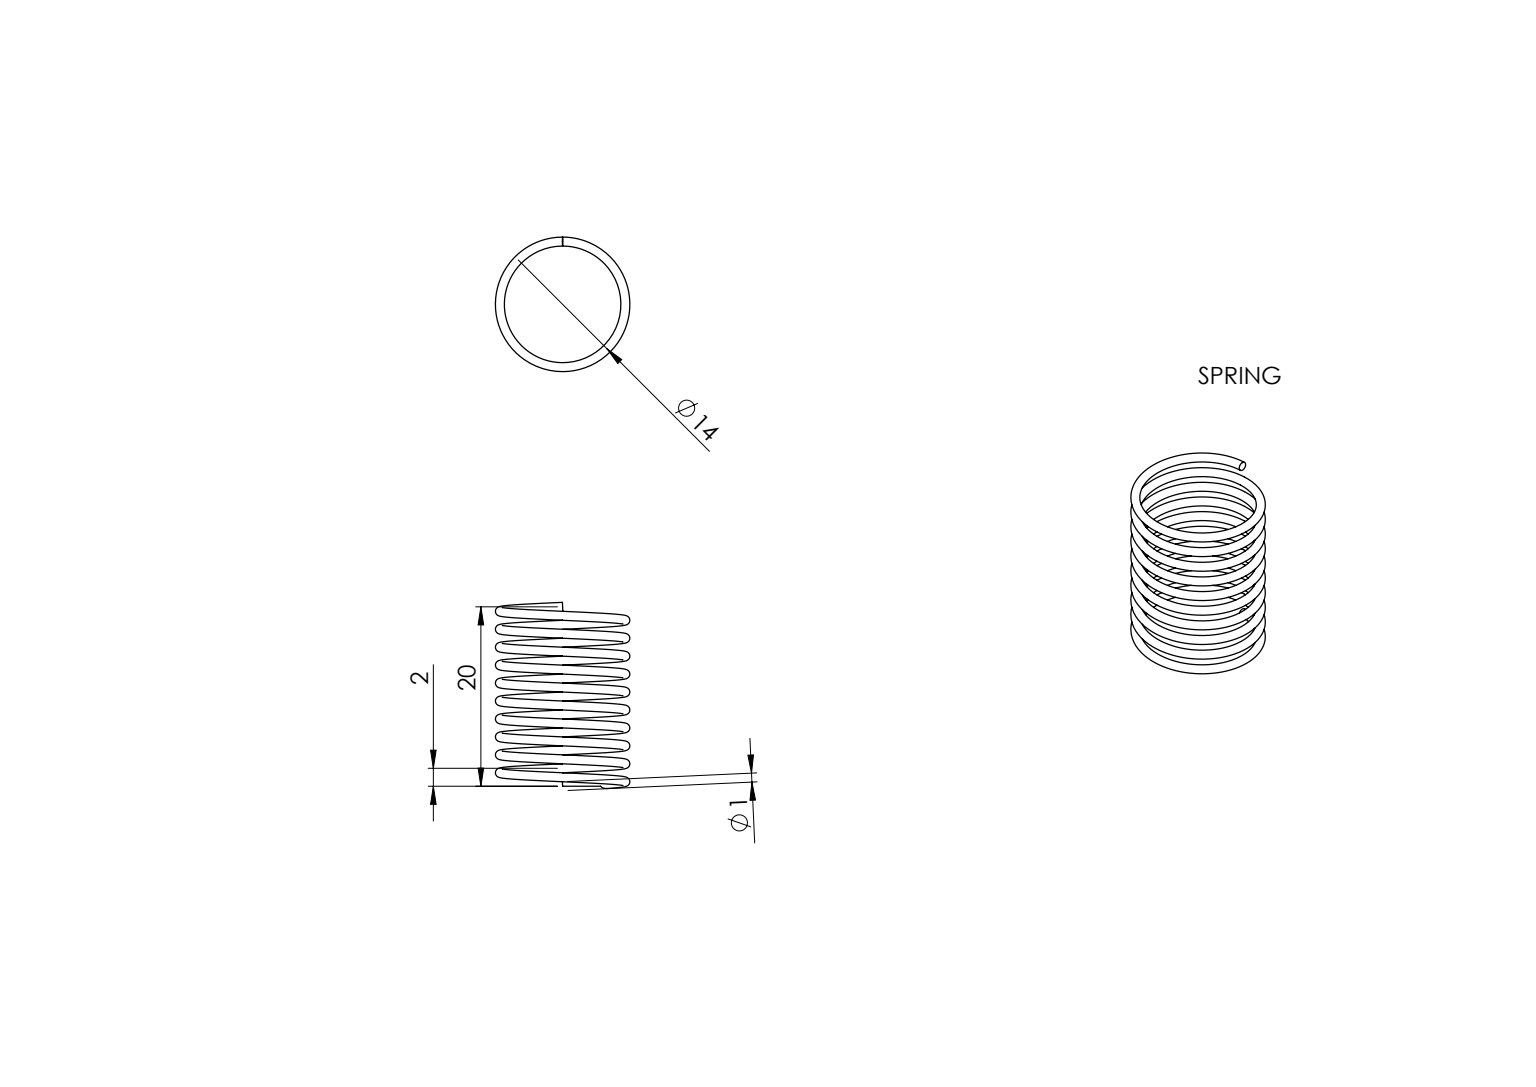
ISO-10303-21;
HEADER;
FILE_DESCRIPTION (('STEP AP214'),
    '1' );
FILE_NAME ('spring.step',
    '2026-10-31T03:44:21',
    ( '' ),
    ( '' ),
    'SwSTEP 2.0',
    'SolidWorks 2026',
    '' );
FILE_SCHEMA (( 'AUTOMOTIVE_DESIGN' ));
ENDSEC;

DATA;
#1=CARTESIAN_POINT ( 'NONE',  ( 55.94051828345054389, 59.20051614449765509, 4.345558710429044957 ) ) ;
#5=CARTESIAN_POINT ( 'NONE',  ( 55.08986747509849380, 53.20051614449766220, 3.727524721679155384 ) ) ;
#7=CARTESIAN_POINT ( 'NONE',  ( 55.11794222512601493, 60.19948385550240744, 3.688883143319541702 ) ) ;
#9=CARTESIAN_POINT ( 'NONE',  ( 44.05948171654949874, 50.79948385550238754, 4.345558710429105354 ) ) ;
#11=CARTESIAN_POINT ( 'NONE',  ( 43.18075615816994173, 53.80051614449766362, 4.924951120819380357 ) ) ;
#23=CARTESIAN_POINT ( 'NONE',  ( 50.02271294988512551, 62.49948385550240459, 7.000000000000000888 ) ) ;
#29=CARTESIAN_POINT ( 'NONE',  ( 47.74827507625478518, 56.59948385550238470, 7.007379884777227730 ) ) ;
#32=CARTESIAN_POINT ( 'NONE',  ( 54.68390685589033495, 51.69948385550241454, -6.485486291978119766 ) ) ;
#34=CARTESIAN_POINT ( 'NONE',  ( 56.65037692655921120, 57.10051614449766078, 2.184720259617097593 ) ) ;
#39=AXIS2_PLACEMENT_3D ( 'NONE', #18626, #14180, #9573 ) ;
#51=CARTESIAN_POINT ( 'NONE',  ( 44.28664221472220675, 59.09948385550240602, -1.832500667257165317 ) ) ;
#56=CARTESIAN_POINT ( 'NONE',  ( 49.97728705011495265, 51.50051614449765935, 8.000000000000001776 ) ) ;
#57=CARTESIAN_POINT ( 'NONE',  ( 53.54508667620424234, 58.70051614449765509, -4.840751629271188961 ) ) ;
#69=CARTESIAN_POINT ( 'NONE',  ( 44.05948171654949874, 62.79948385550241596, 4.345558710429105354 ) ) ;
#70=DIRECTION ( 'NONE',  ( -0.9989677110047504582, -0.04542589977017007230, 1.386346192018204258E-14 ) ) ;
#77=CARTESIAN_POINT ( 'NONE',  ( 58.41169779390614281, 45.99948385550240459, -0.02388180880523160798 ) ) ;
#80=CARTESIAN_POINT ( 'NONE',  ( 50.02271294988512551, 56.49948385550240459, 7.000000000000000888 ) ) ;
#84=CARTESIAN_POINT ( 'NONE',  ( 43.34962307344078880, 54.10051614449766788, -2.184720259617096705 ) ) ;
#92=CARTESIAN_POINT ( 'NONE',  ( 43.20883090819745576, 64.79948385550240175, 4.963592699179006473 ) ) ;
#97=CARTESIAN_POINT ( 'NONE',  ( 42.63976443033212149, 62.00051614449765225, -0.02388180880514948964 ) ) ;
#103=CARTESIAN_POINT ( 'NONE',  ( 55.11794222512599362, 56.80051614449764941, -3.688883143319583446 ) ) ;
#106=CARTESIAN_POINT ( 'NONE',  ( 49.97728705011488870, 55.49948385550241170, -6.000000000000000888 ) ) ;
#108=CARTESIAN_POINT ( 'NONE',  ( 43.20883090819742023, 54.20051614449766220, -4.963592699178938972 ) ) ;
#119=CARTESIAN_POINT ( 'NONE',  ( 43.33558569842703179, 65.09948385550239891, -2.141517661632099223 ) ) ;
#123=CARTESIAN_POINT ( 'NONE',  ( 44.03140696652192787, 61.19948385550239323, -4.306917132069425058 ) ) ;
#125=CARTESIAN_POINT ( 'NONE',  ( 43.18075615816989199, 53.19948385550240744, -4.924951120819313743 ) ) ;
#127=CARTESIAN_POINT ( 'NONE',  ( 45.90387839640208512, 54.30051614449765651, -5.676469297603124353 ) ) ;
#136=CARTESIAN_POINT ( 'NONE',  ( 55.96859303347804371, 62.19948385550240744, 4.306917132069425946 ) ) ;
#137=PLANE ( 'NONE',  #4619 ) ;
#141=CARTESIAN_POINT ( 'NONE',  ( 51.97223112728254790, 58.39948385550241028, 5.992620115222778487 ) ) ;
#144=CARTESIAN_POINT ( 'NONE',  ( 45.31609314410960820, 54.30051614449765651, -6.485486291978072693 ) ) ;
#146=CARTESIAN_POINT ( 'NONE',  ( 48.07319477248762496, 54.40051614449765793, -6.007379884777208190 ) ) ;
#155=CARTESIAN_POINT ( 'NONE',  ( 54.09612160359786515, 63.69948385550240744, -5.676469297603166098 ) ) ;
#165=CARTESIAN_POINT ( 'NONE',  ( 47.37792948025162332, 47.39948385550241028, -7.992620115222770494 ) ) ;
#169=CARTESIAN_POINT ( 'NONE',  ( 55.94051828345050836, 55.79948385550238044, -4.345558710429104465 ) ) ;
#172=CARTESIAN_POINT ( 'NONE',  ( 56.66441430157294690, 56.90051614449766504, -2.141517661632166281 ) ) ;
#185=CARTESIAN_POINT ( 'NONE',  ( 57.61547081786812896, 64.09948385550239891, 2.450534656007040901 ) ) ;
#190=CARTESIAN_POINT ( 'NONE',  ( 44.05948171654945611, 58.20051614449764799, -4.345558710429044069 ) ) ;
#196=CARTESIAN_POINT ( 'NONE',  ( 50.02271294988506156, 56.50051614449767357, -6.000000000000000888 ) ) ;
#200=CARTESIAN_POINT ( 'NONE',  ( 46.49166364869460466, 56.69948385550240744, 4.867452303228209765 ) ) ;
#202=CARTESIAN_POINT ( 'NONE',  ( 47.37792948025170858, 53.60051614449765367, 7.992620115222797139 ) ) ;
#212=CARTESIAN_POINT ( 'NONE',  ( 55.96859303347805081, 62.19948385550241454, 4.306917132069425058 ) ) ;
#216=CARTESIAN_POINT ( 'NONE',  ( 56.65037692655918988, 57.89948385550240317, -2.184720259617163762 ) ) ;
#219=CARTESIAN_POINT ( 'NONE',  ( 52.57664461997811856, 55.59948385550240602, -8.007379884777229506 ) ) ;
#221=CARTESIAN_POINT ( 'NONE',  ( 47.74827507625469281, 54.40051614449766504, -7.007379884777203749 ) ) ;
#229=CARTESIAN_POINT ( 'NONE',  ( 57.36023556966787851, 49.00051614449764514, 0.02388180880515038476 ) ) ;
#230=CARTESIAN_POINT ( 'NONE',  ( 50.02271294988512551, 62.49948385550240459, 7.000000000000000888 ) ) ;
#235=CARTESIAN_POINT ( 'NONE',  ( 44.91013252490152752, 56.79948385550240175, 3.727524721679198461 ) ) ;
#239=CARTESIAN_POINT ( 'NONE',  ( 49.97728705011495265, 55.50051614449766646, 8.000000000000001776 ) ) ;
#240=CARTESIAN_POINT ( 'NONE',  ( 53.50833635130544508, 57.30051614449767072, 4.867452303228181343 ) ) ;
#254=CARTESIAN_POINT ( 'NONE',  ( 55.94051828345050836, 51.79948385550240175, -4.345558710429103577 ) ) ;
#259=CARTESIAN_POINT ( 'NONE',  ( 56.81924384183011512, 48.19948385550240744, 4.924951120819313743 ) ) ;
#261=CARTESIAN_POINT ( 'NONE',  ( 52.25172492374522903, 57.59948385550241312, -7.007379884777225953 ) ) ;
#263=( GEOMETRIC_REPRESENTATION_CONTEXT ( 3 ) GLOBAL_UNCERTAINTY_ASSIGNED_CONTEXT ( ( #6357 ) ) GLOBAL_UNIT_ASSIGNED_CONTEXT ( ( #5384, #15479, #3919 ) ) REPRESENTATION_CONTEXT ( 'NONE', 'WORKASPACE' ) );
#264=CARTESIAN_POINT ( 'NONE',  ( 54.09612160359792199, 57.30051614449765651, 5.676469297603124353 ) ) ;
#276=CARTESIAN_POINT ( 'NONE',  ( 55.94051828345050836, 45.79948385550240886, -4.345558710429104465 ) ) ;
#283=CARTESIAN_POINT ( 'NONE',  ( 43.33558569842706021, 59.90051614449766504, 2.141517661632167169 ) ) ;
#290=CARTESIAN_POINT ( 'NONE',  ( 44.30067958973594955, 54.10051614449766078, -1.875703265242155693 ) ) ;
#296=CARTESIAN_POINT ( 'NONE',  ( 48.02776887271745210, 61.39948385550240317, -5.992620115222778487 ) ) ;
#299=CARTESIAN_POINT ( 'NONE',  ( 47.37792948025170858, 55.60051614449765367, 7.992620115222797139 ) ) ;
#321=CARTESIAN_POINT ( 'NONE',  ( 49.97728705011488159, 55.49948385550240459, -7.000000000000000888 ) ) ;
#323=CARTESIAN_POINT ( 'NONE',  ( 47.37792948025162332, 57.39948385550241028, -7.992620115222770494 ) ) ;
#324=CARTESIAN_POINT ( 'NONE',  ( 47.74827507625469281, 52.40051614449763662, -7.007379884777203749 ) ) ;
#334=CARTESIAN_POINT ( 'NONE',  ( 54.13287192849676188, 64.29948385550241596, 5.649768623646098220 ) ) ;
#341=CARTESIAN_POINT ( 'NONE',  ( 46.49166364869460466, 60.69948385550240033, 4.867452303228209765 ) ) ;
#345=CARTESIAN_POINT ( 'NONE',  ( 43.18075615816994173, 57.80051614449766362, 4.924951120819380357 ) ) ;
#346=CARTESIAN_POINT ( 'NONE',  ( 49.97728705011494554, 57.50051614449766646, 6.000000000000000888 ) ) ;
#360=CARTESIAN_POINT ( 'NONE',  ( 52.25172492374522903, 49.59948385550240602, -7.007379884777227730 ) ) ;
#366=CARTESIAN_POINT ( 'NONE',  ( 54.72065718078924590, 46.29948385550240886, 6.458785618021043895 ) ) ;
#370=CARTESIAN_POINT ( 'NONE',  ( 56.66441430157296821, 64.09948385550239891, 2.141517661632100111 ) ) ;
#373=CARTESIAN_POINT ( 'NONE',  ( 47.74827507625469281, 56.40051614449766504, -7.007379884777203749 ) ) ;
#375=CARTESIAN_POINT ( 'NONE',  ( 52.25172492374522903, 53.59948385550241312, -7.007379884777225953 ) ) ;
#381=CARTESIAN_POINT ( 'NONE',  ( 56.66441430157296821, 54.09948385550240602, 2.141517661632100111 ) ) ;
#387=CARTESIAN_POINT ( 'NONE',  ( 47.70284917648459810, 59.60051614449765367, 6.992620115222797139 ) ) ;
#391=CARTESIAN_POINT ( 'NONE',  ( 46.45491332379576477, 55.70051614449766220, 4.840751629271188961 ) ) ;
#394=CARTESIAN_POINT ( 'NONE',  ( 53.50833635130540955, 61.69948385550240744, -4.867452303228209765 ) ) ;
#396=CARTESIAN_POINT ( 'NONE',  ( 47.37792948025170858, 57.60051614449765367, 7.992620115222797139 ) ) ;
#407=CARTESIAN_POINT ( 'NONE',  ( 47.70284917648453415, 65.39948385550239607, -6.992620115222774047 ) ) ;
#413=CARTESIAN_POINT ( 'NONE',  ( 56.66441430157296821, 62.09948385550239891, 2.141517661632100111 ) ) ;
#415=CARTESIAN_POINT ( 'NONE',  ( 54.72065718078924590, 62.29948385550241596, 6.458785618021043895 ) ) ;
#416=CARTESIAN_POINT ( 'NONE',  ( 57.36023556966787851, 63.00051614449767357, 0.02388180880515038476 ) ) ;
#425=CARTESIAN_POINT ( 'NONE',  ( 44.03140696652198471, 45.80051614449766362, 4.306917132069485454 ) ) ;
#426=CARTESIAN_POINT ( 'NONE',  ( 55.96859303347804371, 64.19948385550239323, 4.306917132069425946 ) ) ;
#431=CARTESIAN_POINT ( 'NONE',  ( 43.69122665457040000, 64.99948385550240459, 0.02388180880521036456 ) ) ;
#433=CARTESIAN_POINT ( 'NONE',  ( 42.38452918213190657, 61.90051614449766504, 2.450534656007115508 ) ) ;
#434=CARTESIAN_POINT ( 'NONE',  ( 44.88205777487401349, 57.80051614449766362, 3.688883143319584779 ) ) ;
#446=CARTESIAN_POINT ( 'NONE',  ( 43.34962307344081012, 54.89948385550240317, 2.184720259617164650 ) ) ;
#451=CARTESIAN_POINT ( 'NONE',  ( 47.42335538002188144, 52.59948385550240602, 8.007379884777233059 ) ) ;
#454=CARTESIAN_POINT ( 'NONE',  ( 56.66441430157296821, 62.09948385550239891, 2.141517661632100111 ) ) ;
#456=CARTESIAN_POINT ( 'NONE',  ( 47.70284917648459100, 63.60051614449766078, 6.992620115222796251 ) ) ;
#458=CARTESIAN_POINT ( 'NONE',  ( 49.97728705011488159, 57.49948385550241170, -7.000000000000000888 ) ) ;
#466=CARTESIAN_POINT ( 'NONE',  ( 54.13287192849676188, 52.29948385550240886, 5.649768623646098220 ) ) ;
#472=CARTESIAN_POINT ( 'NONE',  ( 42.63976443033212149, 64.00051614449765225, -0.02388180880514948964 ) ) ;
#478=CARTESIAN_POINT ( 'NONE',  ( 55.71335778527780036, 58.90051614449766504, -1.832500667257213056 ) ) ;
#483=CARTESIAN_POINT ( 'NONE',  ( 52.57664461997821093, 57.40051614449767214, 8.007379884777206414 ) ) ;
#493=LINE ( 'NONE', #12738, #1897 ) ;
#496=UNCERTAINTY_MEASURE_WITH_UNIT (LENGTH_MEASURE( 1.000000000000000082E-05 ), #5087, 'distance_accuracy_value', 'NONE');
#501=CARTESIAN_POINT ( 'NONE',  ( 55.94051828345050836, 63.79948385550240886, -4.345558710429104465 ) ) ;
#503=CARTESIAN_POINT ( 'NONE',  ( 42.38452918213188525, 63.09948385550240602, -2.450534656007040013 ) ) ;
#505=CARTESIAN_POINT ( 'NONE',  ( 42.63976443033212860, 58.00051614449765225, -0.02388180880514948964 ) ) ;
#511=CARTESIAN_POINT ( 'NONE',  ( 45.86712807150323812, 63.29948385550240886, -5.649768623646098220 ) ) ;
#518=CARTESIAN_POINT ( 'NONE',  ( 51.97223112728254790, 62.39948385550240317, 5.992620115222778487 ) ) ;
#521=CARTESIAN_POINT ( 'NONE',  ( 41.58830220609386430, 62.00051614449766646, -0.02388180880514929535 ) ) ;
#523=CARTESIAN_POINT ( 'NONE',  ( 44.88205777487401349, 61.80051614449766362, 3.688883143319584779 ) ) ;
#539=CARTESIAN_POINT ( 'NONE',  ( 54.13287192849676188, 52.29948385550240886, 5.649768623646098220 ) ) ;
#544=AXIS2_PLACEMENT_3D ( 'NONE', #1693, #7660, #14721 ) ;
#545=CARTESIAN_POINT ( 'NONE',  ( 58.41169779390614281, 49.99948385550240459, -0.02388180880523160798 ) ) ;
#548=CARTESIAN_POINT ( 'NONE',  ( 52.29715082351547295, 64.39948385550239607, 6.992620115222774047 ) ) ;
#552=CARTESIAN_POINT ( 'NONE',  ( 44.05948171654945611, 60.20051614449764799, -4.345558710429044069 ) ) ;
#554=CARTESIAN_POINT ( 'NONE',  ( 50.02271294988512551, 60.49948385550240459, 7.000000000000000888 ) ) ;
#561=CARTESIAN_POINT ( 'NONE',  ( 56.65037692655918988, 51.89948385550241028, -2.184720259617163762 ) ) ;
#570=CARTESIAN_POINT ( 'NONE',  ( 45.86712807150323812, 47.29948385550240886, -5.649768623646098220 ) ) ;
#572=CARTESIAN_POINT ( 'NONE',  ( 46.49166364869456913, 62.30051614449766362, -4.867452303228181343 ) ) ;
#578=CARTESIAN_POINT ( 'NONE',  ( 52.57664461997821093, 61.40051614449765793, 8.007379884777206414 ) ) ;
#596=CARTESIAN_POINT ( 'NONE',  ( 55.08986747509847248, 45.79948385550240886, -3.727524721679197572 ) ) ;
#598=CARTESIAN_POINT ( 'NONE',  ( 41.58830220609386430, 58.99948385550239749, 0.02388180880523263147 ) ) ;
#600=CARTESIAN_POINT ( 'NONE',  ( 47.74827507625469281, 62.40051614449766504, -7.007379884777203749 ) ) ;
#609=CARTESIAN_POINT ( 'NONE',  ( 42.63976443033212149, 48.00051614449766646, -0.02388180880514948964 ) ) ;
#616=CARTESIAN_POINT ( 'NONE',  ( 43.69122665457040000, 60.99948385550241170, 0.02388180880521036456 ) ) ;
#618=CARTESIAN_POINT ( 'NONE',  ( 54.09612160359786515, 47.69948385550240744, -5.676469297603166098 ) ) ;
#621=CARTESIAN_POINT ( 'NONE',  ( 56.81924384183006538, 56.80051614449764941, -4.924951120819380357 ) ) ;
#622=CARTESIAN_POINT ( 'NONE',  ( 44.88205777487401349, 59.80051614449766362, 3.688883143319584779 ) ) ;
#626=ORIENTED_EDGE ( 'NONE', *, *, #1141, .T. ) ;
#636=CARTESIAN_POINT ( 'NONE',  ( 57.36023556966787851, 53.99948385550239749, -0.02388180880522424582 ) ) ;
#641=CARTESIAN_POINT ( 'NONE',  ( 56.79116909180255135, 49.79948385550240175, -4.963592699179005585 ) ) ;
#645=CARTESIAN_POINT ( 'NONE',  ( 44.88205777487398507, 47.19948385550240744, -3.688883143319540814 ) ) ;
#650=CARTESIAN_POINT ( 'NONE',  ( 43.33558569842706021, 57.90051614449766504, 2.141517661632167169 ) ) ;
#654=CARTESIAN_POINT ( 'NONE',  ( 57.36023556966787851, 55.99948385550239038, -0.02388180880522424582 ) ) ;
#663=CARTESIAN_POINT ( 'NONE',  ( 56.65037692655918988, 53.89948385550240317, -2.184720259617163762 ) ) ;
#672=CARTESIAN_POINT ( 'NONE',  ( 43.34962307344078880, 64.10051614449766078, -2.184720259617096705 ) ) ;
#676=CARTESIAN_POINT ( 'NONE',  ( 46.45491332379576477, 61.70051614449766220, 4.840751629271188961 ) ) ;
#682=CARTESIAN_POINT ( 'NONE',  ( 49.97728705011495265, 59.50051614449765935, 8.000000000000001776 ) ) ;
#700=CARTESIAN_POINT ( 'NONE',  ( 46.49166364869460466, 46.69948385550240744, 4.867452303228209765 ) ) ;
#702=CARTESIAN_POINT ( 'NONE',  ( 42.39856655714566358, 60.89948385550241028, 2.493737253992119207 ) ) ;
#703=CARTESIAN_POINT ( 'NONE',  ( 45.86712807150329496, 63.70051614449766220, 5.649768623646139964 ) ) ;
#712=CARTESIAN_POINT ( 'NONE',  ( 44.03140696652198471, 53.80051614449766362, 4.306917132069485454 ) ) ;
#722=CARTESIAN_POINT ( 'NONE',  ( 47.42335538002180328, 58.40051614449765793, -8.007379884777206414 ) ) ;
#723=CARTESIAN_POINT ( 'NONE',  ( 44.30067958973594955, 62.10051614449765367, -1.875703265242155693 ) ) ;
#734=CARTESIAN_POINT ( 'NONE',  ( 43.34962307344081012, 60.89948385550241028, 2.184720259617164650 ) ) ;
#738=CARTESIAN_POINT ( 'NONE',  ( 47.42335538002188144, 54.59948385550240602, 8.007379884777233059 ) ) ;
#740=CARTESIAN_POINT ( 'NONE',  ( 44.03140696652192787, 65.19948385550240744, -4.306917132069425058 ) ) ;
#743=CARTESIAN_POINT ( 'NONE',  ( 56.65037692655921120, 61.10051614449766078, 2.184720259617097593 ) ) ;
#744=CARTESIAN_POINT ( 'NONE',  ( 44.28664221472220675, 65.09948385550239891, -1.832500667257165317 ) ) ;
#745=CARTESIAN_POINT ( 'NONE',  ( 43.34962307344081012, 58.89948385550241028, 2.184720259617164650 ) ) ;
#754=CARTESIAN_POINT ( 'NONE',  ( 45.90387839640214196, 58.69948385550240033, 5.676469297603166098 ) ) ;
#764=CARTESIAN_POINT ( 'NONE',  ( 55.96859303347804371, 46.19948385550238612, 4.306917132069425946 ) ) ;
#767=CARTESIAN_POINT ( 'NONE',  ( 53.54508667620424234, 58.70051614449765509, -4.840751629271188961 ) ) ;
#780=ADVANCED_BREP_SHAPE_REPRESENTATION ( '', ( #2030, #10359 ), #6832 ) ;
#796=CARTESIAN_POINT ( 'NONE',  ( 54.13287192849676188, 64.29948385550241596, 5.649768623646098220 ) ) ;
#798=CARTESIAN_POINT ( 'NONE',  ( 57.60143344285433642, 63.89948385550240317, -2.493737253992118319 ) ) ;
#799=CARTESIAN_POINT ( 'NONE',  ( 52.29715082351538769, 62.60051614449766078, -6.992620115222796251 ) ) ;
#806=CARTESIAN_POINT ( 'NONE',  ( 55.94051828345054389, 55.20051614449766220, 4.345558710429044957 ) ) ;
#815=CARTESIAN_POINT ( 'NONE',  ( 47.74827507625478518, 48.59948385550239180, 7.007379884777227730 ) ) ;
#817=CARTESIAN_POINT ( 'NONE',  ( 49.97728705011486738, 47.49948385550240459, -8.000000000000001776 ) ) ;
#820=CARTESIAN_POINT ( 'NONE',  ( 55.69932041026405045, 61.10051614449766788, 1.875703265242156359 ) ) ;
#830=EDGE_LOOP ( 'NONE', ( #4840, #13776, #3319, #7867, #626, #1665 ) ) ;
#832=CARTESIAN_POINT ( 'NONE',  ( 56.65037692655918988, 57.89948385550240317, -2.184720259617163762 ) ) ;
#836=CARTESIAN_POINT ( 'NONE',  ( 45.27934281921075410, 55.29948385550240175, -6.458785618021043895 ) ) ;
#838=CARTESIAN_POINT ( 'NONE',  ( 51.92680522751233951, 51.59948385550240602, -6.007379884777223289 ) ) ;
#841=CARTESIAN_POINT ( 'NONE',  ( 44.03140696652198471, 61.80051614449767072, 4.306917132069485454 ) ) ;
#842=CARTESIAN_POINT ( 'NONE',  ( 49.97728705011488870, 65.49948385550240459, -6.000000000000000888 ) ) ;
#844=CARTESIAN_POINT ( 'NONE',  ( 56.66441430157296821, 60.09948385550240602, 2.141517661632100111 ) ) ;
#852=CARTESIAN_POINT ( 'NONE',  ( 43.33558569842703179, 61.09948385550240602, -2.141517661632099223 ) ) ;
#863=CARTESIAN_POINT ( 'NONE',  ( 46.45491332379576477, 59.70051614449766220, 4.840751629271188961 ) ) ;
#888=CARTESIAN_POINT ( 'NONE',  ( 44.88205777487398507, 51.19948385550240744, -3.688883143319540814 ) ) ;
#890=CARTESIAN_POINT ( 'NONE',  ( 44.03140696652192787, 47.19948385550240744, -4.306917132069425058 ) ) ;
#891=CARTESIAN_POINT ( 'NONE',  ( 41.58830220609386430, 46.00051614449764514, -0.02388180880514929535 ) ) ;
#902=CARTESIAN_POINT ( 'NONE',  ( 43.34962307344078880, 52.10051614449766078, -2.184720259617096705 ) ) ;
#913=CARTESIAN_POINT ( 'NONE',  ( 44.03140696652192787, 49.19948385550240033, -4.306917132069425058 ) ) ;
#915=CARTESIAN_POINT ( 'NONE',  ( 56.81924384183011512, 50.19948385550241454, 4.924951120819313743 ) ) ;
#917=CARTESIAN_POINT ( 'NONE',  ( 49.97728705011494554, 59.50051614449765935, 6.000000000000000888 ) ) ;
#919=PLANE ( 'NONE',  #15371 ) ;
#931=CARTESIAN_POINT ( 'NONE',  ( 55.94051828345050836, 55.79948385550239465, -4.345558710429103577 ) ) ;
#937=CARTESIAN_POINT ( 'NONE',  ( 54.72065718078924590, 60.29948385550240175, 6.458785618021043895 ) ) ;
#939=CARTESIAN_POINT ( 'NONE',  ( 55.08986747509847248, 49.79948385550240175, -3.727524721679197572 ) ) ;
#943=CARTESIAN_POINT ( 'NONE',  ( 57.61547081786810764, 46.90051614449766504, -2.450534656007114176 ) ) ;
#945=CARTESIAN_POINT ( 'NONE',  ( 55.71335778527780036, 44.90051614449765793, -1.832500667257213056 ) ) ;
#954=CARTESIAN_POINT ( 'NONE',  ( 54.13287192849676188, 60.29948385550240886, 5.649768623646098220 ) ) ;
#966=CARTESIAN_POINT ( 'NONE',  ( 56.66441430157296821, 54.09948385550240602, 2.141517661632100111 ) ) ;
#968=CARTESIAN_POINT ( 'NONE',  ( 44.05948171654945611, 46.20051614449766930, -4.345558710429044069 ) ) ;
#991=CARTESIAN_POINT ( 'NONE',  ( 50.02271294988506156, 44.50051614449765935, -6.000000000000000888 ) ) ;
#995=CARTESIAN_POINT ( 'NONE',  ( 44.91013252490152752, 52.79948385550240175, 3.727524721679198461 ) ) ;
#997=CARTESIAN_POINT ( 'NONE',  ( 43.18075615816989199, 63.19948385550240744, -4.924951120819313743 ) ) ;
#998=CARTESIAN_POINT ( 'NONE',  ( 56.81924384183006538, 48.80051614449767072, -4.924951120819380357 ) ) ;
#1009=CARTESIAN_POINT ( 'NONE',  ( 50.02271294988505446, 54.50051614449765935, -7.000000000000000888 ) ) ;
#1018=CARTESIAN_POINT ( 'NONE',  ( 57.36023556966787851, 49.99948385550238328, -0.02388180880522424582 ) ) ;
#1020=CARTESIAN_POINT ( 'NONE',  ( 49.97728705011495265, 63.50051614449765935, 8.000000000000001776 ) ) ;
#1022=CARTESIAN_POINT ( 'NONE',  ( 47.74827507625469281, 48.40051614449764372, -7.007379884777203749 ) ) ;
#1035=CARTESIAN_POINT ( 'NONE',  ( 44.03140696652193498, 57.19948385550239323, -4.306917132069424170 ) ) ;
#1040=CARTESIAN_POINT ( 'NONE',  ( 47.37792948025162332, 59.39948385550240317, -7.992620115222770494 ) ) ;
#1042=CARTESIAN_POINT ( 'NONE',  ( 49.97728705011488870, 51.49948385550240459, -6.000000000000000888 ) ) ;
#1045=CARTESIAN_POINT ( 'NONE',  ( 56.81924384183006538, 44.80051614449766362, -4.924951120819380357 ) ) ;
#1046=CARTESIAN_POINT ( 'NONE',  ( 43.69122665457040000, 48.00051614449766646, -0.02388180880515696977 ) ) ;
#1053=CARTESIAN_POINT ( 'NONE',  ( 42.63976443033212860, 56.99948385550241170, 0.02388180880522514787 ) ) ;
#1061=CARTESIAN_POINT ( 'NONE',  ( 56.65037692655918988, 49.89948385550240317, -2.184720259617163762 ) ) ;
#1063=CARTESIAN_POINT ( 'NONE',  ( 57.36023556966787851, 47.00051614449764514, 0.02388180880515038476 ) ) ;
#1085=CARTESIAN_POINT ( 'NONE',  ( 44.91013252490150620, 48.20051614449766930, -3.727524721679154940 ) ) ;
#1089=CARTESIAN_POINT ( 'NONE',  ( 43.69122665457040000, 52.99948385550241170, 0.02388180880521036456 ) ) ;
#1091=CARTESIAN_POINT ( 'NONE',  ( 56.66441430157296821, 46.09948385550240602, 2.141517661632100111 ) ) ;
#1092=CARTESIAN_POINT ( 'NONE',  ( 41.58830220609386430, 48.00051614449766646, -0.02388180880514929535 ) ) ;
#1100=CARTESIAN_POINT ( 'NONE',  ( 49.97728705011495265, 51.50051614449765935, 7.000000000000000888 ) ) ;
#1108=CARTESIAN_POINT ( 'NONE',  ( 55.94051828345050836, 51.79948385550240175, -4.345558710429104465 ) ) ;
#1110=CARTESIAN_POINT ( 'NONE',  ( 45.31609314410967926, 46.69948385550240744, 6.485486291978119766 ) ) ;
#1112=CARTESIAN_POINT ( 'NONE',  ( 45.90387839640208512, 46.30051614449766362, -5.676469297603124353 ) ) ;
#1127=CARTESIAN_POINT ( 'NONE',  ( 57.61547081786812896, 58.09948385550241312, 2.450534656007040901 ) ) ;
#1131=CARTESIAN_POINT ( 'NONE',  ( 55.71335778527780747, 48.09948385550240602, 1.832500667257165983 ) ) ;
#1135=CARTESIAN_POINT ( 'NONE',  ( 43.20883090819742023, 50.20051614449766220, -4.963592699178938972 ) ) ;
#1136=CARTESIAN_POINT ( 'NONE',  ( 48.07319477248762496, 50.40051614449766504, -6.007379884777208190 ) ) ;
#1141=EDGE_CURVE ( 'NONE', #2212, #18471, #2132, .T. ) ;
#1146=CARTESIAN_POINT ( 'NONE',  ( 43.34962307344081012, 60.89948385550241028, 2.184720259617164650 ) ) ;
#1156=CARTESIAN_POINT ( 'NONE',  ( 57.36023556966787851, 51.99948385550238328, -0.02388180880522424582 ) ) ;
#1160=CARTESIAN_POINT ( 'NONE',  ( 54.13287192849671214, 50.70051614449766220, -5.649768623646139964 ) ) ;
#1183=CARTESIAN_POINT ( 'NONE',  ( 44.88205777487401349, 49.80051614449765651, 3.688883143319584779 ) ) ;
#1187=CARTESIAN_POINT ( 'NONE',  ( 53.54508667620428497, 48.29948385550240175, 4.840751629271157874 ) ) ;
#1190=CARTESIAN_POINT ( 'NONE',  ( 52.62207051974839089, 64.39948385550239607, 7.992620115222770494 ) ) ;
#1191=CARTESIAN_POINT ( 'NONE',  ( 47.74827507625469281, 64.40051614449765793, -7.007379884777203749 ) ) ;
#1205=CARTESIAN_POINT ( 'NONE',  ( 43.34962307344081012, 50.89948385550241028, 2.184720259617164650 ) ) ;
#1207=CARTESIAN_POINT ( 'NONE',  ( 54.72065718078924590, 46.29948385550240886, 6.458785618021043895 ) ) ;
#1209=CARTESIAN_POINT ( 'NONE',  ( 55.96859303347802239, 46.80051614449767072, -4.306917132069484566 ) ) ;
#1225=CARTESIAN_POINT ( 'NONE',  ( 56.79116909180255135, 61.79948385550240175, -4.963592699179005585 ) ) ;
#1228=CARTESIAN_POINT ( 'NONE',  ( 48.02776887271745210, 51.39948385550241028, -5.992620115222778487 ) ) ;
#1232=CARTESIAN_POINT ( 'NONE',  ( 54.72065718078918906, 48.70051614449766930, -6.458785618021089192 ) ) ;
#1233=CARTESIAN_POINT ( 'NONE',  ( 50.02271294988506156, 50.50051614449765935, -6.000000000000000888 ) ) ;
#1243=CARTESIAN_POINT ( 'NONE',  ( 50.02271294988512551, 62.49948385550240459, 7.000000000000000888 ) ) ;
#1258=CARTESIAN_POINT ( 'NONE',  ( 49.97728705011488159, 53.49948385550240459, -7.000000000000000888 ) ) ;
#1260=CARTESIAN_POINT ( 'NONE',  ( 49.97728705011495265, 45.50051614449765935, 7.000000000000000888 ) ) ;
#1283=CARTESIAN_POINT ( 'NONE',  ( 44.30067958973594955, 50.10051614449766078, -1.875703265242155693 ) ) ;
#1287=CARTESIAN_POINT ( 'NONE',  ( 49.97728705011488870, 51.49948385550240459, -6.000000000000000888 ) ) ;
#1291=CARTESIAN_POINT ( 'NONE',  ( 57.36023556966787851, 51.99948385550238328, -0.02388180880522424582 ) ) ;
#1292=CARTESIAN_POINT ( 'NONE',  ( 47.42335538002180328, 46.40051614449765793, -8.007379884777206414 ) ) ;
#1309=CARTESIAN_POINT ( 'NONE',  ( 47.70284917648453415, 49.39948385550238896, -6.992620115222774047 ) ) ;
#1311=CARTESIAN_POINT ( 'NONE',  ( 54.68390685589033495, 53.69948385550240744, -6.485486291978119766 ) ) ;
#1312=CARTESIAN_POINT ( 'NONE',  ( 56.65037692655921120, 49.10051614449766078, 2.184720259617097593 ) ) ;
#1328=CARTESIAN_POINT ( 'NONE',  ( 50.02271294988513972, 58.49948385550241170, 8.000000000000001776 ) ) ;
#1330=CARTESIAN_POINT ( 'NONE',  ( 44.91013252490152752, 58.79948385550240175, 3.727524721679198461 ) ) ;
#1333=CARTESIAN_POINT ( 'NONE',  ( 43.20883090819742023, 46.20051614449766220, -4.963592699178938972 ) ) ;
#1334=CARTESIAN_POINT ( 'NONE',  ( 44.30067958973594955, 52.10051614449766788, -1.875703265242155693 ) ) ;
#1345=CARTESIAN_POINT ( 'NONE',  ( 56.65037692655918988, 47.89948385550240317, -2.184720259617163762 ) ) ;
#1350=CARTESIAN_POINT ( 'NONE',  ( 49.97728705011488159, 55.49948385550240459, -7.000000000000000888 ) ) ;
#1352=CARTESIAN_POINT ( 'NONE',  ( 44.03140696652198471, 49.80051614449766362, 4.306917132069485454 ) ) ;
#1364=CARTESIAN_POINT ( 'NONE',  ( 45.27934281921075410, 63.29948385550240175, -6.458785618021043895 ) ) ;
#1373=CARTESIAN_POINT ( 'NONE',  ( 51.92680522751238925, 49.40051614449766504, 6.007379884777208190 ) ) ;
#1378=CARTESIAN_POINT ( 'NONE',  ( 50.02271294988511841, 54.49948385550240459, 6.000000000000000888 ) ) ;
#1380=CARTESIAN_POINT ( 'NONE',  ( 54.13287192849676188, 50.29948385550240175, 5.649768623646098220 ) ) ;
#1382=CARTESIAN_POINT ( 'NONE',  ( 47.37792948025170858, 51.60051614449766788, 7.992620115222797139 ) ) ;
#1401=CARTESIAN_POINT ( 'NONE',  ( 52.25172492374522903, 57.59948385550241312, -7.007379884777225953 ) ) ;
#1403=CARTESIAN_POINT ( 'NONE',  ( 41.58830220609386430, 50.99948385550241170, 0.02388180880523263147 ) ) ;
#1405=CARTESIAN_POINT ( 'NONE',  ( 42.63976443033212860, 50.00051614449766646, -0.02388180880514948964 ) ) ;
#1414=ORIENTED_EDGE ( 'NONE', *, *, #12268, .T. ) ;
#1425=CARTESIAN_POINT ( 'NONE',  ( 55.11794222512601493, 58.19948385550240744, 3.688883143319541702 ) ) ;
#1428=CARTESIAN_POINT ( 'NONE',  ( 57.60143344285435774, 53.10051614449767499, 2.493737253992045044 ) ) ;
#1430=CARTESIAN_POINT ( 'NONE',  ( 51.97223112728249816, 48.60051614449766788, -5.992620115222793586 ) ) ;
#1442=CARTESIAN_POINT ( 'NONE',  ( 45.90387839640214196, 48.69948385550240744, 5.676469297603166098 ) ) ;
#1446=CARTESIAN_POINT ( 'NONE',  ( 49.97728705011486738, 49.49948385550241170, -8.000000000000001776 ) ) ;
#1448=CARTESIAN_POINT ( 'NONE',  ( 43.34962307344081012, 58.89948385550241028, 2.184720259617164650 ) ) ;
#1451=CARTESIAN_POINT ( 'NONE',  ( 47.74827507625469281, 54.40051614449766504, -7.007379884777203749 ) ) ;
#1458=CARTESIAN_POINT ( 'NONE',  ( 41.58830220609386430, 64.99948385550240459, 0.02388180880523263147 ) ) ;
#1463=CARTESIAN_POINT ( 'NONE',  ( 55.94051828345054389, 61.20051614449765509, 4.345558710429044957 ) ) ;
#1467=UNCERTAINTY_MEASURE_WITH_UNIT (LENGTH_MEASURE( 1.000000000000000082E-05 ), #8121, 'distance_accuracy_value', 'NONE');
#1469=CARTESIAN_POINT ( 'NONE',  ( 53.54508667620424234, 50.70051614449766220, -4.840751629271188961 ) ) ;
#1473=CARTESIAN_POINT ( 'NONE',  ( 44.88205777487398507, 55.19948385550240744, -3.688883143319540814 ) ) ;
#1475=CARTESIAN_POINT ( 'NONE',  ( 50.02271294988512551, 54.49948385550240459, 7.000000000000000888 ) ) ;
#1476=CARTESIAN_POINT ( 'NONE',  ( 52.57664461997821093, 51.40051614449767214, 8.007379884777206414 ) ) ;
#1497=CARTESIAN_POINT ( 'NONE',  ( 45.86712807150323812, 57.29948385550240175, -5.649768623646098220 ) ) ;
#1499=CARTESIAN_POINT ( 'NONE',  ( 47.37792948025162332, 53.39948385550241028, -7.992620115222770494 ) ) ;
#1501=CARTESIAN_POINT ( 'NONE',  ( 44.03140696652198471, 51.80051614449766362, 4.306917132069485454 ) ) ;
#1521=CARTESIAN_POINT ( 'NONE',  ( 55.69932041026404335, 59.89948385550240317, -1.875703265242203432 ) ) ;
#1524=CARTESIAN_POINT ( 'NONE',  ( 45.31609314410960820, 56.30051614449766362, -6.485486291978072693 ) ) ;
#1525=CARTESIAN_POINT ( 'NONE',  ( 48.07319477248762496, 58.40051614449765793, -6.007379884777208190 ) ) ;
#1535=EDGE_CURVE ( 'NONE', #11812, #12707, #10245, .T. ) ;
#1538=CARTESIAN_POINT ( 'NONE',  ( 43.34962307344081012, 48.89948385550240317, 2.184720259617164650 ) ) ;
#1544=CARTESIAN_POINT ( 'NONE',  ( 49.97728705011486738, 45.49948385550240459, -8.000000000000001776 ) ) ;
#1546=CARTESIAN_POINT ( 'NONE',  ( 43.34962307344081012, 60.89948385550241028, 2.184720259617164650 ) ) ;
#1549=CARTESIAN_POINT ( 'NONE',  ( 49.97728705011495265, 51.50051614449765935, 7.000000000000000888 ) ) ;
#1563=CARTESIAN_POINT ( 'NONE',  ( 52.29715082351547295, 46.39948385550240317, 6.992620115222774047 ) ) ;
#1570=CARTESIAN_POINT ( 'NONE',  ( 55.96859303347802239, 58.80051614449765651, -4.306917132069484566 ) ) ;
#1574=CARTESIAN_POINT ( 'NONE',  ( 53.50833635130544508, 55.30051614449765651, 4.867452303228181343 ) ) ;
#1577=CARTESIAN_POINT ( 'NONE',  ( 55.08986747509847248, 55.79948385550239465, -3.727524721679197572 ) ) ;
#1580=CARTESIAN_POINT ( 'NONE',  ( 56.81924384183006538, 50.80051614449766362, -4.924951120819380357 ) ) ;
#1593=CARTESIAN_POINT ( 'NONE',  ( 54.13287192849676188, 62.29948385550240886, 5.649768623646098220 ) ) ;
#1598=CARTESIAN_POINT ( 'NONE',  ( 55.96859303347804371, 60.19948385550240744, 4.306917132069425946 ) ) ;
#1601=CARTESIAN_POINT ( 'NONE',  ( 56.81924384183011512, 56.19948385550240744, 4.924951120819313743 ) ) ;
#1604=CARTESIAN_POINT ( 'NONE',  ( 56.66441430157294690, 52.90051614449765793, -2.141517661632166281 ) ) ;
#1619=CARTESIAN_POINT ( 'NONE',  ( 49.97728705011488159, 65.49948385550240459, -7.000000000000000888 ) ) ;
#1625=CARTESIAN_POINT ( 'NONE',  ( 49.97728705011488870, 57.49948385550241170, -6.000000000000000888 ) ) ;
#1629=CARTESIAN_POINT ( 'NONE',  ( 50.02271294988505446, 52.50051614449766646, -8.000000000000001776 ) ) ;
#1631=CARTESIAN_POINT ( 'NONE',  ( 46.45491332379576477, 53.70051614449766220, 4.840751629271188961 ) ) ;
#1638=CARTESIAN_POINT ( 'NONE',  ( 54.31203442848995877, 44.90264883920728778, -4.999999999999999112 ) ) ;
#1650=CARTESIAN_POINT ( 'NONE',  ( 43.20883090819745576, 48.79948385550240175, 4.963592699179006473 ) ) ;
#1652=CARTESIAN_POINT ( 'NONE',  ( 47.70284917648453415, 55.39948385550238896, -6.992620115222774047 ) ) ;
#1655=CARTESIAN_POINT ( 'NONE',  ( 52.25172492374527877, 55.40051614449764372, 7.007379884777203749 ) ) ;
#1664=CARTESIAN_POINT ( 'NONE',  ( 47.70284917648453415, 47.39948385550238896, -6.992620115222774047 ) ) ;
#1665=ORIENTED_EDGE ( 'NONE', *, *, #2942, .F. ) ;
#1668=CARTESIAN_POINT ( 'NONE',  ( 50.02271294988505446, 62.50051614449766646, -7.000000000000000888 ) ) ;
#1675=CARTESIAN_POINT ( 'NONE',  ( 48.07319477248762496, 52.40051614449767214, -6.007379884777208190 ) ) ;
#1679=CARTESIAN_POINT ( 'NONE',  ( 44.28664221472220675, 59.09948385550240602, -1.832500667257165317 ) ) ;
#1681=CARTESIAN_POINT ( 'NONE',  ( 49.97728705011495265, 51.50051614449765935, 8.000000000000001776 ) ) ;
#1690=CARTESIAN_POINT ( 'NONE',  ( 54.09612160359786515, 61.69948385550240744, -5.676469297603166098 ) ) ;
#1693=CARTESIAN_POINT ( 'NONE',  ( 49.99999999999997158, 65.00000000000002842, -7.000000000000000888 ) ) ;
#1694=CARTESIAN_POINT ( 'NONE',  ( 56.66441430157296821, 60.09948385550240602, 2.141517661632100111 ) ) ;
#1696=CARTESIAN_POINT ( 'NONE',  ( 45.31609314410967926, 52.69948385550240744, 6.485486291978119766 ) ) ;
#1698=CARTESIAN_POINT ( 'NONE',  ( 43.34962307344078880, 52.10051614449766078, -2.184720259617096705 ) ) ;
#1708=CARTESIAN_POINT ( 'NONE',  ( 49.97728705011488159, 63.49948385550241170, -7.000000000000000888 ) ) ;
#1713=CARTESIAN_POINT ( 'NONE',  ( 44.28664221472220675, 55.09948385550241312, -1.832500667257165317 ) ) ;
#1716=CARTESIAN_POINT ( 'NONE',  ( 58.41169779390614281, 55.00051614449766646, 0.02388180880515032231 ) ) ;
#1717=CARTESIAN_POINT ( 'NONE',  ( 53.50833635130544508, 53.30051614449767072, 4.867452303228181343 ) ) ;
#1732=CARTESIAN_POINT ( 'NONE',  ( 44.03140696652193498, 49.19948385550240744, -4.306917132069424170 ) ) ;
#1735=ORIENTED_EDGE ( 'NONE', *, *, #11053, .F. ) ;
#1738=CARTESIAN_POINT ( 'NONE',  ( 47.42335538002188144, 46.59948385550239891, 8.007379884777233059 ) ) ;
#1742=CARTESIAN_POINT ( 'NONE',  ( 52.29715082351547295, 58.39948385550238896, 6.992620115222774047 ) ) ;
#1745=CARTESIAN_POINT ( 'NONE',  ( 50.02271294988505446, 52.50051614449765935, -7.000000000000000888 ) ) ;
#1753=CARTESIAN_POINT ( 'NONE',  ( 49.97728705011486738, 65.49948385550240459, -8.000000000000001776 ) ) ;
#1760=CARTESIAN_POINT ( 'NONE',  ( 47.74827507625470702, 60.40051614449766504, -7.007379884777204637 ) ) ;
#1764=CARTESIAN_POINT ( 'NONE',  ( 51.92680522751238925, 57.40051614449767214, 6.007379884777208190 ) ) ;
#1768=CARTESIAN_POINT ( 'NONE',  ( 56.30877334542961421, 55.99948385550241170, -0.02388180880520959434 ) ) ;
#1770=CARTESIAN_POINT ( 'NONE',  ( 57.60143344285435774, 53.10051614449767499, 2.493737253992045044 ) ) ;
#1789=CARTESIAN_POINT ( 'NONE',  ( 54.13287192849676188, 60.29948385550240886, 5.649768623646098220 ) ) ;
#1792=CARTESIAN_POINT ( 'NONE',  ( 52.62207051974839089, 60.39948385550241028, 7.992620115222770494 ) ) ;
#1794=CARTESIAN_POINT ( 'NONE',  ( 54.13287192849671214, 56.70051614449766220, -5.649768623646139964 ) ) ;
#1803=CARTESIAN_POINT ( 'NONE',  ( 57.36023556966787851, 47.00051614449765935, 0.02388180880515038476 ) ) ;
#1809=CARTESIAN_POINT ( 'NONE',  ( 53.54508667620424234, 44.70051614449765509, -4.840751629271188961 ) ) ;
#1812=CARTESIAN_POINT ( 'NONE',  ( 45.31609314410960820, 50.30051614449766362, -6.485486291978072693 ) ) ;
#1813=CARTESIAN_POINT ( 'NONE',  ( 43.69122665457040000, 56.00051614449765935, -0.02388180880515696977 ) ) ;
#1826=CARTESIAN_POINT ( 'NONE',  ( 54.09612160359786515, 49.69948385550240744, -5.676469297603166098 ) ) ;
#1831=CARTESIAN_POINT ( 'NONE',  ( 43.18075615816994173, 63.80051614449766362, 4.924951120819380357 ) ) ;
#1833=CARTESIAN_POINT ( 'NONE',  ( 56.65037692655918988, 63.89948385550239607, -2.184720259617163762 ) ) ;
#1836=CARTESIAN_POINT ( 'NONE',  ( 44.05948171654945611, 52.20051614449764799, -4.345558710429044069 ) ) ;
#1838=CARTESIAN_POINT ( 'NONE',  ( 55.94051828345050836, 51.79948385550240175, -4.345558710429104465 ) ) ;
#1848=CARTESIAN_POINT ( 'NONE',  ( 55.94051828345050836, 49.79948385550240175, -4.345558710429104465 ) ) ;
#1856=CARTESIAN_POINT ( 'NONE',  ( 56.66441430157294690, 58.90051614449766504, -2.141517661632166281 ) ) ;
#1864=CARTESIAN_POINT ( 'NONE',  ( 44.28664221472221385, 55.90051614449766504, 1.832500667257213722 ) ) ;
#1867=CARTESIAN_POINT ( 'NONE',  ( 48.02776887271745210, 65.39948385550239607, -5.992620115222778487 ) ) ;
#1870=CARTESIAN_POINT ( 'NONE',  ( 41.58830220609386430, 62.00051614449766646, -0.02388180880514929535 ) ) ;
#1888=CARTESIAN_POINT ( 'NONE',  ( 53.50833635130540955, 47.69948385550240744, -4.867452303228209765 ) ) ;
#1890=CARTESIAN_POINT ( 'NONE',  ( 43.20883090819745576, 56.79948385550240175, 4.963592699179006473 ) ) ;
#1891=CARTESIAN_POINT ( 'NONE',  ( 49.97728705011495265, 57.50051614449766646, 7.000000000000000888 ) ) ;
#1894=DIRECTION ( 'NONE',  ( -1.387778780781445991E-14, 0.000000000000000000, -1.000000000000000000 ) ) ;
#1897=VECTOR ( 'NONE', #5185, 1000.000000000000000 ) ;
#1901=CARTESIAN_POINT ( 'NONE',  ( 47.74827507625470702, 46.40051614449765083, -7.007379884777204637 ) ) ;
#1909=CARTESIAN_POINT ( 'NONE',  ( 50.02271294988511841, 60.49948385550240459, 6.000000000000000888 ) ) ;
#1912=CARTESIAN_POINT ( 'NONE',  ( 41.58830220609386430, 58.00051614449765935, -0.02388180880514929535 ) ) ;
#1915=CARTESIAN_POINT ( 'NONE',  ( 55.11794222512599362, 54.80051614449764941, -3.688883143319583446 ) ) ;
#1926=SHAPE_REPRESENTATION ( 'spring', ( #10359 ), #6832 ) ;
#1929=CARTESIAN_POINT ( 'NONE',  ( 55.96859303347805081, 52.19948385550240033, 4.306917132069425058 ) ) ;
#1934=CARTESIAN_POINT ( 'NONE',  ( 41.58830220609386430, 52.99948385550241170, 0.02388180880523263147 ) ) ;
#1937=CARTESIAN_POINT ( 'NONE',  ( 46.45491332379572924, 47.29948385550241596, -4.840751629271157874 ) ) ;
#1942=CARTESIAN_POINT ( 'NONE',  ( 54.09612160359792199, 63.30051614449766362, 5.676469297603124353 ) ) ;
#1944=CARTESIAN_POINT ( 'NONE',  ( 49.97728705011488159, 53.49948385550240459, -7.000000000000000888 ) ) ;
#1948=CARTESIAN_POINT ( 'NONE',  ( 56.65037692655918988, 49.89948385550240317, -2.184720259617163762 ) ) ;
#1960=CARTESIAN_POINT ( 'NONE',  ( 46.45491332379576477, 63.70051614449766930, 4.840751629271188961 ) ) ;
#1964=CARTESIAN_POINT ( 'NONE',  ( 50.02271294988505446, 58.50051614449765225, -8.000000000000001776 ) ) ;
#1982=CARTESIAN_POINT ( 'NONE',  ( 55.96859303347804371, 62.19948385550240744, 4.306917132069425946 ) ) ;
#1984=CARTESIAN_POINT ( 'NONE',  ( 50.02271294988513972, 62.49948385550240459, 8.000000000000001776 ) ) ;
#1985=CARTESIAN_POINT ( 'NONE',  ( 54.13287192849671214, 60.70051614449766220, -5.649768623646139964 ) ) ;
#1995=CARTESIAN_POINT ( 'NONE',  ( 55.94051828345054389, 45.20051614449765509, 4.345558710429044957 ) ) ;
#2002=CARTESIAN_POINT ( 'NONE',  ( 55.08986747509847248, 61.79948385550240175, -3.727524721679197572 ) ) ;
#2004=CARTESIAN_POINT ( 'NONE',  ( 52.29715082351547295, 46.39948385550240317, 6.992620115222774047 ) ) ;
#2006=CARTESIAN_POINT ( 'NONE',  ( 47.42335538002180328, 60.40051614449765793, -8.007379884777206414 ) ) ;
#2007=CARTESIAN_POINT ( 'NONE',  ( 44.91013252490150620, 60.20051614449766220, -3.727524721679154940 ) ) ;
#2020=CARTESIAN_POINT ( 'NONE',  ( 56.65037692655918988, 53.89948385550240317, -2.184720259617163762 ) ) ;
#2026=CARTESIAN_POINT ( 'NONE',  ( 45.31609314410967926, 50.69948385550240744, 6.485486291978119766 ) ) ;
#2029=CARTESIAN_POINT ( 'NONE',  ( 54.13287192849676188, 64.29948385550241596, 5.649768623646098220 ) ) ;
#2030=MANIFOLD_SOLID_BREP ( 'Cavity1', #16195 ) ;
#2033=CARTESIAN_POINT ( 'NONE',  ( 43.34962307344078880, 58.10051614449766078, -2.184720259617096705 ) ) ;
#2035=CARTESIAN_POINT ( 'NONE',  ( 47.74827507625478518, 60.59948385550239891, 7.007379884777227730 ) ) ;
#2041=CARTESIAN_POINT ( 'NONE',  ( 57.36023556966787851, 49.99948385550238328, -0.02388180880522424582 ) ) ;
#2048=CARTESIAN_POINT ( 'NONE',  ( 55.94051828345054389, 63.20051614449764799, 4.345558710429044957 ) ) ;
#2052=CARTESIAN_POINT ( 'NONE',  ( 51.97223112728249816, 62.60051614449765367, -5.992620115222793586 ) ) ;
#2057=CARTESIAN_POINT ( 'NONE',  ( 52.62207051974829852, 58.60051614449766788, -7.992620115222797139 ) ) ;
#2074=CARTESIAN_POINT ( 'NONE',  ( 43.34962307344081012, 64.89948385550239607, 2.184720259617164650 ) ) ;
#2076=CARTESIAN_POINT ( 'NONE',  ( 47.42335538002188144, 58.59948385550239891, 8.007379884777233059 ) ) ;
#2077=CARTESIAN_POINT ( 'NONE',  ( 49.97728705011495265, 59.50051614449765935, 7.000000000000000888 ) ) ;
#2096=CARTESIAN_POINT ( 'NONE',  ( 55.11794222512601493, 64.19948385550240744, 3.688883143319541702 ) ) ;
#2098=CARTESIAN_POINT ( 'NONE',  ( 54.13287192849676188, 46.29948385550240886, 5.649768623646098220 ) ) ;
#2100=CARTESIAN_POINT ( 'NONE',  ( 42.39856655714564226, 60.10051614449766788, -2.493737253992044156 ) ) ;
#2101=CARTESIAN_POINT ( 'NONE',  ( 44.88205777487401349, 63.80051614449766362, 3.688883143319584779 ) ) ;
#2115=CARTESIAN_POINT ( 'NONE',  ( 43.33558569842703179, 51.09948385550240602, -2.141517661632099223 ) ) ;
#2119=CARTESIAN_POINT ( 'NONE',  ( 58.41169779390614281, 51.99948385550239749, -0.02388180880523160798 ) ) ;
#2122=CARTESIAN_POINT ( 'NONE',  ( 57.36023556966787851, 63.99948385550241881, -0.02388180880522424582 ) ) ;
#2126=CARTESIAN_POINT ( 'NONE',  ( 52.25172492374527877, 59.40051614449765083, 7.007379884777203749 ) ) ;
#2127=CARTESIAN_POINT ( 'NONE',  ( 56.66441430157296821, 58.09948385550240602, 2.141517661632100111 ) ) ;
#2132=CIRCLE ( 'NONE', #10569, 0.4999999999999972244 ) ;
#2138=CARTESIAN_POINT ( 'NONE',  ( 54.09612160359786515, 53.69948385550240744, -5.676469297603166098 ) ) ;
#2147=CARTESIAN_POINT ( 'NONE',  ( 49.97728705011488159, 47.49948385550240459, -7.000000000000000888 ) ) ;
#2149=CARTESIAN_POINT ( 'NONE',  ( 48.02776887271750184, 59.60051614449765367, 5.992620115222795363 ) ) ;
#2155=CARTESIAN_POINT ( 'NONE',  ( 42.38452918213190657, 59.90051614449767214, 2.450534656007115508 ) ) ;
#2168=B_SPLINE_CURVE_WITH_KNOTS ( 'NONE', 3,
 ( #13578, #1638, #16728, #7976, #6412, #16821 ),
 .UNSPECIFIED., .F., .F.,
 ( 4, 2, 4 ),
 ( 0.000000000000000000, 0.0003657767439067419277, 0.0007315534878134838555 ),
 .UNSPECIFIED. ) ;
#2175=CARTESIAN_POINT ( 'NONE',  ( 51.92680522751233951, 45.59948385550240602, -6.007379884777223289 ) ) ;
#2177=CARTESIAN_POINT ( 'NONE',  ( 54.68390685589033495, 57.69948385550241454, -6.485486291978119766 ) ) ;
#2179=CARTESIAN_POINT ( 'NONE',  ( 49.97728705011495265, 63.50051614449765935, 7.000000000000000888 ) ) ;
#2188=CARTESIAN_POINT ( 'NONE',  ( 56.65037692655921120, 53.10051614449766078, 2.184720259617097593 ) ) ;
#2197=CARTESIAN_POINT ( 'NONE',  ( 55.96859303347804371, 48.19948385550240033, 4.306917132069425946 ) ) ;
#2200=CARTESIAN_POINT ( 'NONE',  ( 52.62207051974829852, 58.60051614449766788, -7.992620115222797139 ) ) ;
#2202=CARTESIAN_POINT ( 'NONE',  ( 43.69122665457040000, 62.00051614449766646, -0.02388180880515696977 ) ) ;
#2212=VERTEX_POINT ( 'NONE', #8306 ) ;
#2220=CARTESIAN_POINT ( 'NONE',  ( 47.74827507625477807, 60.59948385550239891, 7.007379884777229506 ) ) ;
#2224=CARTESIAN_POINT ( 'NONE',  ( 57.61547081786812896, 54.09948385550241312, 2.450534656007040901 ) ) ;
#2228=CARTESIAN_POINT ( 'NONE',  ( 55.96859303347804371, 64.19948385550239323, 4.306917132069425946 ) ) ;
#2234=CARTESIAN_POINT ( 'NONE',  ( 47.70284917648459100, 59.60051614449765367, 6.992620115222796251 ) ) ;
#2235=CARTESIAN_POINT ( 'NONE',  ( 44.28664221472221385, 45.90051614449766504, 1.832500667257213722 ) ) ;
#2237=CARTESIAN_POINT ( 'NONE',  ( 47.74827507625478518, 58.59948385550238470, 7.007379884777227730 ) ) ;
#2248=CARTESIAN_POINT ( 'NONE',  ( 45.90387839640214196, 54.69948385550240744, 5.676469297603166098 ) ) ;
#2257=CARTESIAN_POINT ( 'NONE',  ( 54.09612160359786515, 47.69948385550240744, -5.676469297603166098 ) ) ;
#2259=CARTESIAN_POINT ( 'NONE',  ( 46.49166364869456913, 64.30051614449766362, -4.867452303228181343 ) ) ;
#2280=CARTESIAN_POINT ( 'NONE',  ( 47.74827507625478518, 62.59948385550240602, 7.007379884777227730 ) ) ;
#2282=CARTESIAN_POINT ( 'NONE',  ( 42.39856655714566358, 64.89948385550239607, 2.493737253992119207 ) ) ;
#2283=CARTESIAN_POINT ( 'NONE',  ( 44.05948171654945611, 64.20051614449765509, -4.345558710429044069 ) ) ;
#2293=CARTESIAN_POINT ( 'NONE',  ( 56.65037692655921120, 55.10051614449766078, 2.184720259617097593 ) ) ;
#2294=CARTESIAN_POINT ( 'NONE',  ( 55.48859070151218020, 45.00000000000002132, -4.999999999999993783 ) ) ;
#2300=CARTESIAN_POINT ( 'NONE',  ( 52.29715082351547295, 48.39948385550240317, 6.992620115222774047 ) ) ;
#2303=CARTESIAN_POINT ( 'NONE',  ( 54.68390685589033495, 47.69948385550240744, -6.485486291978119766 ) ) ;
#2304=CARTESIAN_POINT ( 'NONE',  ( 53.54508667620424234, 62.70051614449766220, -4.840751629271188961 ) ) ;
#2316=CARTESIAN_POINT ( 'NONE',  ( 56.65037692655918988, 59.89948385550241028, -2.184720259617163762 ) ) ;
#2320=CARTESIAN_POINT ( 'NONE',  ( 45.31609314410967926, 52.69948385550240744, 6.485486291978119766 ) ) ;
#2322=CARTESIAN_POINT ( 'NONE',  ( 56.30877334542961421, 51.99948385550239749, -0.02388180880520959434 ) ) ;
#2326=CARTESIAN_POINT ( 'NONE',  ( 54.09612160359792199, 61.30051614449766362, 5.676469297603124353 ) ) ;
#2328=CARTESIAN_POINT ( 'NONE',  ( 51.92680522751233951, 63.59948385550239891, -6.007379884777223289 ) ) ;
#2330=CARTESIAN_POINT ( 'NONE',  ( 44.05948171654949874, 58.79948385550240886, 4.345558710429105354 ) ) ;
#2340=CARTESIAN_POINT ( 'NONE',  ( 56.66441430157296821, 60.09948385550240602, 2.141517661632100111 ) ) ;
#2352=CARTESIAN_POINT ( 'NONE',  ( 52.29715082351547295, 48.39948385550240317, 6.992620115222774047 ) ) ;
#2354=CARTESIAN_POINT ( 'NONE',  ( 52.29715082351538769, 44.60051614449766788, -6.992620115222796251 ) ) ;
#2376=CARTESIAN_POINT ( 'NONE',  ( 44.88205777487398507, 53.19948385550240744, -3.688883143319540814 ) ) ;
#2378=CARTESIAN_POINT ( 'NONE',  ( 52.25172492374522903, 45.59948385550240602, -7.007379884777225953 ) ) ;
#2379=CARTESIAN_POINT ( 'NONE',  ( 44.05948171654945611, 62.20051614449764799, -4.345558710429044069 ) ) ;
#2390=CARTESIAN_POINT ( 'NONE',  ( 47.74827507625470702, 54.40051614449765793, -7.007379884777204637 ) ) ;
#2398=CARTESIAN_POINT ( 'NONE',  ( 54.09612160359786515, 49.69948385550240744, -5.676469297603166098 ) ) ;
#2400=CARTESIAN_POINT ( 'NONE',  ( 50.02271294988513972, 48.49948385550241170, 8.000000000000001776 ) ) ;
#2403=CARTESIAN_POINT ( 'NONE',  ( 46.45491332379576477, 63.70051614449766930, 4.840751629271188961 ) ) ;
#2406=APPLICATION_CONTEXT ( 'automotive_design' ) ;
#2417=CARTESIAN_POINT ( 'NONE',  ( 45.90387839640214196, 58.69948385550240033, 5.676469297603166098 ) ) ;
#2421=CARTESIAN_POINT ( 'NONE',  ( 56.81924384183011512, 58.19948385550240744, 4.924951120819313743 ) ) ;
#2424=CARTESIAN_POINT ( 'NONE',  ( 44.28664221472220675, 53.09948385550240602, -1.832500667257165317 ) ) ;
#2427=CARTESIAN_POINT ( 'NONE',  ( 50.02271294988505446, 44.50051614449765935, -8.000000000000001776 ) ) ;
#2428=CARTESIAN_POINT ( 'NONE',  ( 44.30067958973596376, 62.89948385550240317, 1.875703265242204099 ) ) ;
#2438=CARTESIAN_POINT ( 'NONE',  ( 50.02271294988512551, 56.49948385550240459, 7.000000000000000888 ) ) ;
#2446=CARTESIAN_POINT ( 'NONE',  ( 56.65037692655918988, 53.89948385550240317, -2.184720259617163762 ) ) ;
#2448=CARTESIAN_POINT ( 'NONE',  ( 43.33558569842706021, 49.90051614449766504, 2.141517661632167169 ) ) ;
#2473=CARTESIAN_POINT ( 'NONE',  ( 44.30067958973596376, 64.89948385550239607, 1.875703265242204099 ) ) ;
#2478=CARTESIAN_POINT ( 'NONE',  ( 55.69932041026404335, 51.89948385550241028, -1.875703265242203432 ) ) ;
#2480=CARTESIAN_POINT ( 'NONE',  ( 47.70284917648453415, 49.39948385550238896, -6.992620115222774047 ) ) ;
#2481=CARTESIAN_POINT ( 'NONE',  ( 57.61547081786810764, 46.90051614449766504, -2.450534656007114176 ) ) ;
#2491=CARTESIAN_POINT ( 'NONE',  ( 45.90387839640208512, 54.30051614449765651, -5.676469297603124353 ) ) ;
#2501=CARTESIAN_POINT ( 'NONE',  ( 43.33558569842703179, 53.09948385550240602, -2.141517661632099223 ) ) ;
#2503=CARTESIAN_POINT ( 'NONE',  ( 58.41169779390614281, 45.99948385550240459, -0.02388180880523160798 ) ) ;
#2505=CARTESIAN_POINT ( 'NONE',  ( 52.25172492374527877, 51.40051614449767214, 7.007379884777203749 ) ) ;
#2518=CARTESIAN_POINT ( 'NONE',  ( 54.09612160359786515, 57.69948385550240744, -5.676469297603166098 ) ) ;
#2524=CARTESIAN_POINT ( 'NONE',  ( 45.31609314410967926, 60.69948385550240033, 6.485486291978119766 ) ) ;
#2527=CARTESIAN_POINT ( 'NONE',  ( 53.50833635130540955, 47.69948385550240744, -4.867452303228209765 ) ) ;
#2531=CARTESIAN_POINT ( 'NONE',  ( 44.05948171654945611, 64.20051614449765509, -4.345558710429044069 ) ) ;
#2533=CARTESIAN_POINT ( 'NONE',  ( 44.28664221472220675, 61.09948385550241312, -1.832500667257165317 ) ) ;
#2541=CARTESIAN_POINT ( 'NONE',  ( 47.74827507625478518, 60.59948385550239891, 7.007379884777227730 ) ) ;
#2552=CARTESIAN_POINT ( 'NONE',  ( 55.96859303347804371, 54.19948385550240033, 4.306917132069425946 ) ) ;
#2555=CARTESIAN_POINT ( 'NONE',  ( 52.25172492374527877, 49.40051614449766504, 7.007379884777203749 ) ) ;
#2577=CARTESIAN_POINT ( 'NONE',  ( 51.92680522751238925, 51.40051614449767214, 6.007379884777208190 ) ) ;
#2581=CARTESIAN_POINT ( 'NONE',  ( 56.30877334542961421, 49.99948385550240459, -0.02388180880520959434 ) ) ;
#2583=CARTESIAN_POINT ( 'NONE',  ( 49.97728705011488159, 45.49948385550240459, -7.000000000000000888 ) ) ;
#2584=CARTESIAN_POINT ( 'NONE',  ( 58.41169779390614281, 45.00051614449765225, 0.02388180880515032231 ) ) ;
#2596=CARTESIAN_POINT ( 'NONE',  ( 57.36023556966787851, 55.00051614449765935, 0.02388180880515038476 ) ) ;
#2598=CARTESIAN_POINT ( 'NONE',  ( 55.48859070151218020, 45.00000000000002132, -4.999999999999993783 ) ) ;
#2603=CARTESIAN_POINT ( 'NONE',  ( 52.25172492374522903, 53.59948385550241312, -7.007379884777225953 ) ) ;
#2606=CARTESIAN_POINT ( 'NONE',  ( 45.31609314410960820, 64.30051614449766362, -6.485486291978072693 ) ) ;
#2608=CARTESIAN_POINT ( 'NONE',  ( 57.36023556966787851, 47.00051614449764514, 0.02388180880515038476 ) ) ;
#2622=CARTESIAN_POINT ( 'NONE',  ( 45.27934281921075410, 57.29948385550240175, -6.458785618021043895 ) ) ;
#2625=CARTESIAN_POINT ( 'NONE',  ( 44.88205777487398507, 51.19948385550240744, -3.688883143319540814 ) ) ;
#2628=CARTESIAN_POINT ( 'NONE',  ( 56.81924384183006538, 48.80051614449767072, -4.924951120819380357 ) ) ;
#2629=CARTESIAN_POINT ( 'NONE',  ( 44.30067958973594955, 48.10051614449766078, -1.875703265242155693 ) ) ;
#2639=CARTESIAN_POINT ( 'NONE',  ( 57.36023556966787851, 57.99948385550239038, -0.02388180880522424582 ) ) ;
#2649=CARTESIAN_POINT ( 'NONE',  ( 43.33558569842703179, 51.09948385550240602, -2.141517661632099223 ) ) ;
#2651=CARTESIAN_POINT ( 'NONE',  ( 57.36023556966787851, 45.00051614449763804, 0.02388180880515038476 ) ) ;
#2670=CARTESIAN_POINT ( 'NONE',  ( 53.54508667620424234, 46.70051614449766220, -4.840751629271188961 ) ) ;
#2673=CARTESIAN_POINT ( 'NONE',  ( 55.11794222512601493, 54.19948385550241454, 3.688883143319541702 ) ) ;
#2675=CARTESIAN_POINT ( 'NONE',  ( 44.05948171654949874, 48.79948385550238754, 4.345558710429105354 ) ) ;
#2676=CARTESIAN_POINT ( 'NONE',  ( 45.31609314410960820, 46.30051614449766362, -6.485486291978072693 ) ) ;
#2692=CARTESIAN_POINT ( 'NONE',  ( 56.65037692655918988, 49.89948385550240317, -2.184720259617163762 ) ) ;
#2694=CARTESIAN_POINT ( 'NONE',  ( 42.39856655714564226, 64.10051614449766078, -2.493737253992044156 ) ) ;
#2697=CARTESIAN_POINT ( 'NONE',  ( 49.97728705011495265, 49.50051614449765935, 7.000000000000000888 ) ) ;
#2714=CARTESIAN_POINT ( 'NONE',  ( 56.81924384183011512, 60.19948385550240744, 4.924951120819313743 ) ) ;
#2716=CARTESIAN_POINT ( 'NONE',  ( 55.08986747509847248, 53.79948385550241596, -3.727524721679197572 ) ) ;
#2719=CARTESIAN_POINT ( 'NONE',  ( 52.62207051974829852, 46.60051614449764656, -7.992620115222797139 ) ) ;
#2721=CARTESIAN_POINT ( 'NONE',  ( 49.97728705011494554, 49.50051614449766646, 6.000000000000000888 ) ) ;
#2730=CARTESIAN_POINT ( 'NONE',  ( 49.97728705011488159, 57.49948385550241170, -7.000000000000000888 ) ) ;
#2740=CARTESIAN_POINT ( 'NONE',  ( 45.90387839640214196, 50.69948385550240744, 5.676469297603166098 ) ) ;
#2743=CARTESIAN_POINT ( 'NONE',  ( 44.05948171654945611, 48.20051614449764799, -4.345558710429044069 ) ) ;
#2748=PRODUCT_DEFINITION_SHAPE ( 'NONE', 'NONE',  #3281 ) ;
#2761=CARTESIAN_POINT ( 'NONE',  ( 51.92680522751238925, 47.40051614449765793, 6.007379884777208190 ) ) ;
#2765=CARTESIAN_POINT ( 'NONE',  ( 46.45491332379572924, 53.29948385550240886, -4.840751629271157874 ) ) ;
#2768=CARTESIAN_POINT ( 'NONE',  ( 56.65037692655918988, 49.89948385550240317, -2.184720259617163762 ) ) ;
#2769=CARTESIAN_POINT ( 'NONE',  ( 54.72065718078918906, 44.70051614449765509, -6.458785618021089192 ) ) ;
#2783=CARTESIAN_POINT ( 'NONE',  ( 52.29715082351547295, 54.39948385550239607, 6.992620115222774047 ) ) ;
#2785=CARTESIAN_POINT ( 'NONE',  ( 56.81924384183011512, 52.19948385550240744, 4.924951120819313743 ) ) ;
#2788=CARTESIAN_POINT ( 'NONE',  ( 47.74827507625469281, 50.40051614449764372, -7.007379884777203749 ) ) ;
#2803=CARTESIAN_POINT ( 'NONE',  ( 52.62207051974839089, 58.39948385550241028, 7.992620115222770494 ) ) ;
#2805=CARTESIAN_POINT ( 'NONE',  ( 51.92680522751233951, 55.59948385550240602, -6.007379884777223289 ) ) ;
#2809=CARTESIAN_POINT ( 'NONE',  ( 56.79116909180259398, 49.20051614449766220, 4.963592699178938972 ) ) ;
#2810=CARTESIAN_POINT ( 'NONE',  ( 44.28664221472221385, 51.90051614449765793, 1.832500667257213722 ) ) ;
#2826=CARTESIAN_POINT ( 'NONE',  ( 55.96859303347805081, 46.19948385550240033, 4.306917132069425058 ) ) ;
#2833=CARTESIAN_POINT ( 'NONE',  ( 43.34962307344081012, 48.89948385550240317, 2.184720259617164650 ) ) ;
#2835=CARTESIAN_POINT ( 'NONE',  ( 47.70284917648459100, 49.60051614449763946, 6.992620115222796251 ) ) ;
#2846=CARTESIAN_POINT ( 'NONE',  ( 47.74827507625478518, 48.59948385550239180, 7.007379884777227730 ) ) ;
#2858=CARTESIAN_POINT ( 'NONE',  ( 56.30877334542961421, 47.00051614449766646, 0.02388180880515774693 ) ) ;
#2862=CARTESIAN_POINT ( 'NONE',  ( 44.91013252490152752, 54.79948385550240175, 3.727524721679198461 ) ) ;
#2865=CARTESIAN_POINT ( 'NONE',  ( 45.90387839640214196, 54.69948385550240744, 5.676469297603166098 ) ) ;
#2866=CARTESIAN_POINT ( 'NONE',  ( 54.68390685589039890, 47.30051614449766362, 6.485486291978072693 ) ) ;
#2871=CARTESIAN_POINT ( 'NONE',  ( 0.000000000000000000, 0.000000000000000000, 0.000000000000000000 ) ) ;
#2885=CARTESIAN_POINT ( 'NONE',  ( 56.66441430157296821, 56.09948385550240602, 2.141517661632100111 ) ) ;
#2887=CARTESIAN_POINT ( 'NONE',  ( 49.97728705011486738, 53.49948385550240459, -8.000000000000001776 ) ) ;
#2890=CARTESIAN_POINT ( 'NONE',  ( 47.74827507625469281, 46.40051614449764372, -7.007379884777203749 ) ) ;
#2905=CARTESIAN_POINT ( 'NONE',  ( 44.28664221472220675, 57.09948385550240602, -1.832500667257165317 ) ) ;
#2908=CARTESIAN_POINT ( 'NONE',  ( 54.68390685589039890, 51.30051614449765651, 6.485486291978072693 ) ) ;
#2909=CARTESIAN_POINT ( 'NONE',  ( 55.11794222512599362, 48.80051614449767072, -3.688883143319583446 ) ) ;
#2925=CARTESIAN_POINT ( 'NONE',  ( 51.51576781266200555, 45.00000000000000711, -6.337576802645323859 ) ) ;
#2926=CARTESIAN_POINT ( 'NONE',  ( 42.63976443033212860, 58.99948385550239038, 0.02388180880522514787 ) ) ;
#2929=CARTESIAN_POINT ( 'NONE',  ( 54.13287192849671214, 52.70051614449766220, -5.649768623646139964 ) ) ;
#2939=CARTESIAN_POINT ( 'NONE',  ( 47.37792948025162332, 63.39948385550238896, -7.992620115222770494 ) ) ;
#2942=EDGE_CURVE ( 'NONE', #17307, #18471, #10397, .T. ) ;
#2945=CARTESIAN_POINT ( 'NONE',  ( 43.33558569842706021, 57.90051614449766504, 2.141517661632167169 ) ) ;
#2949=CARTESIAN_POINT ( 'NONE',  ( 55.71335778527780036, 46.90051614449766504, -1.832500667257213056 ) ) ;
#2953=CARTESIAN_POINT ( 'NONE',  ( 46.49166364869460466, 54.69948385550240033, 4.867452303228209765 ) ) ;
#2955=CARTESIAN_POINT ( 'NONE',  ( 47.74827507625478518, 54.59948385550239180, 7.007379884777227730 ) ) ;
#2958=CARTESIAN_POINT ( 'NONE',  ( 58.41169779390614281, 55.00051614449766646, 0.02388180880515032231 ) ) ;
#2973=CARTESIAN_POINT ( 'NONE',  ( 45.90387839640214196, 60.69948385550240033, 5.676469297603166098 ) ) ;
#2975=CARTESIAN_POINT ( 'NONE',  ( 42.39856655714566358, 52.89948385550241028, 2.493737253992119207 ) ) ;
#2977=CARTESIAN_POINT ( 'NONE',  ( 44.03140696652198471, 57.80051614449766362, 4.306917132069485454 ) ) ;
#2997=CARTESIAN_POINT ( 'NONE',  ( 51.92680522751233951, 59.59948385550240602, -6.007379884777223289 ) ) ;
#3000=CARTESIAN_POINT ( 'NONE',  ( 47.37792948025170858, 53.60051614449765367, 7.992620115222797139 ) ) ;
#3003=CARTESIAN_POINT ( 'NONE',  ( 44.30067958973594955, 58.10051614449765367, -1.875703265242155693 ) ) ;
#3010=CARTESIAN_POINT ( 'NONE',  ( 45.90387839640214196, 62.69948385550240744, 5.676469297603166098 ) ) ;
#3015=CARTESIAN_POINT ( 'NONE',  ( 49.97728705011488159, 45.49948385550240459, -7.000000000000000888 ) ) ;
#3019=CARTESIAN_POINT ( 'NONE',  ( 49.97728705011495265, 63.50051614449765935, 8.000000000000001776 ) ) ;
#3020=CARTESIAN_POINT ( 'NONE',  ( 53.61415392313774220, 44.99999999999997868, -5.449226822604907206 ) ) ;
#3021=CARTESIAN_POINT ( 'NONE',  ( 43.34962307344081012, 54.89948385550240317, 2.184720259617164650 ) ) ;
#3025=CARTESIAN_POINT ( 'NONE',  ( 55.96859303347802239, 56.80051614449764230, -4.306917132069484566 ) ) ;
#3034=CARTESIAN_POINT ( 'NONE',  ( 52.25172492374522903, 47.59948385550239891, -7.007379884777225953 ) ) ;
#3039=CARTESIAN_POINT ( 'NONE',  ( 45.86712807150329496, 57.70051614449765509, 5.649768623646139964 ) ) ;
#3047=CARTESIAN_POINT ( 'NONE',  ( 49.97728705011494554, 53.50051614449767357, 6.000000000000000888 ) ) ;
#3052=CARTESIAN_POINT ( 'NONE',  ( 44.28664221472220675, 57.09948385550240602, -1.832500667257165317 ) ) ;
#3054=CARTESIAN_POINT ( 'NONE',  ( 43.18075615816994173, 55.80051614449766362, 4.924951120819380357 ) ) ;
#3070=CARTESIAN_POINT ( 'NONE',  ( 50.02271294988512551, 64.49948385550240459, 7.000000000000000888 ) ) ;
#3076=CARTESIAN_POINT ( 'NONE',  ( 52.25172492374522903, 59.59948385550240602, -7.007379884777225953 ) ) ;
#3078=CARTESIAN_POINT ( 'NONE',  ( 58.41169779390614281, 51.99948385550239749, -0.02388180880523160798 ) ) ;
#3080=CARTESIAN_POINT ( 'NONE',  ( 49.97728705011495265, 53.50051614449765935, 7.000000000000000888 ) ) ;
#3091=CARTESIAN_POINT ( 'NONE',  ( 55.94051828345050836, 63.79948385550240886, -4.345558710429104465 ) ) ;
#3092=CARTESIAN_POINT ( 'NONE',  ( 50.02271294988505446, 44.50051614449765935, -7.000000000000000888 ) ) ;
#3098=CARTESIAN_POINT ( 'NONE',  ( 44.88205777487398507, 55.19948385550240744, -3.688883143319540814 ) ) ;
#3101=CARTESIAN_POINT ( 'NONE',  ( 52.57664461997821093, 55.40051614449767214, 8.007379884777206414 ) ) ;
#3102=CARTESIAN_POINT ( 'NONE',  ( 44.30067958973594955, 54.10051614449766078, -1.875703265242155693 ) ) ;
#3112=CARTESIAN_POINT ( 'NONE',  ( 55.94051828345050836, 61.79948385550239465, -4.345558710429104465 ) ) ;
#3121=CARTESIAN_POINT ( 'NONE',  ( 50.02271294988505446, 64.50051614449766646, -8.000000000000001776 ) ) ;
#3123=CARTESIAN_POINT ( 'NONE',  ( 56.65037692655918988, 59.89948385550241028, -2.184720259617163762 ) ) ;
#3126=CARTESIAN_POINT ( 'NONE',  ( 52.29715082351538769, 54.60051614449766788, -6.992620115222796251 ) ) ;
#3137=CARTESIAN_POINT ( 'NONE',  ( 56.65037692655918988, 47.89948385550240317, -2.184720259617163762 ) ) ;
#3142=CARTESIAN_POINT ( 'NONE',  ( 56.65037692655921120, 57.10051614449766078, 2.184720259617097593 ) ) ;
#3147=CARTESIAN_POINT ( 'NONE',  ( 51.92680522751238925, 53.40051614449765793, 6.007379884777208190 ) ) ;
#3149=CARTESIAN_POINT ( 'NONE',  ( 50.02271294988511841, 58.49948385550241170, 6.000000000000000888 ) ) ;
#3152=CARTESIAN_POINT ( 'NONE',  ( 58.41169779390614281, 51.00051614449765935, 0.02388180880515032231 ) ) ;
#3173=CARTESIAN_POINT ( 'NONE',  ( 55.96859303347804371, 56.19948385550241454, 4.306917132069425946 ) ) ;
#3176=CARTESIAN_POINT ( 'NONE',  ( 50.02271294988513972, 56.49948385550240459, 8.000000000000001776 ) ) ;
#3178=CARTESIAN_POINT ( 'NONE',  ( 52.29715082351538769, 52.60051614449766788, -6.992620115222796251 ) ) ;
#3184=ORIENTED_EDGE ( 'NONE', *, *, #1535, .F. ) ;
#3194=CARTESIAN_POINT ( 'NONE',  ( 56.30877334542961421, 57.99948385550241170, -0.02388180880520959434 ) ) ;
#3198=CARTESIAN_POINT ( 'NONE',  ( 50.02271294988505446, 50.50051614449765935, -8.000000000000001776 ) ) ;
#3199=CARTESIAN_POINT ( 'NONE',  ( 50.02271294988506156, 56.50051614449767357, -6.000000000000000888 ) ) ;
#3209=CARTESIAN_POINT ( 'NONE',  ( 55.94051828345050836, 63.79948385550240886, -4.345558710429104465 ) ) ;
#3213=CARTESIAN_POINT ( 'NONE',  ( 49.97728705011488159, 49.49948385550240459, -7.000000000000000888 ) ) ;
#3217=CARTESIAN_POINT ( 'NONE',  ( 56.79116909180259398, 63.20051614449766220, 4.963592699178938972 ) ) ;
#3219=CARTESIAN_POINT ( 'NONE',  ( 52.29715082351547295, 56.39948385550238896, 6.992620115222774047 ) ) ;
#3221=CARTESIAN_POINT ( 'NONE',  ( 45.86712807150329496, 51.70051614449766220, 5.649768623646139964 ) ) ;
#3231=CARTESIAN_POINT ( 'NONE',  ( 56.79116909180255135, 63.79948385550241596, -4.963592699179005585 ) ) ;
#3236=CARTESIAN_POINT ( 'NONE',  ( 44.03140696652198471, 57.80051614449766362, 4.306917132069485454 ) ) ;
#3242=CARTESIAN_POINT ( 'NONE',  ( 44.88205777487401349, 57.80051614449766362, 3.688883143319584779 ) ) ;
#3246=CARTESIAN_POINT ( 'NONE',  ( 55.69932041026404335, 59.89948385550240317, -1.875703265242203432 ) ) ;
#3248=CARTESIAN_POINT ( 'NONE',  ( 49.97728705011495265, 55.50051614449766646, 8.000000000000001776 ) ) ;
#3253=PRODUCT_CONTEXT ( 'NONE', #2406, 'mechanical' ) ;
#3257=CARTESIAN_POINT ( 'NONE',  ( 47.70284917648453415, 61.39948385550241028, -6.992620115222774047 ) ) ;
#3261=CARTESIAN_POINT ( 'NONE',  ( 52.25172492374522903, 61.59948385550239891, -7.007379884777225953 ) ) ;
#3263=CARTESIAN_POINT ( 'NONE',  ( 43.20883090819745576, 58.79948385550240175, 4.963592699179006473 ) ) ;
#3264=CARTESIAN_POINT ( 'NONE',  ( 43.34962307344078880, 56.10051614449766078, -2.184720259617096705 ) ) ;
#3269=CARTESIAN_POINT ( 'NONE',  ( 45.86712807150329496, 45.70051614449766220, 5.649768623646139964 ) ) ;
#3270=CARTESIAN_POINT ( 'NONE',  ( 44.05948171654949874, 64.79948385550240175, 4.345558710429105354 ) ) ;
#3276=CARTESIAN_POINT ( 'NONE',  ( 56.30877334542961421, 45.00051614449765225, 0.02388180880515774693 ) ) ;
#3279=CARTESIAN_POINT ( 'NONE',  ( 47.42335538002180328, 52.40051614449767214, -8.007379884777206414 ) ) ;
#3281=PRODUCT_DEFINITION ( 'UNKNOWN', '', #14811, #18341 ) ;
#3282=CARTESIAN_POINT ( 'NONE',  ( 51.92680522751238925, 53.40051614449765793, 6.007379884777208190 ) ) ;
#3300=CARTESIAN_POINT ( 'NONE',  ( 57.36023556966787851, 49.99948385550239749, -0.02388180880522424582 ) ) ;
#3304=CARTESIAN_POINT ( 'NONE',  ( 50.02271294988513972, 48.49948385550241170, 8.000000000000001776 ) ) ;
#3308=CARTESIAN_POINT ( 'NONE',  ( 56.66441430157296821, 58.09948385550240602, 2.141517661632100111 ) ) ;
#3312=CARTESIAN_POINT ( 'NONE',  ( 54.09612160359792199, 53.30051614449766362, 5.676469297603124353 ) ) ;
#3314=CARTESIAN_POINT ( 'NONE',  ( 45.90387839640214196, 52.69948385550240033, 5.676469297603166098 ) ) ;
#3319=ORIENTED_EDGE ( 'NONE', *, *, #1535, .T. ) ;
#3321=CARTESIAN_POINT ( 'NONE',  ( 43.33558569842703179, 55.09948385550241312, -2.141517661632099223 ) ) ;
#3327=CARTESIAN_POINT ( 'NONE',  ( 50.02271294988505446, 58.50051614449765935, -7.000000000000000888 ) ) ;
#3331=CARTESIAN_POINT ( 'NONE',  ( 48.07319477248762496, 58.40051614449765793, -6.007379884777208190 ) ) ;
#3336=CARTESIAN_POINT ( 'NONE',  ( 55.71335778527780747, 62.09948385550240602, 1.832500667257165983 ) ) ;
#3338=CARTESIAN_POINT ( 'NONE',  ( 42.38452918213190657, 61.90051614449766504, 2.450534656007115508 ) ) ;
#3351=CARTESIAN_POINT ( 'NONE',  ( 52.25172492374522903, 63.59948385550239180, -7.007379884777227730 ) ) ;
#3356=CARTESIAN_POINT ( 'NONE',  ( 48.02776887271745210, 47.39948385550241028, -5.992620115222778487 ) ) ;
#3358=CARTESIAN_POINT ( 'NONE',  ( 56.79116909180255135, 61.79948385550240175, -4.963592699179005585 ) ) ;
#3359=CARTESIAN_POINT ( 'NONE',  ( 55.94051828345053679, 57.20051614449766930, 4.345558710429044069 ) ) ;
#3367=CARTESIAN_POINT ( 'NONE',  ( 56.65037692655918988, 61.89948385550241028, -2.184720259617163762 ) ) ;
#3372=CARTESIAN_POINT ( 'NONE',  ( 55.08986747509847248, 63.79948385550241596, -3.727524721679197572 ) ) ;
#3376=CARTESIAN_POINT ( 'NONE',  ( 57.61547081786810764, 58.90051614449766504, -2.450534656007114176 ) ) ;
#3377=CARTESIAN_POINT ( 'NONE',  ( 55.69932041026405045, 57.10051614449766788, 1.875703265242156359 ) ) ;
#3391=CARTESIAN_POINT ( 'NONE',  ( 50.02271294988512551, 52.49948385550240459, 7.000000000000000888 ) ) ;
#3396=CARTESIAN_POINT ( 'NONE',  ( 47.37792948025162332, 49.39948385550241028, -7.992620115222770494 ) ) ;
#3398=CARTESIAN_POINT ( 'NONE',  ( 56.30877334542961421, 45.99948385550240459, -0.02388180880520959434 ) ) ;
#3402=CARTESIAN_POINT ( 'NONE',  ( 57.36023556966787851, 63.00051614449767357, 0.02388180880515038476 ) ) ;
#3405=CARTESIAN_POINT ( 'NONE',  ( 54.13287192849676188, 52.29948385550240886, 5.649768623646098220 ) ) ;
#3414=CARTESIAN_POINT ( 'NONE',  ( 49.97728705011488159, 49.49948385550240459, -7.000000000000000888 ) ) ;
#3429=CARTESIAN_POINT ( 'NONE',  ( 44.30067958973594955, 56.10051614449766078, -1.875703265242155693 ) ) ;
#3435=CARTESIAN_POINT ( 'NONE',  ( 47.42335538002180328, 62.40051614449765793, -8.007379884777206414 ) ) ;
#3453=CARTESIAN_POINT ( 'NONE',  ( 56.66441430157296821, 64.09948385550239891, 2.141517661632100111 ) ) ;
#3455=CARTESIAN_POINT ( 'NONE',  ( 45.27934281921075410, 57.29948385550240175, -6.458785618021043895 ) ) ;
#3456=CARTESIAN_POINT ( 'NONE',  ( 49.97728705011495265, 61.50051614449765935, 7.000000000000000888 ) ) ;
#3462=EDGE_LOOP ( 'NONE', ( #1735, #1414, #15069, #8475, #5824, #17918 ) ) ;
#3467=CARTESIAN_POINT ( 'NONE',  ( 56.65037692655921120, 47.10051614449766078, 2.184720259617097593 ) ) ;
#3468=CARTESIAN_POINT ( 'NONE',  ( 52.25172492374522903, 61.59948385550239891, -7.007379884777225953 ) ) ;
#3474=CARTESIAN_POINT ( 'NONE',  ( 49.97728705011488870, 61.49948385550241170, -6.000000000000000888 ) ) ;
#3477=CARTESIAN_POINT ( 'NONE',  ( 57.61547081786810764, 60.90051614449766504, -2.450534656007114176 ) ) ;
#3479=CARTESIAN_POINT ( 'NONE',  ( 51.97223112728249816, 60.60051614449765367, -5.992620115222793586 ) ) ;
#3491=CARTESIAN_POINT ( 'NONE',  ( 47.70284917648453415, 49.39948385550239607, -6.992620115222774047 ) ) ;
#3496=CARTESIAN_POINT ( 'NONE',  ( 42.38452918213188525, 53.09948385550240602, -2.450534656007040013 ) ) ;
#3499=CARTESIAN_POINT ( 'NONE',  ( 42.63976443033212860, 64.99948385550240459, 0.02388180880522514787 ) ) ;
#3503=CARTESIAN_POINT ( 'NONE',  ( 43.33558569842706021, 63.90051614449765793, 2.141517661632167169 ) ) ;
#3505=CARTESIAN_POINT ( 'NONE',  ( 43.34962307344081012, 60.89948385550241028, 2.184720259617164650 ) ) ;
#3510=CARTESIAN_POINT ( 'NONE',  ( 44.03140696652192787, 51.19948385550238612, -4.306917132069425058 ) ) ;
#3518=CARTESIAN_POINT ( 'NONE',  ( 47.74827507625478518, 46.59948385550239891, 7.007379884777227730 ) ) ;
#3520=CARTESIAN_POINT ( 'NONE',  ( 53.54508667620424234, 62.70051614449766220, -4.840751629271188961 ) ) ;
#3525=CARTESIAN_POINT ( 'NONE',  ( 56.81924384183006538, 60.80051614449766362, -4.924951120819380357 ) ) ;
#3530=SURFACE_STYLE_USAGE ( .BOTH. , #8313 ) ;
#3540=CARTESIAN_POINT ( 'NONE',  ( 47.37792948025162332, 65.39948385550239607, -7.992620115222770494 ) ) ;
#3547=CARTESIAN_POINT ( 'NONE',  ( 57.36023556966787851, 61.99948385550241170, -0.02388180880522424582 ) ) ;
#3549=CARTESIAN_POINT ( 'NONE',  ( 42.38452918213188525, 57.09948385550240602, -2.450534656007040013 ) ) ;
#3550=CARTESIAN_POINT ( 'NONE',  ( 55.94051828345053679, 61.20051614449766220, 4.345558710429044069 ) ) ;
#3555=CARTESIAN_POINT ( 'NONE',  ( 56.13503143586221000, 44.82443585060838132, -3.788959942617806220 ) ) ;
#3561=CARTESIAN_POINT ( 'NONE',  ( 49.97728705011488870, 63.49948385550241170, -6.000000000000000888 ) ) ;
#3566=CARTESIAN_POINT ( 'NONE',  ( 57.61547081786810764, 62.90051614449765083, -2.450534656007114176 ) ) ;
#3567=CARTESIAN_POINT ( 'NONE',  ( 51.92680522751238925, 63.40051614449765083, 6.007379884777208190 ) ) ;
#3581=CARTESIAN_POINT ( 'NONE',  ( 45.90387839640214196, 50.69948385550240744, 5.676469297603166098 ) ) ;
#3587=CARTESIAN_POINT ( 'NONE',  ( 41.58830220609386430, 50.99948385550241170, 0.02388180880523263147 ) ) ;
#3591=CARTESIAN_POINT ( 'NONE',  ( 47.74827507625478518, 64.59948385550239891, 7.007379884777227730 ) ) ;
#3594=CARTESIAN_POINT ( 'NONE',  ( 47.74827507625469281, 58.40051614449766504, -7.007379884777203749 ) ) ;
#3595=CARTESIAN_POINT ( 'NONE',  ( 45.86712807150323812, 59.29948385550240175, -5.649768623646098220 ) ) ;
#3601=CARTESIAN_POINT ( 'NONE',  ( 45.90387839640214196, 52.69948385550240033, 5.676469297603166098 ) ) ;
#3608=CARTESIAN_POINT ( 'NONE',  ( 52.25172492374528588, 63.40051614449765083, 7.007379884777204637 ) ) ;
#3610=CARTESIAN_POINT ( 'NONE',  ( 55.94051828345050836, 45.79948385550240886, -4.345558710429104465 ) ) ;
#3612=CARTESIAN_POINT ( 'NONE',  ( 44.28664221472221385, 61.90051614449766504, 1.832500667257213722 ) ) ;
#3616=CARTESIAN_POINT ( 'NONE',  ( 45.31609314410960820, 58.30051614449765651, -6.485486291978072693 ) ) ;
#3620=FILL_AREA_STYLE_COLOUR ( '', #12154 ) ;
#3638=CARTESIAN_POINT ( 'NONE',  ( 55.94051828345050836, 61.79948385550239465, -4.345558710429104465 ) ) ;
#3640=CARTESIAN_POINT ( 'NONE',  ( 42.38452918213188525, 61.09948385550241312, -2.450534656007040013 ) ) ;
#3641=CARTESIAN_POINT ( 'NONE',  ( 56.66441430157294690, 60.90051614449766504, -2.141517661632166281 ) ) ;
#3649=PRODUCT ( 'spring', 'spring', '', ( #3253 ) ) ;
#3663=CARTESIAN_POINT ( 'NONE',  ( 52.62207051974829852, 62.60051614449765367, -7.992620115222797139 ) ) ;
#3664=CARTESIAN_POINT ( 'NONE',  ( 51.97223112728249816, 62.60051614449765367, -5.992620115222793586 ) ) ;
#3676=CARTESIAN_POINT ( 'NONE',  ( 52.29715082351547295, 58.39948385550240317, 6.992620115222774047 ) ) ;
#3681=CARTESIAN_POINT ( 'NONE',  ( 56.81924384183011512, 50.19948385550241454, 4.924951120819313743 ) ) ;
#3684=CARTESIAN_POINT ( 'NONE',  ( 45.90387839640214196, 62.69948385550240744, 5.676469297603166098 ) ) ;
#3688=CARTESIAN_POINT ( 'NONE',  ( 47.70284917648459100, 57.60051614449764656, 6.992620115222796251 ) ) ;
#3689=CARTESIAN_POINT ( 'NONE',  ( 51.97223112728254790, 62.39948385550240317, 5.992620115222778487 ) ) ;
#3690=CARTESIAN_POINT ( 'NONE',  ( 57.36023556966787851, 57.99948385550239038, -0.02388180880522424582 ) ) ;
#3701=CARTESIAN_POINT ( 'NONE',  ( 52.29715082351547295, 54.39948385550239607, 6.992620115222774047 ) ) ;
#3707=CARTESIAN_POINT ( 'NONE',  ( 57.36023556966787851, 63.00051614449767357, 0.02388180880515038476 ) ) ;
#3709=FACE_OUTER_BOUND ( 'NONE', #3462, .T. ) ;
#3711=CARTESIAN_POINT ( 'NONE',  ( 43.69122665457040000, 60.00051614449765935, -0.02388180880515696977 ) ) ;
#3717=CARTESIAN_POINT ( 'NONE',  ( 43.18075615816994173, 61.80051614449766362, 4.924951120819380357 ) ) ;
#3734=CARTESIAN_POINT ( 'NONE',  ( 50.02271294988512551, 62.49948385550240459, 7.000000000000000888 ) ) ;
#3736=CARTESIAN_POINT ( 'NONE',  ( 49.97728705011486738, 65.49948385550240459, -8.000000000000001776 ) ) ;
#3739=CARTESIAN_POINT ( 'NONE',  ( 42.63976443033212860, 64.00051614449765225, -0.02388180880514948964 ) ) ;
#3747=CARTESIAN_POINT ( 'NONE',  ( 47.74827507625470702, 50.40051614449765793, -7.007379884777204637 ) ) ;
#3749=CARTESIAN_POINT ( 'NONE',  ( 53.94396537754659704, 44.99999999999997158, -6.362703256440709332 ) ) ;
#3756=CARTESIAN_POINT ( 'NONE',  ( 45.86712807150323812, 47.29948385550240886, -5.649768623646098220 ) ) ;
#3758=CARTESIAN_POINT ( 'NONE',  ( 56.81924384183006538, 58.80051614449766362, -4.924951120819380357 ) ) ;
#3760=CARTESIAN_POINT ( 'NONE',  ( 55.11794222512599362, 62.80051614449766362, -3.688883143319583446 ) ) ;
#3779=CARTESIAN_POINT ( 'NONE',  ( 56.65037692655918988, 55.89948385550240317, -2.184720259617163762 ) ) ;
#3783=CARTESIAN_POINT ( 'NONE',  ( 54.68390685589033495, 51.69948385550241454, -6.485486291978119766 ) ) ;
#3786=CARTESIAN_POINT ( 'NONE',  ( 45.86712807150323812, 65.29948385550241596, -5.649768623646098220 ) ) ;
#3791=CARTESIAN_POINT ( 'NONE',  ( 49.97728705011495265, 61.50051614449765935, 7.000000000000000888 ) ) ;
#3793=CARTESIAN_POINT ( 'NONE',  ( 51.92680522751233951, 61.59948385550240602, -6.007379884777223289 ) ) ;
#3795=CARTESIAN_POINT ( 'NONE',  ( 54.09612160359786515, 59.69948385550240033, -5.676469297603166098 ) ) ;
#3802=CARTESIAN_POINT ( 'NONE',  ( 47.70284917648453415, 61.39948385550241738, -6.992620115222774047 ) ) ;
#3814=CARTESIAN_POINT ( 'NONE',  ( 50.02271294988505446, 44.50051614449765935, -7.000000000000000888 ) ) ;
#3838=CARTESIAN_POINT ( 'NONE',  ( 55.11794222512601493, 48.19948385550240744, 3.688883143319541702 ) ) ;
#3840=CARTESIAN_POINT ( 'NONE',  ( 44.03140696652192787, 49.19948385550240033, -4.306917132069425058 ) ) ;
#3841=CARTESIAN_POINT ( 'NONE',  ( 47.70284917648459100, 59.60051614449765367, 6.992620115222796251 ) ) ;
#3849=CARTESIAN_POINT ( 'NONE',  ( 54.09612160359792199, 55.30051614449765651, 5.676469297603124353 ) ) ;
#3851=CARTESIAN_POINT ( 'NONE',  ( 55.32279841668061238, 44.85244137215321558, -4.999999999999997335 ) ) ;
#3856=CARTESIAN_POINT ( 'NONE',  ( 43.34962307344081012, 46.89948385550240317, 2.184720259617164650 ) ) ;
#3859=CARTESIAN_POINT ( 'NONE',  ( 52.57664461997821093, 63.40051614449765083, 8.007379884777206414 ) ) ;
#3861=CARTESIAN_POINT ( 'NONE',  ( 46.49166364869456913, 60.30051614449767072, -4.867452303228181343 ) ) ;
#3873=CARTESIAN_POINT ( 'NONE',  ( 49.97728705011488159, 57.49948385550241170, -7.000000000000000888 ) ) ;
#3878=CARTESIAN_POINT ( 'NONE',  ( 54.72065718078924590, 54.29948385550241596, 6.458785618021043895 ) ) ;
#3881=CARTESIAN_POINT ( 'NONE',  ( 55.08986747509847248, 47.79948385550240886, -3.727524721679197572 ) ) ;
#3885=CARTESIAN_POINT ( 'NONE',  ( 56.79116909180259398, 45.20051614449766220, 4.963592699178938972 ) ) ;
#3887=CARTESIAN_POINT ( 'NONE',  ( 44.91013252490152752, 62.79948385550240175, 3.727524721679198461 ) ) ;
#3897=CARTESIAN_POINT ( 'NONE',  ( 50.02271294988512551, 58.49948385550241170, 7.000000000000000888 ) ) ;
#3908=CARTESIAN_POINT ( 'NONE',  ( 55.96859303347804371, 52.19948385550240033, 4.306917132069425946 ) ) ;
#3910=CARTESIAN_POINT ( 'NONE',  ( 53.50833635130544508, 59.30051614449766362, 4.867452303228181343 ) ) ;
#3919=( NAMED_UNIT ( * ) SI_UNIT ( $, .STERADIAN. ) SOLID_ANGLE_UNIT ( ) );
#3931=CARTESIAN_POINT ( 'NONE',  ( 48.02776887271745210, 65.39948385550239607, -5.992620115222778487 ) ) ;
#3935=CARTESIAN_POINT ( 'NONE',  ( 55.69932041026404335, 49.89948385550241028, -1.875703265242203432 ) ) ;
#3937=CARTESIAN_POINT ( 'NONE',  ( 57.36023556966787851, 47.99948385550239038, -0.02388180880522424582 ) ) ;
#3938=CARTESIAN_POINT ( 'NONE',  ( 52.62207051974829852, 50.60051614449765367, -7.992620115222797139 ) ) ;
#3946=CARTESIAN_POINT ( 'NONE',  ( 44.03140696652198471, 55.80051614449765651, 4.306917132069485454 ) ) ;
#3954=CARTESIAN_POINT ( 'NONE',  ( 50.02271294988512551, 52.49948385550240459, 7.000000000000000888 ) ) ;
#3956=CARTESIAN_POINT ( 'NONE',  ( 42.39856655714566358, 46.89948385550240317, 2.493737253992119207 ) ) ;
#3958=CARTESIAN_POINT ( 'NONE',  ( 56.65037692655921120, 51.10051614449766078, 2.184720259617097593 ) ) ;
#3961=ORIENTED_EDGE ( 'NONE', *, *, #14283, .F. ) ;
#3969=CARTESIAN_POINT ( 'NONE',  ( 45.86712807150323812, 57.29948385550240175, -5.649768623646098220 ) ) ;
#3973=CARTESIAN_POINT ( 'NONE',  ( 47.37792948025162332, 57.39948385550241028, -7.992620115222770494 ) ) ;
#3976=CARTESIAN_POINT ( 'NONE',  ( 51.92680522751233951, 49.59948385550241312, -6.007379884777223289 ) ) ;
#3979=CARTESIAN_POINT ( 'NONE',  ( 50.02271294988505446, 46.50051614449766646, -8.000000000000001776 ) ) ;
#3980=CARTESIAN_POINT ( 'NONE',  ( 50.02271294988511841, 64.49948385550239038, 6.000000000000000888 ) ) ;
#3990=CARTESIAN_POINT ( 'NONE',  ( 45.86712807150323812, 57.29948385550240175, -5.649768623646098220 ) ) ;
#4001=CARTESIAN_POINT ( 'NONE',  ( 55.94051828345050836, 49.79948385550240175, -4.345558710429104465 ) ) ;
#4004=CARTESIAN_POINT ( 'NONE',  ( 52.29715082351538769, 46.60051614449766078, -6.992620115222796251 ) ) ;
#4027=CARTESIAN_POINT ( 'NONE',  ( 55.69932041026405045, 51.10051614449766078, 1.875703265242156359 ) ) ;
#4030=CARTESIAN_POINT ( 'NONE',  ( 55.71335778527780747, 52.09948385550241312, 1.832500667257165983 ) ) ;
#4033=CARTESIAN_POINT ( 'NONE',  ( 50.02271294988512551, 46.49948385550240459, 7.000000000000000888 ) ) ;
#4034=CARTESIAN_POINT ( 'NONE',  ( 58.41169779390614281, 47.00051614449766646, 0.02388180880515032231 ) ) ;
#4044=CARTESIAN_POINT ( 'NONE',  ( 43.34962307344078880, 54.10051614449766788, -2.184720259617096705 ) ) ;
#4053=CARTESIAN_POINT ( 'NONE',  ( 43.34962307344081012, 52.89948385550240317, 2.184720259617164650 ) ) ;
#4055=CARTESIAN_POINT ( 'NONE',  ( 52.62207051974839089, 46.39948385550240317, 7.992620115222770494 ) ) ;
#4057=CARTESIAN_POINT ( 'NONE',  ( 45.86712807150329496, 45.70051614449766220, 5.649768623646139964 ) ) ;
#4058=CARTESIAN_POINT ( 'NONE',  ( 49.99999999999997158, 45.00000000000001421, -7.499999999999998224 ) ) ;
#4069=CARTESIAN_POINT ( 'NONE',  ( 54.13287192849676188, 60.29948385550240886, 5.649768623646098220 ) ) ;
#4074=CARTESIAN_POINT ( 'NONE',  ( 52.57664461997811856, 61.59948385550240602, -8.007379884777229506 ) ) ;
#4077=CARTESIAN_POINT ( 'NONE',  ( 51.92680522751233951, 47.59948385550239891, -6.007379884777223289 ) ) ;
#4080=CARTESIAN_POINT ( 'NONE',  ( 45.90387839640208512, 64.30051614449766362, -5.676469297603124353 ) ) ;
#4082=CARTESIAN_POINT ( 'NONE',  ( 48.07319477248762496, 46.40051614449765793, -6.007379884777208190 ) ) ;
#4090=CARTESIAN_POINT ( 'NONE',  ( 47.70284917648453415, 57.39948385550241028, -6.992620115222774047 ) ) ;
#4101=CARTESIAN_POINT ( 'NONE',  ( 44.05948171654949874, 48.79948385550238754, 4.345558710429105354 ) ) ;
#4104=CARTESIAN_POINT ( 'NONE',  ( 56.66441430157294690, 50.90051614449766504, -2.141517661632166281 ) ) ;
#4123=CARTESIAN_POINT ( 'NONE',  ( 43.69122665457040000, 52.00051614449766646, -0.02388180880515696977 ) ) ;
#4128=CARTESIAN_POINT ( 'NONE',  ( 44.91013252490152752, 50.79948385550240175, 3.727524721679198461 ) ) ;
#4130=CARTESIAN_POINT ( 'NONE',  ( 57.36023556966787851, 45.99948385550238328, -0.02388180880522424582 ) ) ;
#4131=CARTESIAN_POINT ( 'NONE',  ( 49.97728705011495265, 45.50051614449766646, 8.000000000000001776 ) ) ;
#4151=CARTESIAN_POINT ( 'NONE',  ( 54.13287192849676188, 54.29948385550240886, 5.649768623646098220 ) ) ;
#4154=CARTESIAN_POINT ( 'NONE',  ( 43.20883090819742023, 64.20051614449766930, -4.963592699178938972 ) ) ;
#4156=CARTESIAN_POINT ( 'NONE',  ( 43.33558569842706021, 45.90051614449765793, 2.141517661632167169 ) ) ;
#4168=CARTESIAN_POINT ( 'NONE',  ( 52.62207051974839089, 56.39948385550241028, 7.992620115222770494 ) ) ;
#4170=CARTESIAN_POINT ( 'NONE',  ( 51.97223112728254790, 48.39948385550240317, 5.992620115222778487 ) ) ;
#4174=CARTESIAN_POINT ( 'NONE',  ( 42.39856655714564226, 48.10051614449766078, -2.493737253992044156 ) ) ;
#4175=CARTESIAN_POINT ( 'NONE',  ( 46.49166364869456913, 46.30051614449766362, -4.867452303228181343 ) ) ;
#4183=CARTESIAN_POINT ( 'NONE',  ( 47.74827507625478518, 56.59948385550238470, 7.007379884777227730 ) ) ;
#4194=CARTESIAN_POINT ( 'NONE',  ( 52.29715082351547295, 52.39948385550241738, 6.992620115222774047 ) ) ;
#4196=CARTESIAN_POINT ( 'NONE',  ( 42.63976443033212860, 46.00051614449766646, -0.02388180880514948964 ) ) ;
#4214=CARTESIAN_POINT ( 'NONE',  ( 46.49166364869456913, 48.30051614449765651, -4.867452303228181343 ) ) ;
#4217=CARTESIAN_POINT ( 'NONE',  ( 56.30877334542961421, 47.99948385550239038, -0.02388180880520959434 ) ) ;
#4219=CARTESIAN_POINT ( 'NONE',  ( 47.70284917648453415, 53.39948385550238186, -6.992620115222774047 ) ) ;
#4220=CARTESIAN_POINT ( 'NONE',  ( 52.57664461997821093, 49.40051614449766504, 8.007379884777206414 ) ) ;
#4239=CARTESIAN_POINT ( 'NONE',  ( 43.33558569842703179, 55.09948385550241312, -2.141517661632099223 ) ) ;
#4242=CARTESIAN_POINT ( 'NONE',  ( 54.68390685589033495, 45.69948385550240033, -6.485486291978119766 ) ) ;
#4244=CARTESIAN_POINT ( 'NONE',  ( 43.34962307344078880, 48.10051614449766078, -2.184720259617096705 ) ) ;
#4261=CARTESIAN_POINT ( 'NONE',  ( 54.68390685589033495, 59.69948385550240744, -6.485486291978119766 ) ) ;
#4264=CARTESIAN_POINT ( 'NONE',  ( 50.02271294988511841, 58.49948385550241170, 6.000000000000000888 ) ) ;
#4268=CARTESIAN_POINT ( 'NONE',  ( 57.60143344285435774, 47.10051614449766078, 2.493737253992045044 ) ) ;
#4269=CARTESIAN_POINT ( 'NONE',  ( 48.02776887271750184, 51.60051614449766788, 5.992620115222795363 ) ) ;
#4278=CARTESIAN_POINT ( 'NONE',  ( 45.86712807150323812, 63.29948385550240886, -5.649768623646098220 ) ) ;
#4283=CARTESIAN_POINT ( 'NONE',  ( 55.94051828345050836, 45.79948385550240886, -4.345558710429103577 ) ) ;
#4288=CARTESIAN_POINT ( 'NONE',  ( 56.65037692655918988, 51.89948385550241028, -2.184720259617163762 ) ) ;
#4291=CARTESIAN_POINT ( 'NONE',  ( 50.02271294988505446, 48.50051614449765935, -7.000000000000000888 ) ) ;
#4299=EDGE_LOOP ( 'NONE', ( #18336, #9910, #12103 ) ) ;
#4303=CARTESIAN_POINT ( 'NONE',  ( 52.29715082351547295, 48.39948385550240317, 6.992620115222774047 ) ) ;
#4313=CARTESIAN_POINT ( 'NONE',  ( 44.88205777487401349, 47.80051614449764941, 3.688883143319584779 ) ) ;
#4317=CARTESIAN_POINT ( 'NONE',  ( 53.54508667620428497, 60.29948385550240175, 4.840751629271157874 ) ) ;
#4320=CARTESIAN_POINT ( 'NONE',  ( 52.25172492374522903, 49.59948385550240602, -7.007379884777225953 ) ) ;
#4321=CARTESIAN_POINT ( 'NONE',  ( 56.81924384183006538, 44.80051614449766362, -4.924951120819380357 ) ) ;
#4337=CARTESIAN_POINT ( 'NONE',  ( 57.36023556966787851, 53.99948385550239038, -0.02388180880522424582 ) ) ;
#4339=CARTESIAN_POINT ( 'NONE',  ( 47.37792948025162332, 55.39948385550240317, -7.992620115222770494 ) ) ;
#4341=CARTESIAN_POINT ( 'NONE',  ( 55.96859303347802239, 48.80051614449766362, -4.306917132069484566 ) ) ;
#4361=CARTESIAN_POINT ( 'NONE',  ( 55.08986747509847248, 59.79948385550240175, -3.727524721679197572 ) ) ;
#4366=CARTESIAN_POINT ( 'NONE',  ( 42.38452918213190657, 51.90051614449765793, 2.450534656007115508 ) ) ;
#4367=CARTESIAN_POINT ( 'NONE',  ( 50.02271294988506156, 48.50051614449765935, -6.000000000000000888 ) ) ;
#4379=CARTESIAN_POINT ( 'NONE',  ( 43.33558569842703179, 65.09948385550239891, -2.141517661632099223 ) ) ;
#4384=CARTESIAN_POINT ( 'NONE',  ( 50.02271294988512551, 48.49948385550240459, 7.000000000000000888 ) ) ;
#4391=CARTESIAN_POINT ( 'NONE',  ( 45.90387839640214196, 58.69948385550240033, 5.676469297603166098 ) ) ;
#4394=CARTESIAN_POINT ( 'NONE',  ( 56.66441430157294690, 46.90051614449765793, -2.141517661632166281 ) ) ;
#4404=CARTESIAN_POINT ( 'NONE',  ( 55.94051828345050836, 47.79948385550240886, -4.345558710429104465 ) ) ;
#4411=CARTESIAN_POINT ( 'NONE',  ( 47.70284917648459810, 51.60051614449765367, 6.992620115222797139 ) ) ;
#4417=CARTESIAN_POINT ( 'NONE',  ( 50.02271294988506156, 46.50051614449766646, -6.000000000000000888 ) ) ;
#4422=CARTESIAN_POINT ( 'NONE',  ( 44.91013252490152752, 56.79948385550240175, 3.727524721679198461 ) ) ;
#4425=CARTESIAN_POINT ( 'NONE',  ( 54.09612160359786515, 53.69948385550240744, -5.676469297603166098 ) ) ;
#4427=CARTESIAN_POINT ( 'NONE',  ( 57.61547081786810764, 56.90051614449767214, -2.450534656007114176 ) ) ;
#4446=CARTESIAN_POINT ( 'NONE',  ( 50.02271294988512551, 60.49948385550240459, 7.000000000000000888 ) ) ;
#4448=CARTESIAN_POINT ( 'NONE',  ( 54.68390685589033495, 55.69948385550240744, -6.485486291978119766 ) ) ;
#4450=CARTESIAN_POINT ( 'NONE',  ( 47.70284917648459100, 57.60051614449764656, 6.992620115222796251 ) ) ;
#4461=FACE_OUTER_BOUND ( 'NONE', #4299, .T. ) ;
#4465=CARTESIAN_POINT ( 'NONE',  ( 46.45491332379572924, 59.29948385550240886, -4.840751629271157874 ) ) ;
#4468=CARTESIAN_POINT ( 'NONE',  ( 47.42335538002180328, 54.40051614449765793, -8.007379884777206414 ) ) ;
#4469=CARTESIAN_POINT ( 'NONE',  ( 56.30877334542961421, 51.00051614449765935, 0.02388180880515774693 ) ) ;
#4478=CARTESIAN_POINT ( 'NONE',  ( 57.36023556966787851, 61.99948385550241170, -0.02388180880522424582 ) ) ;
#4484=CARTESIAN_POINT ( 'NONE',  ( 44.05948171654949874, 48.79948385550239465, 4.345558710429104465 ) ) ;
#4489=CARTESIAN_POINT ( 'NONE',  ( 54.68390685589033495, 49.69948385550240744, -6.485486291978119766 ) ) ;
#4490=CARTESIAN_POINT ( 'NONE',  ( 49.99999999999997158, 45.00000000000001421, -6.500000000000004441 ) ) ;
#4493=CARTESIAN_POINT ( 'NONE',  ( 50.02271294988512551, 60.49948385550240459, 7.000000000000000888 ) ) ;
#4496=CARTESIAN_POINT ( 'NONE',  ( 56.66441430157294690, 52.90051614449765793, -2.141517661632166281 ) ) ;
#4506=CARTESIAN_POINT ( 'NONE',  ( 43.18075615816989199, 63.19948385550240744, -4.924951120819313743 ) ) ;
#4512=CARTESIAN_POINT ( 'NONE',  ( 45.86712807150329496, 61.70051614449766220, 5.649768623646139964 ) ) ;
#4516=CARTESIAN_POINT ( 'NONE',  ( 48.02776887271750184, 53.60051614449765367, 5.992620115222795363 ) ) ;
#4520=CARTESIAN_POINT ( 'NONE',  ( 44.30067958973596376, 56.89948385550240317, 1.875703265242204099 ) ) ;
#4522=CARTESIAN_POINT ( 'NONE',  ( 52.29715082351547295, 52.39948385550241738, 6.992620115222774047 ) ) ;
#4524=CARTESIAN_POINT ( 'NONE',  ( 41.58830220609386430, 56.00051614449765935, -0.02388180880514929535 ) ) ;
#4535=CARTESIAN_POINT ( 'NONE',  ( 56.65037692655918988, 63.89948385550239607, -2.184720259617163762 ) ) ;
#4539=CARTESIAN_POINT ( 'NONE',  ( 52.25172492374522903, 55.59948385550241312, -7.007379884777225953 ) ) ;
#4541=CARTESIAN_POINT ( 'NONE',  ( 50.02271294988513972, 52.49948385550241170, 8.000000000000001776 ) ) ;
#4543=CARTESIAN_POINT ( 'NONE',  ( 52.25172492374527877, 55.40051614449764372, 7.007379884777203749 ) ) ;
#4554=CARTESIAN_POINT ( 'NONE',  ( 56.66441430157296821, 62.09948385550239891, 2.141517661632100111 ) ) ;
#4561=CARTESIAN_POINT ( 'NONE',  ( 55.71335778527780747, 54.09948385550241312, 1.832500667257165983 ) ) ;
#4564=CARTESIAN_POINT ( 'NONE',  ( 50.02271294988505446, 56.50051614449767357, -8.000000000000001776 ) ) ;
#4566=CARTESIAN_POINT ( 'NONE',  ( 53.54508667620424234, 52.70051614449766220, -4.840751629271188961 ) ) ;
#4574=CARTESIAN_POINT ( 'NONE',  ( 49.97728705011488159, 65.49948385550240459, -7.000000000000000888 ) ) ;
#4579=CARTESIAN_POINT ( 'NONE',  ( 54.13287192849676188, 48.29948385550240175, 5.649768623646098220 ) ) ;
#4583=CARTESIAN_POINT ( 'NONE',  ( 52.62207051974829852, 62.60051614449765367, -7.992620115222797139 ) ) ;
#4584=CARTESIAN_POINT ( 'NONE',  ( 52.60990417590917900, 44.99999999999999289, -5.983956152663589378 ) ) ;
#4585=CARTESIAN_POINT ( 'NONE',  ( 43.33558569842703179, 61.09948385550240602, -2.141517661632099223 ) ) ;
#4588=CARTESIAN_POINT ( 'NONE',  ( 54.09612160359792199, 55.30051614449765651, 5.676469297603124353 ) ) ;
#4597=CARTESIAN_POINT ( 'NONE',  ( 42.39856655714566358, 62.89948385550240317, 2.493737253992119207 ) ) ;
#4603=CARTESIAN_POINT ( 'NONE',  ( 44.05948171654945611, 62.20051614449765509, -4.345558710429044069 ) ) ;
#4609=CARTESIAN_POINT ( 'NONE',  ( 44.28664221472221385, 53.90051614449765793, 1.832500667257213722 ) ) ;
#4615=CARTESIAN_POINT ( 'NONE',  ( 53.50833635130540955, 55.69948385550240744, -4.867452303228209765 ) ) ;
#4617=CARTESIAN_POINT ( 'NONE',  ( 45.31609314410960820, 52.30051614449766362, -6.485486291978072693 ) ) ;
#4619=AXIS2_PLACEMENT_3D ( 'NONE', #3092, #15039, #10322 ) ;
#4632=CARTESIAN_POINT ( 'NONE',  ( 52.29715082351547295, 62.39948385550240317, 6.992620115222774047 ) ) ;
#4638=CARTESIAN_POINT ( 'NONE',  ( 57.36023556966787851, 59.99948385550240459, -0.02388180880522424582 ) ) ;
#4640=CARTESIAN_POINT ( 'NONE',  ( 52.62207051974839089, 56.39948385550241028, 7.992620115222770494 ) ) ;
#4642=CARTESIAN_POINT ( 'NONE',  ( 43.34962307344078880, 54.10051614449766788, -2.184720259617096705 ) ) ;
#4660=CARTESIAN_POINT ( 'NONE',  ( 56.30877334542961421, 55.99948385550241170, -0.02388180880520959434 ) ) ;
#4663=CARTESIAN_POINT ( 'NONE',  ( 54.72065718078918906, 50.70051614449766220, -6.458785618021089192 ) ) ;
#4664=CARTESIAN_POINT ( 'NONE',  ( 56.30877334542961421, 53.00051614449765935, 0.02388180880515774693 ) ) ;
#4666=DIRECTION ( 'NONE',  ( -1.000000000000000000, 0.000000000000000000, 1.224646799147353207E-16 ) ) ;
#4679=CARTESIAN_POINT ( 'NONE',  ( 44.05948171654949874, 46.79948385550240175, 4.345558710429104465 ) ) ;
#4685=CARTESIAN_POINT ( 'NONE',  ( 56.79116909180255135, 47.79948385550240886, -4.963592699179005585 ) ) ;
#4687=CARTESIAN_POINT ( 'NONE',  ( 45.86712807150323812, 57.29948385550240175, -5.649768623646098220 ) ) ;
#4690=CARTESIAN_POINT ( 'NONE',  ( 57.36023556966787851, 55.00051614449765225, 0.02388180880515038476 ) ) ;
#4692=AXIS2_PLACEMENT_3D ( 'NONE', #5847, #70, #6046 ) ;
#4700=CARTESIAN_POINT ( 'NONE',  ( 54.68390685589033495, 63.69948385550240033, -6.485486291978119766 ) ) ;
#4705=CARTESIAN_POINT ( 'NONE',  ( 44.05948171654945611, 56.20051614449765509, -4.345558710429044069 ) ) ;
#4710=CARTESIAN_POINT ( 'NONE',  ( 49.97728705011494554, 57.50051614449766646, 6.000000000000000888 ) ) ;
#4712=CARTESIAN_POINT ( 'NONE',  ( 53.50833635130540955, 59.69948385550240744, -4.867452303228209765 ) ) ;
#4714=CARTESIAN_POINT ( 'NONE',  ( 57.61547081786810764, 54.90051614449765793, -2.450534656007114176 ) ) ;
#4728=CARTESIAN_POINT ( 'NONE',  ( 42.63976443033212149, 60.99948385550239749, 0.02388180880522514787 ) ) ;
#4736=CARTESIAN_POINT ( 'NONE',  ( 42.63976443033212860, 58.99948385550239038, 0.02388180880522514787 ) ) ;
#4739=CARTESIAN_POINT ( 'NONE',  ( 45.31609314410967926, 54.69948385550240033, 6.485486291978119766 ) ) ;
#4741=CARTESIAN_POINT ( 'NONE',  ( 47.70284917648459100, 55.60051614449764656, 6.992620115222796251 ) ) ;
#4751=CARTESIAN_POINT ( 'NONE',  ( 49.97728705011495265, 49.50051614449765935, 7.000000000000000888 ) ) ;
#4757=CARTESIAN_POINT ( 'NONE',  ( 55.71335778527780036, 44.90051614449765793, -1.832500667257213056 ) ) ;
#4761=CARTESIAN_POINT ( 'NONE',  ( 45.27934281921082516, 53.70051614449766220, 6.458785618021089192 ) ) ;
#4762=CARTESIAN_POINT ( 'NONE',  ( 46.49166364869456913, 54.30051614449765651, -4.867452303228181343 ) ) ;
#4773=CARTESIAN_POINT ( 'NONE',  ( 42.63976443033212149, 52.99948385550240459, 0.02388180880522514787 ) ) ;
#4777=CARTESIAN_POINT ( 'NONE',  ( 42.38452918213190657, 63.90051614449765793, 2.450534656007115508 ) ) ;
#4779=CARTESIAN_POINT ( 'NONE',  ( 43.33558569842703179, 57.09948385550240602, -2.141517661632099223 ) ) ;
#4782=CARTESIAN_POINT ( 'NONE',  ( 49.97728705011495265, 53.50051614449765935, 7.000000000000000888 ) ) ;
#4794=CARTESIAN_POINT ( 'NONE',  ( 44.05948171654949874, 54.79948385550241596, 4.345558710429105354 ) ) ;
#4799=CARTESIAN_POINT ( 'NONE',  ( 52.29715082351539479, 58.60051614449766078, -6.992620115222796251 ) ) ;
#4805=CARTESIAN_POINT ( 'NONE',  ( 55.69932041026405045, 53.10051614449767499, 1.875703265242156359 ) ) ;
#4808=CARTESIAN_POINT ( 'NONE',  ( 44.91013252490152752, 64.79948385550240175, 3.727524721679198461 ) ) ;
#4810=CARTESIAN_POINT ( 'NONE',  ( 50.02271294988505446, 56.50051614449767357, -8.000000000000001776 ) ) ;
#4824=CARTESIAN_POINT ( 'NONE',  ( 54.09612160359786515, 55.69948385550240744, -5.676469297603166098 ) ) ;
#4826=CARTESIAN_POINT ( 'NONE',  ( 52.57664461997811856, 61.59948385550240602, -8.007379884777229506 ) ) ;
#4828=CARTESIAN_POINT ( 'NONE',  ( 50.02271294988505446, 56.50051614449766646, -7.000000000000000888 ) ) ;
#4835=CARTESIAN_POINT ( 'NONE',  ( 56.66441430157294690, 46.90051614449765793, -2.141517661632166281 ) ) ;
#4840=ORIENTED_EDGE ( 'NONE', *, *, #14283, .T. ) ;
#4843=CARTESIAN_POINT ( 'NONE',  ( 51.92680522751238925, 45.40051614449765793, 6.007379884777208190 ) ) ;
#4846=CARTESIAN_POINT ( 'NONE',  ( 54.68390685589039890, 61.30051614449766362, 6.485486291978072693 ) ) ;
#4849=CARTESIAN_POINT ( 'NONE',  ( 44.30067958973594955, 56.10051614449766078, -1.875703265242155693 ) ) ;
#4864=CARTESIAN_POINT ( 'NONE',  ( 47.74827507625477807, 54.59948385550239891, 7.007379884777229506 ) ) ;
#4869=CARTESIAN_POINT ( 'NONE',  ( 42.38452918213188525, 47.09948385550240602, -2.450534656007040013 ) ) ;
#4872=CARTESIAN_POINT ( 'NONE',  ( 44.30067958973596376, 46.89948385550240317, 1.875703265242204099 ) ) ;
#4875=CARTESIAN_POINT ( 'NONE',  ( 47.70284917648459100, 61.60051614449764656, 6.992620115222796251 ) ) ;
#4877=CARTESIAN_POINT ( 'NONE',  ( 42.63976443033212860, 52.99948385550240459, 0.02388180880522514787 ) ) ;
#4880=EDGE_LOOP ( 'NONE', ( #12199, #3184 ) ) ;
#4884=CARTESIAN_POINT ( 'NONE',  ( 52.25172492374522903, 49.59948385550240602, -7.007379884777225953 ) ) ;
#4895=CARTESIAN_POINT ( 'NONE',  ( 53.50833635130544508, 53.30051614449767072, 4.867452303228181343 ) ) ;
#4900=CARTESIAN_POINT ( 'NONE',  ( 57.61547081786810764, 60.90051614449766504, -2.450534656007114176 ) ) ;
#4914=CARTESIAN_POINT ( 'NONE',  ( 56.65037692655918988, 63.89948385550239607, -2.184720259617163762 ) ) ;
#4917=CARTESIAN_POINT ( 'NONE',  ( 47.37792948025162332, 59.39948385550240317, -7.992620115222770494 ) ) ;
#4918=CARTESIAN_POINT ( 'NONE',  ( 45.90387839640208512, 62.30051614449766362, -5.676469297603124353 ) ) ;
#4925=CARTESIAN_POINT ( 'NONE',  ( 49.97728705011495265, 47.50051614449766646, 7.000000000000000888 ) ) ;
#4926=CARTESIAN_POINT ( 'NONE',  ( 45.90387839640214196, 62.69948385550240744, 5.676469297603166098 ) ) ;
#4931=CARTESIAN_POINT ( 'NONE',  ( 46.45491332379572924, 63.29948385550240175, -4.840751629271157874 ) ) ;
#4935=CARTESIAN_POINT ( 'NONE',  ( 54.72065718078918906, 56.70051614449766930, -6.458785618021089192 ) ) ;
#4936=CARTESIAN_POINT ( 'NONE',  ( 51.97223112728249816, 54.60051614449766788, -5.992620115222793586 ) ) ;
#4948=CARTESIAN_POINT ( 'NONE',  ( 47.70284917648453415, 55.39948385550239607, -6.992620115222774047 ) ) ;
#4953=CARTESIAN_POINT ( 'NONE',  ( 57.61547081786812896, 56.09948385550240602, 2.450534656007040901 ) ) ;
#4955=CARTESIAN_POINT ( 'NONE',  ( 55.94051828345050836, 63.79948385550240886, -4.345558710429104465 ) ) ;
#4958=CARTESIAN_POINT ( 'NONE',  ( 49.97728705011495265, 59.50051614449765935, 7.000000000000000888 ) ) ;
#4962=CARTESIAN_POINT ( 'NONE',  ( 55.96859303347804371, 60.19948385550240744, 4.306917132069425946 ) ) ;
#4969=CARTESIAN_POINT ( 'NONE',  ( 43.33558569842703179, 51.09948385550240602, -2.141517661632099223 ) ) ;
#4977=CARTESIAN_POINT ( 'NONE',  ( 49.97728705011495265, 63.50051614449765935, 7.000000000000000888 ) ) ;
#4984=CARTESIAN_POINT ( 'NONE',  ( 50.02271294988506156, 58.50051614449765225, -6.000000000000000888 ) ) ;
#4988=CARTESIAN_POINT ( 'NONE',  ( 43.18075615816994173, 57.80051614449766362, 4.924951120819380357 ) ) ;
#5008=CARTESIAN_POINT ( 'NONE',  ( 45.86712807150323812, 63.29948385550240886, -5.649768623646098220 ) ) ;
#5010=CARTESIAN_POINT ( 'NONE',  ( 52.57664461997811856, 59.59948385550240602, -8.007379884777229506 ) ) ;
#5011=CARTESIAN_POINT ( 'NONE',  ( 54.09612160359792199, 59.30051614449766362, 5.676469297603124353 ) ) ;
#5024=CARTESIAN_POINT ( 'NONE',  ( 55.94051828345054389, 47.20051614449766220, 4.345558710429044957 ) ) ;
#5031=CARTESIAN_POINT ( 'NONE',  ( 46.49166364869460466, 62.69948385550240744, 4.867452303228209765 ) ) ;
#5035=CARTESIAN_POINT ( 'NONE',  ( 43.20883090819742023, 62.20051614449766220, -4.963592699178938972 ) ) ;
#5037=CARTESIAN_POINT ( 'NONE',  ( 49.97728705011494554, 61.50051614449766646, 6.000000000000000888 ) ) ;
#5049=CARTESIAN_POINT ( 'NONE',  ( 45.86712807150323812, 53.29948385550240886, -5.649768623646098220 ) ) ;
#5054=CARTESIAN_POINT ( 'NONE',  ( 42.38452918213188525, 51.09948385550240602, -2.450534656007040013 ) ) ;
#5056=CARTESIAN_POINT ( 'NONE',  ( 43.33558569842703179, 63.09948385550240602, -2.141517661632099223 ) ) ;
#5059=CARTESIAN_POINT ( 'NONE',  ( 45.86712807150329496, 59.70051614449766220, 5.649768623646139964 ) ) ;
#5060=CARTESIAN_POINT ( 'NONE',  ( 44.05948171654949874, 56.79948385550240886, 4.345558710429105354 ) ) ;
#5069=CARTESIAN_POINT ( 'NONE',  ( 57.36023556966787851, 51.99948385550238328, -0.02388180880522424582 ) ) ;
#5078=CARTESIAN_POINT ( 'NONE',  ( 43.33558569842706021, 63.90051614449765793, 2.141517661632167169 ) ) ;
#5081=CARTESIAN_POINT ( 'NONE',  ( 55.94051828345050836, 47.79948385550240886, -4.345558710429104465 ) ) ;
#5085=CARTESIAN_POINT ( 'NONE',  ( 55.69932041026405045, 59.10051614449766078, 1.875703265242156359 ) ) ;
#5087=( LENGTH_UNIT ( ) NAMED_UNIT ( * ) SI_UNIT ( .MILLI., .METRE. ) );
#5090=CARTESIAN_POINT ( 'NONE',  ( 57.60143344285435774, 57.10051614449766788, 2.493737253992045044 ) ) ;
#5107=CARTESIAN_POINT ( 'NONE',  ( 55.11794222512601493, 46.19948385550240744, 3.688883143319541702 ) ) ;
#5109=CARTESIAN_POINT ( 'NONE',  ( 56.81924384183011512, 58.19948385550240744, 4.924951120819313743 ) ) ;
#5110=CARTESIAN_POINT ( 'NONE',  ( 55.94051828345053679, 63.20051614449765509, 4.345558710429044069 ) ) ;
#5116=CARTESIAN_POINT ( 'NONE',  ( 54.13287192849671214, 48.70051614449766220, -5.649768623646139964 ) ) ;
#5117=CARTESIAN_POINT ( 'NONE',  ( 54.76112626223286384, 45.00000000000007816, -5.734953493745535091 ) ) ;
#5126=CARTESIAN_POINT ( 'NONE',  ( 57.60143344285435774, 61.10051614449766788, 2.493737253992045044 ) ) ;
#5128=CARTESIAN_POINT ( 'NONE',  ( 48.02776887271750184, 59.60051614449765367, 5.992620115222795363 ) ) ;
#5140=CARTESIAN_POINT ( 'NONE',  ( 54.13287192849676188, 50.29948385550240175, 5.649768623646098220 ) ) ;
#5144=CARTESIAN_POINT ( 'NONE',  ( 50.02271294988513972, 52.49948385550241170, 8.000000000000001776 ) ) ;
#5147=CARTESIAN_POINT ( 'NONE',  ( 43.34962307344081012, 64.89948385550239607, 2.184720259617164650 ) ) ;
#5150=CARTESIAN_POINT ( 'NONE',  ( 56.66441430157294690, 58.90051614449766504, -2.141517661632166281 ) ) ;
#5151=CARTESIAN_POINT ( 'NONE',  ( 55.11794222512601493, 62.19948385550240744, 3.688883143319541702 ) ) ;
#5152=CARTESIAN_POINT ( 'NONE',  ( 47.70284917648453415, 57.39948385550241028, -6.992620115222774047 ) ) ;
#5160=CARTESIAN_POINT ( 'NONE',  ( 55.96859303347804371, 52.19948385550240033, 4.306917132069425946 ) ) ;
#5171=CARTESIAN_POINT ( 'NONE',  ( 48.02776887271750184, 61.60051614449765367, 5.992620115222795363 ) ) ;
#5176=CARTESIAN_POINT ( 'NONE',  ( 49.97728705011495265, 57.50051614449766646, 8.000000000000001776 ) ) ;
#5185=DIRECTION ( 'NONE',  ( -1.000000000000000000, 0.000000000000000000, 1.224646799147353207E-16 ) ) ;
#5197=CARTESIAN_POINT ( 'NONE',  ( 43.33558569842703179, 65.09948385550239891, -2.141517661632099223 ) ) ;
#5199=CARTESIAN_POINT ( 'NONE',  ( 45.27934281921075410, 63.29948385550240175, -6.458785618021043895 ) ) ;
#5200=CARTESIAN_POINT ( 'NONE',  ( 55.94051828345053679, 59.20051614449766220, 4.345558710429044069 ) ) ;
#5208=CARTESIAN_POINT ( 'NONE',  ( 56.65037692655921120, 51.10051614449766078, 2.184720259617097593 ) ) ;
#5213=CARTESIAN_POINT ( 'NONE',  ( 55.11928596558036020, 44.77036257738321012, -5.000000000000000888 ) ) ;
#5218=DIRECTION ( 'NONE',  ( -0.04542589977017699732, 0.9989677110047501252, 0.000000000000000000 ) ) ;
#5221=CARTESIAN_POINT ( 'NONE',  ( 57.60143344285435774, 59.10051614449766078, 2.493737253992045044 ) ) ;
#5222=CARTESIAN_POINT ( 'NONE',  ( 55.71335778527780036, 60.90051614449766504, -1.832500667257213056 ) ) ;
#5236=CARTESIAN_POINT ( 'NONE',  ( 43.34962307344081012, 56.89948385550240317, 2.184720259617164650 ) ) ;
#5242=CARTESIAN_POINT ( 'NONE',  ( 41.58830220609386430, 54.99948385550239749, 0.02388180880523263147 ) ) ;
#5245=CARTESIAN_POINT ( 'NONE',  ( 53.54508667620428497, 46.29948385550240886, 4.840751629271157874 ) ) ;
#5249=CARTESIAN_POINT ( 'NONE',  ( 57.36023556966787851, 59.00051614449765935, 0.02388180880515038476 ) ) ;
#5250=CARTESIAN_POINT ( 'NONE',  ( 48.07319477248768180, 64.59948385550241312, 6.007379884777225953 ) ) ;
#5251=CARTESIAN_POINT ( 'NONE',  ( 47.70284917648453415, 59.39948385550241028, -6.992620115222774047 ) ) ;
#5261=CARTESIAN_POINT ( 'NONE',  ( 52.29715082351547295, 60.39948385550239607, 6.992620115222774047 ) ) ;
#5268=CARTESIAN_POINT ( 'NONE',  ( 54.09612160359792199, 63.30051614449766362, 5.676469297603124353 ) ) ;
#5270=CARTESIAN_POINT ( 'NONE',  ( 44.03140696652192787, 47.19948385550240744, -4.306917132069425058 ) ) ;
#5272=CARTESIAN_POINT ( 'NONE',  ( 55.11794222512599362, 62.80051614449766362, -3.688883143319583446 ) ) ;
#5293=CARTESIAN_POINT ( 'NONE',  ( 51.92680522751233951, 49.59948385550241312, -6.007379884777223289 ) ) ;
#5295=CARTESIAN_POINT ( 'NONE',  ( 50.02271294988512551, 48.49948385550240459, 7.000000000000000888 ) ) ;
#5297=CARTESIAN_POINT ( 'NONE',  ( 52.25172492374527877, 59.40051614449765083, 7.007379884777203749 ) ) ;
#5308=CARTESIAN_POINT ( 'NONE',  ( 52.29715082351539479, 50.60051614449766078, -6.992620115222796251 ) ) ;
#5321=CARTESIAN_POINT ( 'NONE',  ( 56.81924384183011512, 48.19948385550240744, 4.924951120819313743 ) ) ;
#5323=CARTESIAN_POINT ( 'NONE',  ( 53.50833635130544508, 59.30051614449766362, 4.867452303228181343 ) ) ;
#5341=CARTESIAN_POINT ( 'NONE',  ( 55.96859303347805081, 58.19948385550240744, 4.306917132069425058 ) ) ;
#5345=CARTESIAN_POINT ( 'NONE',  ( 42.39856655714566358, 50.89948385550240317, 2.493737253992119207 ) ) ;
#5348=CARTESIAN_POINT ( 'NONE',  ( 50.02271294988511841, 52.49948385550241170, 6.000000000000000888 ) ) ;
#5353=CARTESIAN_POINT ( 'NONE',  ( 45.31609314410960820, 46.30051614449766362, -6.485486291978072693 ) ) ;
#5354=CARTESIAN_POINT ( 'NONE',  ( 56.30877334542961421, 45.00051614449765225, 0.02388180880515774693 ) ) ;
#5361=CARTESIAN_POINT ( 'NONE',  ( 54.13287192849676188, 56.29948385550240175, 5.649768623646098220 ) ) ;
#5371=CARTESIAN_POINT ( 'NONE',  ( 43.33558569842703179, 53.09948385550240602, -2.141517661632099223 ) ) ;
#5373=CARTESIAN_POINT ( 'NONE',  ( 48.07319477248762496, 62.40051614449765793, -6.007379884777208190 ) ) ;
#5384=( LENGTH_UNIT ( ) NAMED_UNIT ( * ) SI_UNIT ( .MILLI., .METRE. ) );
#5392=CARTESIAN_POINT ( 'NONE',  ( 46.45491332379572924, 65.29948385550241596, -4.840751629271157874 ) ) ;
#5395=CARTESIAN_POINT ( 'NONE',  ( 44.28664221472220675, 51.09948385550240602, -1.832500667257165317 ) ) ;
#5397=CARTESIAN_POINT ( 'NONE',  ( 43.18075615816989199, 65.19948385550240744, -4.924951120819313743 ) ) ;
#5398=CARTESIAN_POINT ( 'NONE',  ( 47.42335538002180328, 50.40051614449766504, -8.007379884777206414 ) ) ;
#5402=( BOUNDED_CURVE ( )  B_SPLINE_CURVE ( 2, ( #3015, #13202, #10441, #4283, #11820, #16250, #12108, #2826, #18117, #8976, #13393, #14665, #17925, #4679, #18018, #16351, #8881, #10639, #14863, #19313, #14961, #19216, #11721, #14763, #1345, #7319, #13295, #5851, #4579, #17825, #4384, #10348, #1442, #4484, #1538, #10535, #15065, #1732, #15346, #3491, #3213, #360, #1826, #8077, #14053, #3300, #6234, #13955, #5140, #15154, #10735, #9175, #3581, #12397, #18502, #15537, #2115, #17027, #7698, #6333, #13676, #7893, #16828, #254, #11111, #18601, #12489, #1929, #539, #13866, #3391, #12207, #16927, #9257, #18220, #4773, #9353, #6613, #5049, #15440, #16735, #6511, #15246, #7794, #2020, #636, #13773, #7982, #12305, #12592, #18308, #4864, #10826, #9456, #446, #11020, #9545, #6418, #18406, #4948, #10921, #5428, #12791, #931, #3779, #9641, #9932, #14347, #18792, #18692, #15932, #11404, #17410, #9742, #5236, #6902, #12890, #1035, #3969, #6707, #3873, #8269, #2518, #14248, #832, #11313, #9832, #5341, #8368, #3676, #17317, #15833, #2417, #15737, #8474, #12690, #18893, #11211, #17217, #14454, #6803, #6998, #12977, #18985, #2316, #5524, #11499, #17509, #4069, #17119, #15638, #2220, #8178, #14151, #734, #4728, #13637, #18172, #7657, #3257, #7465, #10692, #1690, #11973, #13731, #12264, #16594, #212, #1593, #4632, #23, #15303, #13446, #9217, #14916, #13827, #6192, #6011, #10880, #17977, #16886, #3351, #9130, #12164, #4535, #18265, #10494, #6372, #10592, #16498, #3070, #16693, #15207, #6099, #12068, #7755, #119, #18070, #13546, #407, #12352 ),
 .UNSPECIFIED., .F., .F. ) 
 B_SPLINE_CURVE_WITH_KNOTS ( ( 3, 2, 2, 2, 2, 2, 2, 2, 2, 2, 2, 2, 2, 2, 2, 2, 2, 2, 2, 2, 2, 2, 2, 2, 2, 2, 2, 2, 2, 2, 2, 2, 2, 2, 2, 2, 2, 2, 2, 2, 2, 2, 2, 2, 2, 2, 2, 2, 2, 2, 2, 2, 2, 2, 2, 2, 2, 2, 2, 2, 2, 2, 2, 2, 2, 2, 2, 2, 2, 2, 2, 2, 2, 2, 2, 2, 2, 2, 2, 2, 2, 2, 2, 2, 2, 2, 2, 2, 2, 2, 2, 2, 2, 2, 2, 2, 2, 2, 2, 2, 3 ),
 ( 0.000000000000000000, 0.01000000000000000021, 0.02000000000000000042, 0.02999999999999999889, 0.04000000000000000083, 0.05000000000000000278, 0.05999999999999999778, 0.07000000000000000666, 0.08000000000000000167, 0.08999999999999999667, 0.1000000000000000056, 0.1100000000000000006, 0.1199999999999999956, 0.1300000000000000044, 0.1400000000000000133, 0.1499999999999999944, 0.1600000000000000033, 0.1700000000000000122, 0.1799999999999999933, 0.1900000000000000022, 0.2000000000000000111, 0.2099999999999999922, 0.2200000000000000011, 0.2300000000000000100, 0.2399999999999999911, 0.2500000000000000000, 0.2600000000000000089, 0.2700000000000000178, 0.2800000000000000266, 0.2899999999999999800, 0.2999999999999999889, 0.3099999999999999978, 0.3200000000000000067, 0.3300000000000000155, 0.3400000000000000244, 0.3499999999999999778, 0.3599999999999999867, 0.3699999999999999956, 0.3800000000000000044, 0.3900000000000000133, 0.4000000000000000222, 0.4099999999999999756, 0.4199999999999999845, 0.4299999999999999933, 0.4400000000000000022, 0.4500000000000000111, 0.4600000000000000200, 0.4699999999999999734, 0.4799999999999999822, 0.4899999999999999911, 0.5000000000000000000, 0.5100000000000000089, 0.5200000000000000178, 0.5300000000000000266, 0.5400000000000000355, 0.5500000000000000444, 0.5600000000000000533, 0.5699999999999999512, 0.5799999999999999600, 0.5899999999999999689, 0.5999999999999999778, 0.6099999999999999867, 0.6199999999999999956, 0.6300000000000000044, 0.6400000000000000133, 0.6500000000000000222, 0.6600000000000000311, 0.6700000000000000400, 0.6800000000000000488, 0.6899999999999999467, 0.6999999999999999556, 0.7099999999999999645, 0.7199999999999999734, 0.7299999999999999822, 0.7399999999999999911, 0.7500000000000000000, 0.7600000000000000089, 0.7700000000000000178, 0.7800000000000000266, 0.7900000000000000355, 0.8000000000000000444, 0.8100000000000000533, 0.8199999999999999512, 0.8299999999999999600, 0.8399999999999999689, 0.8499999999999999778, 0.8599999999999999867, 0.8699999999999999956, 0.8800000000000000044, 0.8900000000000000133, 0.9000000000000000222, 0.9100000000000000311, 0.9200000000000000400, 0.9300000000000000488, 0.9399999999999999467, 0.9499999999999999556, 0.9599999999999999645, 0.9699999999999999734, 0.9799999999999999822, 0.9899999999999999911, 1.000000000000000000 ),
 .UNSPECIFIED. ) 
 CURVE ( )  GEOMETRIC_REPRESENTATION_ITEM ( )  RATIONAL_B_SPLINE_CURVE ( ( 1.000000000000000000, 0.9510565162951535312, 1.000000000000000000, 0.9510565162951535312, 1.000000000000000000, 0.9510565162951535312, 1.000000000000000000, 0.9510565162951535312, 1.000000000000000000, 0.9510565162951535312, 1.000000000000000000, 0.9510565162951535312, 1.000000000000000000, 0.9510565162951535312, 1.000000000000000000, 0.9510565162951535312, 1.000000000000000000, 0.9510565162951535312, 1.000000000000000000, 0.9510565162951535312, 1.000000000000000000, 0.9510565162951535312, 1.000000000000000000, 0.9510565162951535312, 1.000000000000000000, 0.9510565162951535312, 1.000000000000000000, 0.9510565162951535312, 1.000000000000000000, 0.9510565162951535312, 1.000000000000000000, 0.9510565162951535312, 1.000000000000000000, 0.9510565162951535312, 1.000000000000000000, 0.9510565162951535312, 1.000000000000000000, 0.9510565162951535312, 1.000000000000000000, 0.9510565162951535312, 1.000000000000000000, 0.9510565162951535312, 1.000000000000000000, 0.9510565162951535312, 1.000000000000000000, 0.9510565162951535312, 1.000000000000000000, 0.9510565162951535312, 1.000000000000000000, 0.9510565162951535312, 1.000000000000000000, 0.9510565162951535312, 1.000000000000000000, 0.9510565162951535312, 1.000000000000000000, 0.9510565162951535312, 1.000000000000000000, 0.9510565162951535312, 1.000000000000000000, 0.9510565162951535312, 1.000000000000000000, 0.9510565162951535312, 1.000000000000000000, 0.9510565162951535312, 1.000000000000000000, 0.9510565162951535312, 1.000000000000000000, 0.9510565162951535312, 1.000000000000000000, 0.9510565162951535312, 1.000000000000000000, 0.9510565162951535312, 1.000000000000000000, 0.9510565162951535312, 1.000000000000000000, 0.9510565162951535312, 1.000000000000000000, 0.9510565162951535312, 1.000000000000000000, 0.9510565162951535312, 1.000000000000000000, 0.9510565162951535312, 1.000000000000000000, 0.9510565162951535312, 1.000000000000000000, 0.9510565162951535312, 1.000000000000000000, 0.9510565162951535312, 1.000000000000000000, 0.9510565162951535312, 1.000000000000000000, 0.9510565162951535312, 1.000000000000000000, 0.9510565162951535312, 1.000000000000000000, 0.9510565162951535312, 1.000000000000000000, 0.9510565162951535312, 1.000000000000000000, 0.9510565162951535312, 1.000000000000000000, 0.9510565162951535312, 1.000000000000000000, 0.9510565162951535312, 1.000000000000000000, 0.9510565162951535312, 1.000000000000000000, 0.9510565162951535312, 1.000000000000000000, 0.9510565162951535312, 1.000000000000000000, 0.9510565162951535312, 1.000000000000000000, 0.9510565162951535312, 1.000000000000000000, 0.9510565162951535312, 1.000000000000000000, 0.9510565162951535312, 1.000000000000000000, 0.9510565162951535312, 1.000000000000000000, 0.9510565162951535312, 1.000000000000000000, 0.9510565162951535312, 1.000000000000000000, 0.9510565162951535312, 1.000000000000000000, 0.9510565162951535312, 1.000000000000000000, 0.9510565162951535312, 1.000000000000000000, 0.9510565162951535312, 1.000000000000000000, 0.9510565162951535312, 1.000000000000000000, 0.9510565162951535312, 1.000000000000000000, 0.9510565162951535312, 1.000000000000000000, 0.9510565162951535312, 1.000000000000000000, 0.9510565162951535312, 1.000000000000000000, 0.9510565162951535312, 1.000000000000000000, 0.9510565162951535312, 1.000000000000000000, 0.9510565162951535312, 1.000000000000000000, 0.9510565162951535312, 1.000000000000000000, 0.9510565162951535312, 1.000000000000000000, 0.9510565162951535312, 1.000000000000000000, 0.9510565162951535312, 1.000000000000000000, 0.9510565162951535312, 1.000000000000000000, 0.9510565162951535312, 1.000000000000000000, 0.9510565162951535312, 1.000000000000000000, 0.9510565162951535312, 1.000000000000000000, 0.9510565162951535312, 1.000000000000000000, 0.9510565162951535312, 1.000000000000000000, 0.9510565162951535312, 1.000000000000000000, 0.9510565162951535312, 1.000000000000000000, 0.9510565162951535312, 1.000000000000000000, 0.9510565162951535312, 1.000000000000000000, 0.9510565162951535312, 1.000000000000000000, 0.9510565162951535312, 1.000000000000000000, 0.9510565162951535312, 1.000000000000000000, 0.9510565162951535312, 1.000000000000000000, 0.9510565162951535312, 1.000000000000000000, 0.9510565162951535312, 1.000000000000000000, 0.9510565162951535312, 1.000000000000000000, 0.9510565162951535312, 1.000000000000000000, 0.9510565162951535312, 1.000000000000000000, 0.9510565162951535312, 1.000000000000000000, 0.9510565162951535312, 1.000000000000000000, 0.9510565162951535312, 1.000000000000000000 ) ) 
 REPRESENTATION_ITEM ( '' )  );
#5405=CARTESIAN_POINT ( 'NONE',  ( 47.70284917648459810, 55.60051614449765367, 6.992620115222797139 ) ) ;
#5413=CARTESIAN_POINT ( 'NONE',  ( 45.86712807150323812, 53.29948385550240886, -5.649768623646098220 ) ) ;
#5415=CARTESIAN_POINT ( 'NONE',  ( 47.42335538002180328, 64.40051614449764372, -8.007379884777206414 ) ) ;
#5417=CARTESIAN_POINT ( 'NONE',  ( 44.28664221472221385, 61.90051614449766504, 1.832500667257213722 ) ) ;
#5428=CARTESIAN_POINT ( 'NONE',  ( 52.25172492374522903, 55.59948385550241312, -7.007379884777227730 ) ) ;
#5432=CARTESIAN_POINT ( 'NONE',  ( 43.20883090819745576, 60.79948385550241596, 4.963592699179006473 ) ) ;
#5435=CARTESIAN_POINT ( 'NONE',  ( 49.97728705011488870, 53.49948385550240459, -6.000000000000000888 ) ) ;
#5440=CARTESIAN_POINT ( 'NONE',  ( 58.41169779390614281, 45.00051614449765225, 0.02388180880515032231 ) ) ;
#5442=CARTESIAN_POINT ( 'NONE',  ( 48.07319477248768180, 62.59948385550238470, 6.007379884777225953 ) ) ;
#5453=CARTESIAN_POINT ( 'NONE',  ( 45.86712807150323812, 59.29948385550240175, -5.649768623646098220 ) ) ;
#5462=CARTESIAN_POINT ( 'NONE',  ( 44.05948171654949874, 54.79948385550241596, 4.345558710429105354 ) ) ;
#5464=CARTESIAN_POINT ( 'NONE',  ( 55.96859303347802239, 44.80051614449767072, -4.306917132069484566 ) ) ;
#5486=CARTESIAN_POINT ( 'NONE',  ( 44.28664221472221385, 45.90051614449766504, 1.832500667257213722 ) ) ;
#5490=CARTESIAN_POINT ( 'NONE',  ( 48.07319477248768180, 52.59948385550240602, 6.007379884777225953 ) ) ;
#5492=CARTESIAN_POINT ( 'NONE',  ( 45.27934281921075410, 65.29948385550241596, -6.458785618021043895 ) ) ;
#5493=CARTESIAN_POINT ( 'NONE',  ( 54.72065718078918906, 46.70051614449766220, -6.458785618021089192 ) ) ;
#5502=CARTESIAN_POINT ( 'NONE',  ( 47.74827507625470702, 52.40051614449765083, -7.007379884777204637 ) ) ;
#5509=CARTESIAN_POINT ( 'NONE',  ( 56.66441430157296821, 52.09948385550240602, 2.141517661632100111 ) ) ;
#5511=CARTESIAN_POINT ( 'NONE',  ( 57.60143344285435774, 63.10051614449766078, 2.493737253992045044 ) ) ;
#5513=CARTESIAN_POINT ( 'NONE',  ( 44.05948171654945611, 50.20051614449764088, -4.345558710429044069 ) ) ;
#5524=CARTESIAN_POINT ( 'NONE',  ( 57.36023556966787851, 59.99948385550240459, -0.02388180880522424582 ) ) ;
#5528=CARTESIAN_POINT ( 'NONE',  ( 43.18075615816989199, 61.19948385550241454, -4.924951120819313743 ) ) ;
#5532=CARTESIAN_POINT ( 'NONE',  ( 44.28664221472220675, 49.09948385550241312, -1.832500667257165317 ) ) ;
#5535=CARTESIAN_POINT ( 'NONE',  ( 42.39856655714564226, 50.10051614449766078, -2.493737253992044156 ) ) ;
#5536=CARTESIAN_POINT ( 'NONE',  ( 50.02271294988506156, 46.50051614449766646, -6.000000000000000888 ) ) ;
#5546=CARTESIAN_POINT ( 'NONE',  ( 55.96859303347804371, 56.19948385550241454, 4.306917132069425946 ) ) ;
#5561=CARTESIAN_POINT ( 'NONE',  ( 47.74827507625478518, 48.59948385550239180, 7.007379884777227730 ) ) ;
#5563=CARTESIAN_POINT ( 'NONE',  ( 56.65037692655921120, 47.10051614449766078, 2.184720259617097593 ) ) ;
#5587=CARTESIAN_POINT ( 'NONE',  ( 46.45491332379576477, 51.70051614449765509, 4.840751629271188961 ) ) ;
#5590=CARTESIAN_POINT ( 'NONE',  ( 55.08986747509847248, 49.79948385550240175, -3.727524721679197572 ) ) ;
#5593=CARTESIAN_POINT ( 'NONE',  ( 41.58830220609386430, 64.99948385550240459, 0.02388180880523263147 ) ) ;
#5594=CARTESIAN_POINT ( 'NONE',  ( 54.68390685589039890, 49.30051614449766362, 6.485486291978072693 ) ) ;
#5605=CARTESIAN_POINT ( 'NONE',  ( 42.63976443033212149, 52.00051614449765935, -0.02388180880514948964 ) ) ;
#5612=CARTESIAN_POINT ( 'NONE',  ( 47.70284917648453415, 51.39948385550238896, -6.992620115222774047 ) ) ;
#5614=CARTESIAN_POINT ( 'NONE',  ( 45.31609314410967926, 48.69948385550241454, 6.485486291978119766 ) ) ;
#5616=CARTESIAN_POINT ( 'NONE',  ( 54.13287192849671214, 48.70051614449766220, -5.649768623646139964 ) ) ;
#5632=CARTESIAN_POINT ( 'NONE',  ( 45.27934281921075410, 59.29948385550240886, -6.458785618021043895 ) ) ;
#5634=CARTESIAN_POINT ( 'NONE',  ( 46.49166364869460466, 48.69948385550241454, 4.867452303228209765 ) ) ;
#5637=CARTESIAN_POINT ( 'NONE',  ( 47.42335538002180328, 48.40051614449766504, -8.007379884777206414 ) ) ;
#5639=CARTESIAN_POINT ( 'NONE',  ( 55.71335778527780036, 46.90051614449766504, -1.832500667257213056 ) ) ;
#5649=CARTESIAN_POINT ( 'NONE',  ( 52.29715082351547295, 56.39948385550238896, 6.992620115222774047 ) ) ;
#5662=CARTESIAN_POINT ( 'NONE',  ( 56.66441430157296821, 50.09948385550240602, 2.141517661632100111 ) ) ;
#5665=CARTESIAN_POINT ( 'NONE',  ( 56.66441430157294690, 48.90051614449766504, -2.141517661632166281 ) ) ;
#5689=CARTESIAN_POINT ( 'NONE',  ( 46.49166364869456913, 50.30051614449766362, -4.867452303228181343 ) ) ;
#5695=CARTESIAN_POINT ( 'NONE',  ( 56.30877334542961421, 51.99948385550239749, -0.02388180880520959434 ) ) ;
#5697=CARTESIAN_POINT ( 'NONE',  ( 55.96859303347804371, 52.19948385550240033, 4.306917132069425946 ) ) ;
#5698=CARTESIAN_POINT ( 'NONE',  ( 57.61547081786810764, 48.90051614449766504, -2.450534656007114176 ) ) ;
#5716=CARTESIAN_POINT ( 'NONE',  ( 42.63976443033212860, 50.99948385550240459, 0.02388180880522514787 ) ) ;
#5719=CARTESIAN_POINT ( 'NONE',  ( 57.61547081786812896, 50.09948385550240602, 2.450534656007040901 ) ) ;
#5721=CARTESIAN_POINT ( 'NONE',  ( 55.94051828345053679, 45.20051614449764088, 4.345558710429044069 ) ) ;
#5735=CARTESIAN_POINT ( 'NONE',  ( 47.42335538002188144, 60.59948385550240602, 8.007379884777233059 ) ) ;
#5738=CARTESIAN_POINT ( 'NONE',  ( 53.50833635130540955, 51.69948385550241454, -4.867452303228209765 ) ) ;
#5741=CARTESIAN_POINT ( 'NONE',  ( 41.58830220609386430, 50.00051614449765935, -0.02388180880514929535 ) ) ;
#5742=CARTESIAN_POINT ( 'NONE',  ( 49.97728705011494554, 51.50051614449765935, 6.000000000000000888 ) ) ;
#5761=CARTESIAN_POINT ( 'NONE',  ( 45.86712807150323812, 49.29948385550240175, -5.649768623646098220 ) ) ;
#5763=CARTESIAN_POINT ( 'NONE',  ( 55.94051828345053679, 45.20051614449764088, 4.345558710429044069 ) ) ;
#5785=CARTESIAN_POINT ( 'NONE',  ( 55.11794222512599362, 48.80051614449767072, -3.688883143319583446 ) ) ;
#5787=CARTESIAN_POINT ( 'NONE',  ( 49.97728705011488870, 57.49948385550241170, -6.000000000000000888 ) ) ;
#5789=CARTESIAN_POINT ( 'NONE',  ( 45.86712807150323812, 51.29948385550240175, -5.649768623646098220 ) ) ;
#5790=CARTESIAN_POINT ( 'NONE',  ( 41.58830220609386430, 50.00051614449765935, -0.02388180880514929535 ) ) ;
#5809=CARTESIAN_POINT ( 'NONE',  ( 45.90387839640214196, 50.69948385550240744, 5.676469297603166098 ) ) ;
#5811=CARTESIAN_POINT ( 'NONE',  ( 47.42335538002188144, 54.59948385550240602, 8.007379884777233059 ) ) ;
#5813=CARTESIAN_POINT ( 'NONE',  ( 50.02271294988505446, 50.50051614449765935, -7.000000000000000888 ) ) ;
#5824=ORIENTED_EDGE ( 'NONE', *, *, #17008, .T. ) ;
#5829=CARTESIAN_POINT ( 'NONE',  ( 47.37792948025162332, 61.39948385550240317, -7.992620115222770494 ) ) ;
#5832=CARTESIAN_POINT ( 'NONE',  ( 48.02776887271745210, 59.39948385550240317, -5.992620115222778487 ) ) ;
#5835=CARTESIAN_POINT ( 'NONE',  ( 52.57664461997821093, 53.40051614449765793, 8.007379884777206414 ) ) ;
#5836=CARTESIAN_POINT ( 'NONE',  ( 44.88205777487401349, 47.80051614449764941, 3.688883143319584779 ) ) ;
#5846=CARTESIAN_POINT ( 'NONE',  ( 43.34962307344081012, 64.89948385550239607, 2.184720259617164650 ) ) ;
#5847=CARTESIAN_POINT ( 'NONE',  ( 50.02271294988505446, 64.50051614449765225, -7.000000000000000888 ) ) ;
#5851=CARTESIAN_POINT ( 'NONE',  ( 55.96859303347805081, 48.19948385550240744, 4.306917132069425058 ) ) ;
#5858=CARTESIAN_POINT ( 'NONE',  ( 57.36023556966787851, 57.99948385550239038, -0.02388180880522424582 ) ) ;
#5861=CARTESIAN_POINT ( 'NONE',  ( 43.33558569842706021, 45.90051614449765793, 2.141517661632167169 ) ) ;
#5873=CARTESIAN_POINT ( 'NONE',  ( 42.38452918213188525, 65.09948385550239891, -2.450534656007040013 ) ) ;
#5883=CARTESIAN_POINT ( 'NONE',  ( 46.45491332379576477, 45.70051614449766220, 4.840751629271188961 ) ) ;
#5886=CARTESIAN_POINT ( 'NONE',  ( 46.45491332379572924, 57.29948385550240175, -4.840751629271157874 ) ) ;
#5889=CARTESIAN_POINT ( 'NONE',  ( 55.94051828345050836, 55.79948385550238044, -4.345558710429104465 ) ) ;
#5890=CARTESIAN_POINT ( 'NONE',  ( 52.62207051974829852, 56.60051614449765367, -7.992620115222797139 ) ) ;
#5904=CARTESIAN_POINT ( 'NONE',  ( 44.03140696652192787, 59.19948385550238612, -4.306917132069425058 ) ) ;
#5906=CARTESIAN_POINT ( 'NONE',  ( 52.57664461997811856, 53.59948385550240602, -8.007379884777229506 ) ) ;
#5910=CARTESIAN_POINT ( 'NONE',  ( 50.02271294988505446, 54.50051614449765935, -7.000000000000000888 ) ) ;
#5934=CARTESIAN_POINT ( 'NONE',  ( 53.54508667620428497, 56.29948385550240886, 4.840751629271157874 ) ) ;
#5936=CARTESIAN_POINT ( 'NONE',  ( 47.37792948025170858, 55.60051614449765367, 7.992620115222797139 ) ) ;
#5938=CARTESIAN_POINT ( 'NONE',  ( 55.08986747509849380, 49.20051614449766220, 3.727524721679155384 ) ) ;
#5957=CARTESIAN_POINT ( 'NONE',  ( 58.41169779390614281, 63.00051614449766646, 0.02388180880515032231 ) ) ;
#5960=CARTESIAN_POINT ( 'NONE',  ( 54.13287192849676188, 60.29948385550240886, 5.649768623646098220 ) ) ;
#5963=CARTESIAN_POINT ( 'NONE',  ( 44.03140696652198471, 53.80051614449766362, 4.306917132069485454 ) ) ;
#5974=CARTESIAN_POINT ( 'NONE',  ( 50.02271294988513972, 64.49948385550239038, 8.000000000000001776 ) ) ;
#5982=CARTESIAN_POINT ( 'NONE',  ( 54.13287192849671214, 60.70051614449766220, -5.649768623646139964 ) ) ;
#5988=CARTESIAN_POINT ( 'NONE',  ( 55.69932041026405045, 55.10051614449765367, 1.875703265242156359 ) ) ;
#5993=CARTESIAN_POINT ( 'NONE',  ( 51.92680522751233951, 55.59948385550240602, -6.007379884777223289 ) ) ;
#5996=CIRCLE ( 'NONE', #39, 0.4999999999999972244 ) ;
#5997=CARTESIAN_POINT ( 'NONE',  ( 49.97728705011488159, 51.49948385550240459, -7.000000000000000888 ) ) ;
#5999=CARTESIAN_POINT ( 'NONE',  ( 56.79116909180259398, 53.20051614449766220, 4.963592699178938972 ) ) ;
#6011=CARTESIAN_POINT ( 'NONE',  ( 44.03140696652193498, 63.19948385550240744, -4.306917132069424170 ) ) ;
#6015=CARTESIAN_POINT ( 'NONE',  ( 43.34962307344081012, 58.89948385550241028, 2.184720259617164650 ) ) ;
#6017=CARTESIAN_POINT ( 'NONE',  ( 42.38452918213188525, 51.09948385550240602, -2.450534656007040013 ) ) ;
#6019=CARTESIAN_POINT ( 'NONE',  ( 49.97728705011495265, 55.50051614449766646, 7.000000000000000888 ) ) ;
#6033=CARTESIAN_POINT ( 'NONE',  ( 56.30877334542961421, 59.99948385550241170, -0.02388180880520959434 ) ) ;
#6036=CARTESIAN_POINT ( 'NONE',  ( 52.62207051974829852, 50.60051614449765367, -7.992620115222797139 ) ) ;
#6037=CARTESIAN_POINT ( 'NONE',  ( 55.11794222512599362, 58.80051614449766362, -3.688883143319583446 ) ) ;
#6045=CARTESIAN_POINT ( 'NONE',  ( 47.70284917648453415, 65.39948385550239607, -6.992620115222774047 ) ) ;
#6046=DIRECTION ( 'NONE',  ( 0.04542589977017006536, -0.9989677110047503472, 0.000000000000000000 ) ) ;
#6055=CARTESIAN_POINT ( 'NONE',  ( 43.20883090819745576, 46.79948385550240886, 4.963592699179006473 ) ) ;
#6056=CARTESIAN_POINT ( 'NONE',  ( 51.88965917396063077, 45.00000000000000711, -6.239765512074564313 ) ) ;
#6057=CARTESIAN_POINT ( 'NONE',  ( 54.13287192849676188, 58.29948385550240175, 5.649768623646098220 ) ) ;
#6060=CARTESIAN_POINT ( 'NONE',  ( 44.03140696652198471, 55.80051614449766362, 4.306917132069485454 ) ) ;
#6072=CARTESIAN_POINT ( 'NONE',  ( 45.90387839640214196, 46.69948385550240744, 5.676469297603166098 ) ) ;
#6077=CARTESIAN_POINT ( 'NONE',  ( 43.34962307344078880, 62.10051614449766078, -2.184720259617096705 ) ) ;
#6081=CARTESIAN_POINT ( 'NONE',  ( 48.07319477248762496, 54.40051614449765793, -6.007379884777208190 ) ) ;
#6084=CARTESIAN_POINT ( 'NONE',  ( 51.97223112728254790, 58.39948385550241028, 5.992620115222778487 ) ) ;
#6087=CARTESIAN_POINT ( 'NONE',  ( 42.39856655714564226, 52.10051614449766788, -2.493737253992044156 ) ) ;
#6099=CARTESIAN_POINT ( 'NONE',  ( 44.05948171654949874, 64.79948385550240175, 4.345558710429104465 ) ) ;
#6103=CARTESIAN_POINT ( 'NONE',  ( 49.97728705011488159, 59.49948385550240459, -7.000000000000000888 ) ) ;
#6105=CARTESIAN_POINT ( 'NONE',  ( 42.38452918213188525, 55.09948385550241312, -2.450534656007040013 ) ) ;
#6107=CARTESIAN_POINT ( 'NONE',  ( 54.09612160359792199, 55.30051614449765651, 5.676469297603124353 ) ) ;
#6117=CARTESIAN_POINT ( 'NONE',  ( 54.13287192849676188, 62.29948385550240886, 5.649768623646098220 ) ) ;
#6122=CARTESIAN_POINT ( 'NONE',  ( 51.97223112728254790, 54.39948385550241028, 5.992620115222778487 ) ) ;
#6125=CARTESIAN_POINT ( 'NONE',  ( 43.18075615816994173, 51.80051614449766362, 4.924951120819380357 ) ) ;
#6127=CARTESIAN_POINT ( 'NONE',  ( 44.28664221472221385, 53.90051614449765793, 1.832500667257213722 ) ) ;
#6133=CARTESIAN_POINT ( 'NONE',  ( 45.86712807150323812, 65.29948385550241596, -5.649768623646098220 ) ) ;
#6142=CARTESIAN_POINT ( 'NONE',  ( 47.42335538002188144, 48.59948385550239891, 8.007379884777233059 ) ) ;
#6144=CARTESIAN_POINT ( 'NONE',  ( 42.63976443033212860, 56.99948385550241170, 0.02388180880522514787 ) ) ;
#6147=CARTESIAN_POINT ( 'NONE',  ( 57.36023556966787851, 57.00051614449766646, 0.02388180880515038476 ) ) ;
#6158=CARTESIAN_POINT ( 'NONE',  ( 52.25172492374522903, 45.59948385550240602, -7.007379884777225953 ) ) ;
#6166=CARTESIAN_POINT ( 'NONE',  ( 44.05948171654945611, 60.20051614449765509, -4.345558710429044069 ) ) ;
#6173=CARTESIAN_POINT ( 'NONE',  ( 56.30877334542961421, 57.00051614449766646, 0.02388180880515774693 ) ) ;
#6177=CARTESIAN_POINT ( 'NONE',  ( 48.02776887271745210, 57.39948385550241028, -5.992620115222778487 ) ) ;
#6180=CARTESIAN_POINT ( 'NONE',  ( 57.61547081786810764, 50.90051614449765793, -2.450534656007114176 ) ) ;
#6192=CARTESIAN_POINT ( 'NONE',  ( 43.33558569842703179, 63.09948385550240602, -2.141517661632099223 ) ) ;
#6197=CARTESIAN_POINT ( 'NONE',  ( 45.90387839640214196, 56.69948385550240744, 5.676469297603166098 ) ) ;
#6199=CARTESIAN_POINT ( 'NONE',  ( 56.79116909180255135, 55.79948385550239465, -4.963592699179005585 ) ) ;
#6201=CARTESIAN_POINT ( 'NONE',  ( 52.29715082351538769, 54.60051614449766788, -6.992620115222796251 ) ) ;
#6208=CARTESIAN_POINT ( 'NONE',  ( 56.65037692655921120, 49.10051614449766078, 2.184720259617097593 ) ) ;
#6209=CARTESIAN_POINT ( 'NONE',  ( 45.90387839640214196, 64.69948385550240744, 5.676469297603166098 ) ) ;
#6217=CARTESIAN_POINT ( 'NONE',  ( 48.02776887271745210, 57.39948385550241028, -5.992620115222778487 ) ) ;
#6220=CARTESIAN_POINT ( 'NONE',  ( 43.18075615816994173, 55.80051614449766362, 4.924951120819380357 ) ) ;
#6222=CARTESIAN_POINT ( 'NONE',  ( 51.92680522751238925, 55.40051614449767214, 6.007379884777208190 ) ) ;
#6234=CARTESIAN_POINT ( 'NONE',  ( 56.66441430157296821, 50.09948385550240602, 2.141517661632100111 ) ) ;
#6239=CARTESIAN_POINT ( 'NONE',  ( 45.31609314410967926, 46.69948385550240744, 6.485486291978119766 ) ) ;
#6241=CARTESIAN_POINT ( 'NONE',  ( 49.97728705011488159, 59.49948385550240459, -7.000000000000000888 ) ) ;
#6243=CARTESIAN_POINT ( 'NONE',  ( 52.25172492374527877, 57.40051614449765083, 7.007379884777203749 ) ) ;
#6253=CARTESIAN_POINT ( 'NONE',  ( 49.97728705011488159, 51.49948385550240459, -7.000000000000000888 ) ) ;
#6259=CARTESIAN_POINT ( 'NONE',  ( 57.36023556966787851, 61.00051614449765935, 0.02388180880515038476 ) ) ;
#6265=CARTESIAN_POINT ( 'NONE',  ( 51.97223112728249816, 52.60051614449765367, -5.992620115222793586 ) ) ;
#6268=CARTESIAN_POINT ( 'NONE',  ( 55.11794222512601493, 64.19948385550240744, 3.688883143319541702 ) ) ;
#6271=CARTESIAN_POINT ( 'NONE',  ( 45.27934281921082516, 51.70051614449765509, 6.458785618021089192 ) ) ;
#6296=CARTESIAN_POINT ( 'NONE',  ( 43.33558569842703179, 57.09948385550240602, -2.141517661632099223 ) ) ;
#6299=CARTESIAN_POINT ( 'NONE',  ( 56.79116909180255135, 59.79948385550240175, -4.963592699179005585 ) ) ;
#6300=CARTESIAN_POINT ( 'NONE',  ( 56.65037692655921120, 53.10051614449766078, 2.184720259617097593 ) ) ;
#6310=CARTESIAN_POINT ( 'NONE',  ( 49.97728705011495265, 45.50051614449765935, 7.000000000000000888 ) ) ;
#6311=CARTESIAN_POINT ( 'NONE',  ( 52.29715082351547295, 64.39948385550239607, 6.992620115222774047 ) ) ;
#6316=CARTESIAN_POINT ( 'NONE',  ( 55.69932041026405045, 45.10051614449766788, 1.875703265242156359 ) ) ;
#6320=CARTESIAN_POINT ( 'NONE',  ( 54.72065718078918906, 58.70051614449765509, -6.458785618021089192 ) ) ;
#6321=CARTESIAN_POINT ( 'NONE',  ( 49.97728705011494554, 55.50051614449766646, 6.000000000000000888 ) ) ;
#6323=PLANE ( 'NONE',  #8810 ) ;
#6333=CARTESIAN_POINT ( 'NONE',  ( 47.70284917648453415, 51.39948385550240317, -6.992620115222774047 ) ) ;
#6337=CARTESIAN_POINT ( 'NONE',  ( 42.39856655714566358, 46.89948385550240317, 2.493737253992119207 ) ) ;
#6339=CARTESIAN_POINT ( 'NONE',  ( 51.92680522751233951, 45.59948385550240602, -6.007379884777223289 ) ) ;
#6341=CARTESIAN_POINT ( 'NONE',  ( 45.86712807150329496, 53.70051614449766220, 5.649768623646139964 ) ) ;
#6344=CARTESIAN_POINT ( 'NONE',  ( 55.94051828345050836, 53.79948385550238754, -4.345558710429104465 ) ) ;
#6349=CARTESIAN_POINT ( 'NONE',  ( 54.09612160359786515, 49.69948385550240744, -5.676469297603166098 ) ) ;
#6354=CARTESIAN_POINT ( 'NONE',  ( 43.34962307344078880, 60.10051614449766078, -2.184720259617096705 ) ) ;
#6357=UNCERTAINTY_MEASURE_WITH_UNIT (LENGTH_MEASURE( 1.000000000000000082E-05 ), #5384, 'distance_accuracy_value', 'NONE');
#6359=CARTESIAN_POINT ( 'NONE',  ( 44.88205777487401349, 55.80051614449766362, 3.688883143319584779 ) ) ;
#6362=CARTESIAN_POINT ( 'NONE',  ( 49.97728705011494554, 45.50051614449766646, 6.000000000000000888 ) ) ;
#6364=CARTESIAN_POINT ( 'NONE',  ( 57.60143344285435774, 59.10051614449766078, 2.493737253992045044 ) ) ;
#6372=CARTESIAN_POINT ( 'NONE',  ( 55.96859303347805081, 64.19948385550239323, 4.306917132069425058 ) ) ;
#6377=CARTESIAN_POINT ( 'NONE',  ( 57.36023556966787851, 63.99948385550241881, -0.02388180880522424582 ) ) ;
#6380=CARTESIAN_POINT ( 'NONE',  ( 52.62207051974839089, 62.39948385550240317, 7.992620115222770494 ) ) ;
#6381=CARTESIAN_POINT ( 'NONE',  ( 50.02271294988505446, 62.50051614449766646, -7.000000000000000888 ) ) ;
#6391=CARTESIAN_POINT ( 'NONE',  ( 56.66441430157294690, 44.90051614449765793, -2.141517661632166281 ) ) ;
#6394=CARTESIAN_POINT ( 'NONE',  ( 43.34962307344081012, 62.89948385550241028, 2.184720259617164650 ) ) ;
#6399=CARTESIAN_POINT ( 'NONE',  ( 44.88205777487398507, 63.19948385550240744, -3.688883143319540814 ) ) ;
#6402=CARTESIAN_POINT ( 'NONE',  ( 57.60143344285435774, 57.10051614449766788, 2.493737253992045044 ) ) ;
#6404=CARTESIAN_POINT ( 'NONE',  ( 44.28664221472221385, 57.90051614449765793, 1.832500667257213722 ) ) ;
#6412=CARTESIAN_POINT ( 'NONE',  ( 54.77701766759913227, 44.74161735293615294, -5.000000000000010658 ) ) ;
#6418=CARTESIAN_POINT ( 'NONE',  ( 44.03140696652193498, 55.19948385550240744, -4.306917132069424170 ) ) ;
#6419=B_SPLINE_CURVE_WITH_KNOTS ( 'NONE', 3,
 ( #8550, #18964, #5213, #3851, #8450, #2598 ),
 .UNSPECIFIED., .F., .F.,
 ( 4, 2, 4 ),
 ( 0.0007315534878134838555, 0.001060812114463466869, 0.001390070741113449884 ),
 .UNSPECIFIED. ) ;
#6423=CARTESIAN_POINT ( 'NONE',  ( 57.60143344285433642, 55.89948385550241028, -2.493737253992118319 ) ) ;
#6426=CARTESIAN_POINT ( 'NONE',  ( 42.63976443033212860, 62.99948385550241170, 0.02388180880522514787 ) ) ;
#6429=CARTESIAN_POINT ( 'NONE',  ( 45.90387839640208512, 58.30051614449766362, -5.676469297603124353 ) ) ;
#6431=CARTESIAN_POINT ( 'NONE',  ( 52.29715082351547295, 58.39948385550238896, 6.992620115222774047 ) ) ;
#6438=CARTESIAN_POINT ( 'NONE',  ( 43.34962307344081012, 52.89948385550240317, 2.184720259617164650 ) ) ;
#6448=CARTESIAN_POINT ( 'NONE',  ( 56.30877334542961421, 63.00051614449766646, 0.02388180880515774693 ) ) ;
#6453=CARTESIAN_POINT ( 'NONE',  ( 42.39856655714564226, 60.10051614449766788, -2.493737253992044156 ) ) ;
#6472=CARTESIAN_POINT ( 'NONE',  ( 50.02271294988512551, 64.49948385550240459, 7.000000000000000888 ) ) ;
#6475=CARTESIAN_POINT ( 'NONE',  ( 45.31609314410967926, 60.69948385550240033, 6.485486291978119766 ) ) ;
#6476=CARTESIAN_POINT ( 'NONE',  ( 42.63976443033212860, 62.00051614449764514, -0.02388180880514948964 ) ) ;
#6483=CARTESIAN_POINT ( 'NONE',  ( 57.36023556966787851, 45.00051614449765225, 0.02388180880515038476 ) ) ;
#6490=CARTESIAN_POINT ( 'NONE',  ( 56.30877334542961421, 61.99948385550241170, -0.02388180880520959434 ) ) ;
#6491=CARTESIAN_POINT ( 'NONE',  ( 49.99999999999997158, 45.00000000000003553, -7.000000000000000888 ) ) ;
#6492=CARTESIAN_POINT ( 'NONE',  ( 42.63976443033212860, 46.99948385550240459, 0.02388180880522514787 ) ) ;
#6495=CARTESIAN_POINT ( 'NONE',  ( 42.39856655714564226, 62.10051614449765367, -2.493737253992044156 ) ) ;
#6496=CARTESIAN_POINT ( 'NONE',  ( 56.66441430157294690, 44.90051614449765793, -2.141517661632166281 ) ) ;
#6511=CARTESIAN_POINT ( 'NONE',  ( 52.25172492374522903, 53.59948385550241312, -7.007379884777227730 ) ) ;
#6516=CARTESIAN_POINT ( 'NONE',  ( 52.62207051974839089, 50.39948385550241738, 7.992620115222770494 ) ) ;
#6519=CARTESIAN_POINT ( 'NONE',  ( 43.33558569842703179, 65.09948385550239891, -2.141517661632099223 ) ) ;
#6523=CARTESIAN_POINT ( 'NONE',  ( 54.13287192849671214, 62.70051614449766220, -5.649768623646139964 ) ) ;
#6525=CARTESIAN_POINT ( 'NONE',  ( 44.03140696652192787, 61.19948385550239323, -4.306917132069425058 ) ) ;
#6532=CARTESIAN_POINT ( 'NONE',  ( 52.25172492374522903, 51.59948385550240602, -7.007379884777225953 ) ) ;
#6547=CARTESIAN_POINT ( 'NONE',  ( 44.30067958973594955, 60.10051614449766788, -1.875703265242155693 ) ) ;
#6551=CARTESIAN_POINT ( 'NONE',  ( 42.38452918213190657, 57.90051614449765793, 2.450534656007115508 ) ) ;
#6571=CARTESIAN_POINT ( 'NONE',  ( 42.63976443033212860, 62.99948385550241170, 0.02388180880522514787 ) ) ;
#6574=CARTESIAN_POINT ( 'NONE',  ( 56.81924384183011512, 60.19948385550240744, 4.924951120819313743 ) ) ;
#6575=CARTESIAN_POINT ( 'NONE',  ( 54.13287192849671214, 58.70051614449765509, -5.649768623646139964 ) ) ;
#6586=CARTESIAN_POINT ( 'NONE',  ( 52.29715082351539479, 46.60051614449766078, -6.992620115222796251 ) ) ;
#6593=CARTESIAN_POINT ( 'NONE',  ( 53.54508667620428497, 64.29948385550240175, 4.840751629271157874 ) ) ;
#6597=CARTESIAN_POINT ( 'NONE',  ( 52.57664461997821093, 61.40051614449765793, 8.007379884777206414 ) ) ;
#6599=CARTESIAN_POINT ( 'NONE',  ( 51.92680522751238925, 61.40051614449765793, 6.007379884777208190 ) ) ;
#6613=CARTESIAN_POINT ( 'NONE',  ( 44.03140696652193498, 53.19948385550240033, -4.306917132069424170 ) ) ;
#6618=CARTESIAN_POINT ( 'NONE',  ( 54.68390685589033495, 53.69948385550240744, -6.485486291978119766 ) ) ;
#6621=CARTESIAN_POINT ( 'NONE',  ( 55.94051828345050836, 61.79948385550239465, -4.345558710429104465 ) ) ;
#6625=CARTESIAN_POINT ( 'NONE',  ( 47.74827507625469281, 60.40051614449767214, -7.007379884777203749 ) ) ;
#6627=CARTESIAN_POINT ( 'NONE',  ( 44.03140696652192787, 57.19948385550238612, -4.306917132069425058 ) ) ;
#6634=CARTESIAN_POINT ( 'NONE',  ( 44.05948171654949874, 52.79948385550240175, 4.345558710429105354 ) ) ;
#6642=CARTESIAN_POINT ( 'NONE',  ( 50.02271294988505446, 64.50051614449765225, -7.000000000000000888 ) ) ;
#6649=CARTESIAN_POINT ( 'NONE',  ( 44.30067958973594955, 62.10051614449765367, -1.875703265242155693 ) ) ;
#6654=CARTESIAN_POINT ( 'NONE',  ( 54.68390685589039890, 57.30051614449767072, 6.485486291978072693 ) ) ;
#6671=CARTESIAN_POINT ( 'NONE',  ( 49.97728705011488159, 63.49948385550241170, -7.000000000000000888 ) ) ;
#6673=CARTESIAN_POINT ( 'NONE',  ( 54.72065718078924590, 58.29948385550240886, 6.458785618021043895 ) ) ;
#6674=CARTESIAN_POINT ( 'NONE',  ( 44.03140696652198471, 63.80051614449765651, 4.306917132069485454 ) ) ;
#6683=CARTESIAN_POINT ( 'NONE',  ( 44.05948171654945611, 54.20051614449765509, -4.345558710429044069 ) ) ;
#6692=CARTESIAN_POINT ( 'NONE',  ( 50.02271294988505446, 58.50051614449765225, -8.000000000000001776 ) ) ;
#6693=CARTESIAN_POINT ( 'NONE',  ( 44.30067958973594955, 60.10051614449766788, -1.875703265242155693 ) ) ;
#6707=CARTESIAN_POINT ( 'NONE',  ( 47.70284917648453415, 57.39948385550240317, -6.992620115222774047 ) ) ;
#6711=CARTESIAN_POINT ( 'NONE',  ( 45.31609314410967926, 54.69948385550240033, 6.485486291978119766 ) ) ;
#6714=CARTESIAN_POINT ( 'NONE',  ( 47.70284917648453415, 61.39948385550241738, -6.992620115222774047 ) ) ;
#6717=CARTESIAN_POINT ( 'NONE',  ( 56.65037692655921120, 59.10051614449766078, 2.184720259617097593 ) ) ;
#6718=CARTESIAN_POINT ( 'NONE',  ( 44.91013252490152752, 60.79948385550241596, 3.727524721679198461 ) ) ;
#6719=CARTESIAN_POINT ( 'NONE',  ( 52.29715082351547295, 56.39948385550238896, 6.992620115222774047 ) ) ;
#6727=CARTESIAN_POINT ( 'NONE',  ( 55.94051828345050836, 59.79948385550238754, -4.345558710429104465 ) ) ;
#6735=CARTESIAN_POINT ( 'NONE',  ( 43.34962307344081012, 46.89948385550240317, 2.184720259617164650 ) ) ;
#6737=CARTESIAN_POINT ( 'NONE',  ( 56.30877334542961421, 59.00051614449766646, 0.02388180880515774693 ) ) ;
#6767=CARTESIAN_POINT ( 'NONE',  ( 44.03140696652192787, 65.19948385550240744, -4.306917132069425058 ) ) ;
#6769=CARTESIAN_POINT ( 'NONE',  ( 54.72065718078924590, 64.29948385550240175, 6.458785618021043895 ) ) ;
#6770=CARTESIAN_POINT ( 'NONE',  ( 47.70284917648459100, 61.60051614449764656, 6.992620115222796251 ) ) ;
#6779=CARTESIAN_POINT ( 'NONE',  ( 45.90387839640208512, 52.30051614449766362, -5.676469297603124353 ) ) ;
#6789=CARTESIAN_POINT ( 'NONE',  ( 45.27934281921075410, 47.29948385550241596, -6.458785618021043895 ) ) ;
#6790=CARTESIAN_POINT ( 'NONE',  ( 43.69122665457040000, 64.00051614449765225, -0.02388180880515696977 ) ) ;
#6803=CARTESIAN_POINT ( 'NONE',  ( 49.97728705011488159, 59.49948385550240459, -7.000000000000000888 ) ) ;
#6809=CARTESIAN_POINT ( 'NONE',  ( 49.97728705011486738, 55.49948385550241170, -8.000000000000001776 ) ) ;
#6813=CARTESIAN_POINT ( 'NONE',  ( 55.11794222512601493, 50.19948385550241454, 3.688883143319541702 ) ) ;
#6817=CARTESIAN_POINT ( 'NONE',  ( 50.02271294988505446, 62.50051614449766646, -7.000000000000000888 ) ) ;
#6818=CARTESIAN_POINT ( 'NONE',  ( 55.08986747509847248, 61.79948385550240175, -3.727524721679197572 ) ) ;
#6826=CARTESIAN_POINT ( 'NONE',  ( 55.96859303347804371, 60.19948385550240744, 4.306917132069425946 ) ) ;
#6832=( GEOMETRIC_REPRESENTATION_CONTEXT ( 3 ) GLOBAL_UNCERTAINTY_ASSIGNED_CONTEXT ( ( #1467 ) ) GLOBAL_UNIT_ASSIGNED_CONTEXT ( ( #8121, #18933, #12637 ) ) REPRESENTATION_CONTEXT ( 'NONE', 'WORKASPACE' ) );
#6835=CARTESIAN_POINT ( 'NONE',  ( 45.90387839640214196, 48.69948385550240744, 5.676469297603166098 ) ) ;
#6837=CARTESIAN_POINT ( 'NONE',  ( 55.11794222512599362, 58.80051614449766362, -3.688883143319583446 ) ) ;
#6845=FILL_AREA_STYLE ('',( #3620 ) ) ;
#6857=CARTESIAN_POINT ( 'NONE',  ( 55.71335778527780747, 48.09948385550240602, 1.832500667257165983 ) ) ;
#6859=CARTESIAN_POINT ( 'NONE',  ( 56.65037692655918988, 47.89948385550240317, -2.184720259617163762 ) ) ;
#6861=CARTESIAN_POINT ( 'NONE',  ( 42.38452918213190657, 49.90051614449766504, 2.450534656007115508 ) ) ;
#6872=CARTESIAN_POINT ( 'NONE',  ( 56.66441430157294690, 52.90051614449765793, -2.141517661632166281 ) ) ;
#6881=CARTESIAN_POINT ( 'NONE',  ( 44.03140696652192787, 51.19948385550238612, -4.306917132069425058 ) ) ;
#6886=CARTESIAN_POINT ( 'NONE',  ( 56.81924384183011512, 46.19948385550240744, 4.924951120819313743 ) ) ;
#6888=CARTESIAN_POINT ( 'NONE',  ( 51.92680522751238925, 59.40051614449765793, 6.007379884777208190 ) ) ;
#6902=CARTESIAN_POINT ( 'NONE',  ( 42.63976443033212149, 56.99948385550241170, 0.02388180880522514787 ) ) ;
#6906=CARTESIAN_POINT ( 'NONE',  ( 54.68390685589033495, 61.69948385550240744, -6.485486291978119766 ) ) ;
#6909=CARTESIAN_POINT ( 'NONE',  ( 55.11794222512601493, 52.19948385550240744, 3.688883143319541702 ) ) ;
#6915=CARTESIAN_POINT ( 'NONE',  ( 52.57664461997821093, 47.40051614449765793, 8.007379884777206414 ) ) ;
#6916=CARTESIAN_POINT ( 'NONE',  ( 50.02271294988511841, 62.49948385550240459, 6.000000000000000888 ) ) ;
#6927=CARTESIAN_POINT ( 'NONE',  ( 54.09612160359786515, 55.69948385550240744, -5.676469297603166098 ) ) ;
#6938=CARTESIAN_POINT ( 'NONE',  ( 50.02271294988512551, 54.49948385550240459, 7.000000000000000888 ) ) ;
#6940=CARTESIAN_POINT ( 'NONE',  ( 52.25172492374527877, 45.40051614449766504, 7.007379884777203749 ) ) ;
#6959=CARTESIAN_POINT ( 'NONE',  ( 55.11794222512599362, 44.80051614449766362, -3.688883143319583446 ) ) ;
#6962=CARTESIAN_POINT ( 'NONE',  ( 48.02776887271745210, 51.39948385550241028, -5.992620115222778487 ) ) ;
#6964=CARTESIAN_POINT ( 'NONE',  ( 56.79116909180255135, 63.79948385550241596, -4.963592699179005585 ) ) ;
#6965=CARTESIAN_POINT ( 'NONE',  ( 45.27934281921082516, 49.70051614449766220, 6.458785618021089192 ) ) ;
#6974=CARTESIAN_POINT ( 'NONE',  ( 44.05948171654945611, 52.20051614449765509, -4.345558710429044069 ) ) ;
#6980=CARTESIAN_POINT ( 'NONE',  ( 54.13287192849676188, 50.29948385550240175, 5.649768623646098220 ) ) ;
#6982=CARTESIAN_POINT ( 'NONE',  ( 41.58830220609386430, 46.99948385550239749, 0.02388180880523263147 ) ) ;
#6985=CARTESIAN_POINT ( 'NONE',  ( 44.03140696652198471, 45.80051614449764230, 4.306917132069485454 ) ) ;
#6991=CARTESIAN_POINT ( 'NONE',  ( 55.48859070151218020, 45.00000000000002132, -4.999999999999993783 ) ) ;
#6998=CARTESIAN_POINT ( 'NONE',  ( 52.25172492374522903, 59.59948385550239891, -7.007379884777227730 ) ) ;
#7003=CARTESIAN_POINT ( 'NONE',  ( 49.97728705011486738, 59.49948385550240459, -8.000000000000001776 ) ) ;
#7005=CARTESIAN_POINT ( 'NONE',  ( 46.45491332379572924, 53.29948385550240886, -4.840751629271157874 ) ) ;
#7009=CARTESIAN_POINT ( 'NONE',  ( 56.79116909180259398, 47.20051614449766220, 4.963592699178938972 ) ) ;
#7012=CARTESIAN_POINT ( 'NONE',  ( 55.71335778527780036, 48.90051614449766504, -1.832500667257213056 ) ) ;
#7022=CARTESIAN_POINT ( 'NONE',  ( 45.90387839640214196, 60.69948385550240033, 5.676469297603166098 ) ) ;
#7031=CARTESIAN_POINT ( 'NONE',  ( 44.03140696652192787, 49.19948385550240033, -4.306917132069425058 ) ) ;
#7033=CARTESIAN_POINT ( 'NONE',  ( 43.33558569842706021, 47.90051614449765793, 2.141517661632167169 ) ) ;
#7054=CARTESIAN_POINT ( 'NONE',  ( 44.30067958973594955, 48.10051614449766078, -1.875703265242155693 ) ) ;
#7057=ADVANCED_FACE ( 'NONE', ( #7686 ), #6323, .T. ) ;
#7059=CARTESIAN_POINT ( 'NONE',  ( 48.02776887271745210, 53.39948385550241028, -5.992620115222778487 ) ) ;
#7061=CARTESIAN_POINT ( 'NONE',  ( 54.09612160359786515, 47.69948385550240744, -5.676469297603166098 ) ) ;
#7062=CARTESIAN_POINT ( 'NONE',  ( 52.62207051974829852, 46.60051614449764656, -7.992620115222797139 ) ) ;
#7071=CARTESIAN_POINT ( 'NONE',  ( 54.13287192849671214, 50.70051614449766220, -5.649768623646139964 ) ) ;
#7079=CARTESIAN_POINT ( 'NONE',  ( 42.63976443033212860, 48.99948385550240459, 0.02388180880522514787 ) ) ;
#7081=CARTESIAN_POINT ( 'NONE',  ( 45.27934281921075410, 49.29948385550240886, -6.458785618021043895 ) ) ;
#7083=CARTESIAN_POINT ( 'NONE',  ( 50.02271294988505446, 46.50051614449765935, -7.000000000000000888 ) ) ;
#7097=CARTESIAN_POINT ( 'NONE',  ( 50.02271294988513972, 56.49948385550240459, 8.000000000000001776 ) ) ;
#7102=CARTESIAN_POINT ( 'NONE',  ( 56.30877334542961421, 47.99948385550239038, -0.02388180880520959434 ) ) ;
#7105=CARTESIAN_POINT ( 'NONE',  ( 49.97728705011495265, 45.50051614449766646, 8.000000000000001776 ) ) ;
#7107=CARTESIAN_POINT ( 'NONE',  ( 55.11794222512599362, 50.80051614449766362, -3.688883143319583446 ) ) ;
#7119=CARTESIAN_POINT ( 'NONE',  ( 42.63976443033212860, 60.99948385550238328, 0.02388180880522514787 ) ) ;
#7134=CARTESIAN_POINT ( 'NONE',  ( 50.02271294988512551, 48.49948385550240459, 7.000000000000000888 ) ) ;
#7136=CARTESIAN_POINT ( 'NONE',  ( 57.36023556966787851, 51.00051614449763804, 0.02388180880515038476 ) ) ;
#7157=CARTESIAN_POINT ( 'NONE',  ( 48.07319477248762496, 48.40051614449766504, -6.007379884777208190 ) ) ;
#7160=CARTESIAN_POINT ( 'NONE',  ( 53.54508667620428497, 54.29948385550241596, 4.840751629271157874 ) ) ;
#7162=CARTESIAN_POINT ( 'NONE',  ( 45.90387839640214196, 46.69948385550240744, 5.676469297603166098 ) ) ;
#7163=CARTESIAN_POINT ( 'NONE',  ( 43.20883090819742023, 48.20051614449766930, -4.963592699178938972 ) ) ;
#7180=CARTESIAN_POINT ( 'NONE',  ( 42.63976443033212860, 54.99948385550241170, 0.02388180880522514787 ) ) ;
#7182=CARTESIAN_POINT ( 'NONE',  ( 56.79116909180255135, 47.79948385550240886, -4.963592699179005585 ) ) ;
#7184=CARTESIAN_POINT ( 'NONE',  ( 49.97728705011495265, 47.50051614449766646, 7.000000000000000888 ) ) ;
#7199=CARTESIAN_POINT ( 'NONE',  ( 49.97728705011486738, 57.49948385550241170, -8.000000000000001776 ) ) ;
#7201=CARTESIAN_POINT ( 'NONE',  ( 51.97223112728254790, 52.39948385550241028, 5.992620115222778487 ) ) ;
#7204=CARTESIAN_POINT ( 'NONE',  ( 50.02271294988505446, 48.50051614449765935, -8.000000000000001776 ) ) ;
#7206=CARTESIAN_POINT ( 'NONE',  ( 55.71335778527780036, 50.90051614449765793, -1.832500667257213056 ) ) ;
#7230=CARTESIAN_POINT ( 'NONE',  ( 42.63976443033212860, 52.99948385550240459, 0.02388180880522514787 ) ) ;
#7233=CARTESIAN_POINT ( 'NONE',  ( 47.70284917648459100, 47.60051614449763946, 6.992620115222796251 ) ) ;
#7239=ADVANCED_FACE ( 'NONE', ( #12778 ), #919, .F. ) ;
#7257=CARTESIAN_POINT ( 'NONE',  ( 53.50833635130544508, 47.30051614449766362, 4.867452303228181343 ) ) ;
#7261=CARTESIAN_POINT ( 'NONE',  ( 51.97223112728254790, 52.39948385550241028, 5.992620115222778487 ) ) ;
#7263=CARTESIAN_POINT ( 'NONE',  ( 44.05948171654949874, 54.79948385550241596, 4.345558710429105354 ) ) ;
#7265=CARTESIAN_POINT ( 'NONE',  ( 50.02271294988505446, 48.50051614449765935, -8.000000000000001776 ) ) ;
#7278=CARTESIAN_POINT ( 'NONE',  ( 45.90387839640214196, 54.69948385550240744, 5.676469297603166098 ) ) ;
#7280=CARTESIAN_POINT ( 'NONE',  ( 52.62207051974839089, 54.39948385550241028, 7.992620115222770494 ) ) ;
#7283=CARTESIAN_POINT ( 'NONE',  ( 44.03140696652198471, 49.80051614449766362, 4.306917132069485454 ) ) ;
#7300=CARTESIAN_POINT ( 'NONE',  ( 41.58830220609386430, 60.99948385550241170, 0.02388180880523263147 ) ) ;
#7303=CARTESIAN_POINT ( 'NONE',  ( 46.45491332379572924, 57.29948385550240175, -4.840751629271157874 ) ) ;
#7306=CARTESIAN_POINT ( 'NONE',  ( 58.41169779390614281, 49.00051614449765935, 0.02388180880515032231 ) ) ;
#7308=CARTESIAN_POINT ( 'NONE',  ( 46.49166364869456913, 52.30051614449766362, -4.867452303228181343 ) ) ;
#7311=VERTEX_POINT ( 'NONE', #4058 ) ;
#7319=CARTESIAN_POINT ( 'NONE',  ( 57.36023556966787851, 47.99948385550239749, -0.02388180880522424582 ) ) ;
#7326=CARTESIAN_POINT ( 'NONE',  ( 44.05948171654949874, 56.79948385550240886, 4.345558710429105354 ) ) ;
#7328=CARTESIAN_POINT ( 'NONE',  ( 55.94051828345053679, 47.20051614449766220, 4.345558710429044069 ) ) ;
#7337=CARTESIAN_POINT ( 'NONE',  ( 43.18075615816989199, 65.19948385550240744, -4.924951120819313743 ) ) ;
#7348=CARTESIAN_POINT ( 'NONE',  ( 44.88205777487401349, 45.80051614449766362, 3.688883143319584779 ) ) ;
#7352=CARTESIAN_POINT ( 'NONE',  ( 55.11794222512601493, 58.19948385550240744, 3.688883143319541702 ) ) ;
#7354=CARTESIAN_POINT ( 'NONE',  ( 54.09612160359786515, 55.69948385550240744, -5.676469297603166098 ) ) ;
#7356=CARTESIAN_POINT ( 'NONE',  ( 50.02271294988505446, 54.50051614449765935, -8.000000000000001776 ) ) ;
#7377=CARTESIAN_POINT ( 'NONE',  ( 54.09612160359786515, 57.69948385550240744, -5.676469297603166098 ) ) ;
#7379=CARTESIAN_POINT ( 'NONE',  ( 47.42335538002188144, 52.59948385550240602, 8.007379884777233059 ) ) ;
#7381=CARTESIAN_POINT ( 'NONE',  ( 52.29715082351538769, 50.60051614449766788, -6.992620115222796251 ) ) ;
#7398=CARTESIAN_POINT ( 'NONE',  ( 43.69122665457040000, 56.99948385550241170, 0.02388180880521036456 ) ) ;
#7402=CARTESIAN_POINT ( 'NONE',  ( 42.38452918213190657, 53.90051614449765793, 2.450534656007115508 ) ) ;
#7403=CARTESIAN_POINT ( 'NONE',  ( 53.54508667620424234, 48.70051614449766930, -4.840751629271188961 ) ) ;
#7412=CARTESIAN_POINT ( 'NONE',  ( 49.97728705011488159, 63.49948385550241170, -7.000000000000000888 ) ) ;
#7422=CARTESIAN_POINT ( 'NONE',  ( 52.57664461997821093, 63.40051614449765083, 8.007379884777206414 ) ) ;
#7425=CARTESIAN_POINT ( 'NONE',  ( 56.65037692655918988, 55.89948385550240317, -2.184720259617163762 ) ) ;
#7428=CARTESIAN_POINT ( 'NONE',  ( 44.05948171654945611, 56.20051614449764799, -4.345558710429044069 ) ) ;
#7437=CARTESIAN_POINT ( 'NONE',  ( 56.66441430157296821, 46.09948385550240602, 2.141517661632100111 ) ) ;
#7443=CARTESIAN_POINT ( 'NONE',  ( 52.25172492374528588, 61.40051614449765793, 7.007379884777204637 ) ) ;
#7448=CARTESIAN_POINT ( 'NONE',  ( 44.28664221472221385, 57.90051614449765793, 1.832500667257213722 ) ) ;
#7451=CARTESIAN_POINT ( 'NONE',  ( 44.91013252490152752, 58.79948385550240175, 3.727524721679198461 ) ) ;
#7453=CARTESIAN_POINT ( 'NONE',  ( 45.86712807150323812, 55.29948385550240175, -5.649768623646098220 ) ) ;
#7454=CARTESIAN_POINT ( 'NONE',  ( 43.18075615816994173, 51.80051614449766362, 4.924951120819380357 ) ) ;
#7465=CARTESIAN_POINT ( 'NONE',  ( 49.97728705011488159, 61.49948385550240459, -7.000000000000000888 ) ) ;
#7470=CARTESIAN_POINT ( 'NONE',  ( 52.29715082351547295, 58.39948385550238896, 6.992620115222774047 ) ) ;
#7473=CARTESIAN_POINT ( 'NONE',  ( 54.72065718078924590, 54.29948385550241596, 6.458785618021043895 ) ) ;
#7475=CARTESIAN_POINT ( 'NONE',  ( 55.96859303347802239, 52.80051614449764941, -4.306917132069484566 ) ) ;
#7494=CARTESIAN_POINT ( 'NONE',  ( 44.88205777487398507, 59.19948385550240744, -3.688883143319540814 ) ) ;
#7498=CARTESIAN_POINT ( 'NONE',  ( 57.61547081786810764, 50.90051614449765793, -2.450534656007114176 ) ) ;
#7499=CARTESIAN_POINT ( 'NONE',  ( 50.02271294988506156, 58.50051614449765225, -6.000000000000000888 ) ) ;
#7508=CARTESIAN_POINT ( 'NONE',  ( 52.29715082351547295, 64.39948385550239607, 6.992620115222774047 ) ) ;
#7517=CARTESIAN_POINT ( 'NONE',  ( 54.72065718078924590, 48.29948385550240175, 6.458785618021043895 ) ) ;
#7520=CARTESIAN_POINT ( 'NONE',  ( 44.03140696652192787, 59.19948385550238612, -4.306917132069425058 ) ) ;
#7523=CARTESIAN_POINT ( 'NONE',  ( 47.70284917648459100, 51.60051614449765367, 6.992620115222796251 ) ) ;
#7533=CARTESIAN_POINT ( 'NONE',  ( 56.81924384183011512, 64.19948385550240744, 4.924951120819313743 ) ) ;
#7536=ORIENTED_EDGE ( 'NONE', *, *, #16858, .F. ) ;
#7539=CARTESIAN_POINT ( 'NONE',  ( 49.97728705011495265, 61.50051614449765935, 7.000000000000000888 ) ) ;
#7544=CARTESIAN_POINT ( 'NONE',  ( 53.54508667620424234, 54.70051614449765509, -4.840751629271188961 ) ) ;
#7549=CARTESIAN_POINT ( 'NONE',  ( 50.02271294988511841, 56.49948385550240459, 6.000000000000000888 ) ) ;
#7553=CARTESIAN_POINT ( 'NONE',  ( 41.58830220609386430, 52.00051614449766646, -0.02388180880514929535 ) ) ;
#7568=CARTESIAN_POINT ( 'NONE',  ( 52.29715082351547295, 60.39948385550239607, 6.992620115222774047 ) ) ;
#7570=CARTESIAN_POINT ( 'NONE',  ( 42.39856655714566358, 50.89948385550240317, 2.493737253992119207 ) ) ;
#7572=CARTESIAN_POINT ( 'NONE',  ( 44.03140696652198471, 53.80051614449766362, 4.306917132069485454 ) ) ;
#7581=CARTESIAN_POINT ( 'NONE',  ( 44.03140696652192787, 63.19948385550240744, -4.306917132069425058 ) ) ;
#7588=CARTESIAN_POINT ( 'NONE',  ( 51.97223112728254790, 56.39948385550241028, 5.992620115222778487 ) ) ;
#7591=CARTESIAN_POINT ( 'NONE',  ( 57.60143344285435774, 51.10051614449766078, 2.493737253992045044 ) ) ;
#7592=CARTESIAN_POINT ( 'NONE',  ( 55.11794222512599362, 52.80051614449766362, -3.688883143319583446 ) ) ;
#7603=CARTESIAN_POINT ( 'NONE',  ( 44.03140696652192787, 65.19948385550240744, -4.306917132069425058 ) ) ;
#7612=CARTESIAN_POINT ( 'NONE',  ( 56.81924384183011512, 46.19948385550240744, 4.924951120819313743 ) ) ;
#7615=CARTESIAN_POINT ( 'NONE',  ( 56.66441430157296821, 56.09948385550240602, 2.141517661632100111 ) ) ;
#7619=CARTESIAN_POINT ( 'NONE',  ( 54.13287192849671214, 56.70051614449766220, -5.649768623646139964 ) ) ;
#7627=CARTESIAN_POINT ( 'NONE',  ( 45.31609314410967926, 64.69948385550240744, 6.485486291978119766 ) ) ;
#7632=CARTESIAN_POINT ( 'NONE',  ( 54.13287192849671214, 56.70051614449766220, -5.649768623646139964 ) ) ;
#7637=CARTESIAN_POINT ( 'NONE',  ( 55.11794222512599362, 52.80051614449766362, -3.688883143319583446 ) ) ;
#7642=CARTESIAN_POINT ( 'NONE',  ( 49.97728705011488870, 59.49948385550240459, -6.000000000000000888 ) ) ;
#7645=CARTESIAN_POINT ( 'NONE',  ( 57.61547081786810764, 52.90051614449766504, -2.450534656007114176 ) ) ;
#7655=APPLICATION_CONTEXT ( 'automotive_design' ) ;
#7657=CARTESIAN_POINT ( 'NONE',  ( 45.86712807150323812, 61.29948385550240886, -5.649768623646098220 ) ) ;
#7660=DIRECTION ( 'NONE',  ( -0.9989677110047502362, -0.04542589977017699732, 6.931730960091013400E-15 ) ) ;
#7661=CARTESIAN_POINT ( 'NONE',  ( 54.13287192849676188, 58.29948385550240175, 5.649768623646098220 ) ) ;
#7663=CARTESIAN_POINT ( 'NONE',  ( 56.81924384183011512, 54.19948385550241454, 4.924951120819313743 ) ) ;
#7665=CARTESIAN_POINT ( 'NONE',  ( 50.02271294988505446, 52.50051614449765935, -7.000000000000000888 ) ) ;
#7674=CARTESIAN_POINT ( 'NONE',  ( 43.34962307344078880, 48.10051614449766078, -2.184720259617096705 ) ) ;
#7680=CARTESIAN_POINT ( 'NONE',  ( 51.92680522751233951, 57.59948385550240602, -6.007379884777223289 ) ) ;
#7683=CARTESIAN_POINT ( 'NONE',  ( 56.79116909180259398, 55.20051614449766220, 4.963592699178938972 ) ) ;
#7685=CARTESIAN_POINT ( 'NONE',  ( 56.30877334542961421, 55.00051614449766646, 0.02388180880515774693 ) ) ;
#7686=FACE_OUTER_BOUND ( 'NONE', #14495, .T. ) ;
#7698=CARTESIAN_POINT ( 'NONE',  ( 45.86712807150323812, 51.29948385550240175, -5.649768623646098220 ) ) ;
#7702=CARTESIAN_POINT ( 'NONE',  ( 49.97728705011486738, 47.49948385550240459, -8.000000000000001776 ) ) ;
#7705=CARTESIAN_POINT ( 'NONE',  ( 44.05948171654949874, 58.79948385550240886, 4.345558710429105354 ) ) ;
#7708=CARTESIAN_POINT ( 'NONE',  ( 42.63976443033212860, 56.00051614449765935, -0.02388180880514948964 ) ) ;
#7719=CARTESIAN_POINT ( 'NONE',  ( 54.09612160359786515, 45.69948385550240744, -5.676469297603166098 ) ) ;
#7726=CARTESIAN_POINT ( 'NONE',  ( 55.96859303347802239, 56.80051614449764941, -4.306917132069484566 ) ) ;
#7734=CARTESIAN_POINT ( 'NONE',  ( 43.69122665457040000, 58.00051614449765935, -0.02388180880515696977 ) ) ;
#7739=CARTESIAN_POINT ( 'NONE',  ( 44.30067958973596376, 54.89948385550240317, 1.875703265242204099 ) ) ;
#7741=CARTESIAN_POINT ( 'NONE',  ( 54.72065718078918906, 50.70051614449766220, -6.458785618021089192 ) ) ;
#7755=CARTESIAN_POINT ( 'NONE',  ( 42.63976443033212149, 64.99948385550240459, 0.02388180880522514787 ) ) ;
#7760=CARTESIAN_POINT ( 'NONE',  ( 42.63976443033212860, 60.99948385550238328, 0.02388180880522514787 ) ) ;
#7762=CARTESIAN_POINT ( 'NONE',  ( 57.60143344285433642, 59.89948385550240317, -2.493737253992118319 ) ) ;
#7763=CARTESIAN_POINT ( 'NONE',  ( 55.96859303347802239, 56.80051614449764230, -4.306917132069484566 ) ) ;
#7772=CARTESIAN_POINT ( 'NONE',  ( 52.29715082351539479, 48.60051614449766078, -6.992620115222796251 ) ) ;
#7780=CARTESIAN_POINT ( 'NONE',  ( 48.07319477248768180, 64.59948385550241312, 6.007379884777225953 ) ) ;
#7782=CARTESIAN_POINT ( 'NONE',  ( 54.72065718078918906, 60.70051614449766930, -6.458785618021089192 ) ) ;
#7783=CARTESIAN_POINT ( 'NONE',  ( 43.69122665457040000, 54.00051614449765935, -0.02388180880515696977 ) ) ;
#7794=CARTESIAN_POINT ( 'NONE',  ( 55.94051828345050836, 53.79948385550240175, -4.345558710429103577 ) ) ;
#7799=CARTESIAN_POINT ( 'NONE',  ( 50.02271294988513972, 46.49948385550240459, 8.000000000000001776 ) ) ;
#7801=CARTESIAN_POINT ( 'NONE',  ( 45.86712807150323812, 63.29948385550240886, -5.649768623646098220 ) ) ;
#7804=CARTESIAN_POINT ( 'NONE',  ( 42.63976443033212860, 54.00051614449766646, -0.02388180880514948964 ) ) ;
#7809=CARTESIAN_POINT ( 'NONE',  ( 52.25172492374522903, 51.59948385550240602, -7.007379884777225953 ) ) ;
#7815=CARTESIAN_POINT ( 'NONE',  ( 47.74827507625478518, 50.59948385550238470, 7.007379884777227730 ) ) ;
#7822=CARTESIAN_POINT ( 'NONE',  ( 42.63976443033212149, 58.00051614449765225, -0.02388180880514948964 ) ) ;
#7827=B_SPLINE_CURVE_WITH_KNOTS ( 'NONE', 3,
 ( #17191, #17003, #11284, #14323, #3749, #9715, #5117, #9811, #15714, #2294 ),
 .UNSPECIFIED., .F., .F.,
 ( 4, 2, 2, 2, 4 ),
 ( 0.000000000000000000, 0.003112635120760290971, 0.004668952681140444913, 0.005447111461330522535, 0.006225270241520600156 ),
 .UNSPECIFIED. ) ;
#7828=CARTESIAN_POINT ( 'NONE',  ( 55.08986747509849380, 57.20051614449766220, 3.727524721679155384 ) ) ;
#7831=( NAMED_UNIT ( * ) SI_UNIT ( $, .STERADIAN. ) SOLID_ANGLE_UNIT ( ) );
#7833=CARTESIAN_POINT ( 'NONE',  ( 53.54508667620428497, 64.29948385550240175, 4.840751629271157874 ) ) ;
#7835=CARTESIAN_POINT ( 'NONE',  ( 42.39856655714564226, 62.10051614449765367, -2.493737253992044156 ) ) ;
#7859=CARTESIAN_POINT ( 'NONE',  ( 55.08986747509847248, 47.79948385550240886, -3.727524721679197572 ) ) ;
#7861=CARTESIAN_POINT ( 'NONE',  ( 56.81924384183011512, 62.19948385550240744, 4.924951120819313743 ) ) ;
#7862=CARTESIAN_POINT ( 'NONE',  ( 56.65037692655921120, 55.10051614449766078, 2.184720259617097593 ) ) ;
#7867=ORIENTED_EDGE ( 'NONE', *, *, #17008, .F. ) ;
#7870=CARTESIAN_POINT ( 'NONE',  ( 43.33558569842706021, 45.90051614449765793, 2.141517661632167169 ) ) ;
#7877=CARTESIAN_POINT ( 'NONE',  ( 48.02776887271745210, 61.39948385550240317, -5.992620115222778487 ) ) ;
#7880=CARTESIAN_POINT ( 'NONE',  ( 52.57664461997821093, 57.40051614449767214, 8.007379884777206414 ) ) ;
#7881=CARTESIAN_POINT ( 'NONE',  ( 55.08986747509849380, 55.20051614449766220, 3.727524721679155384 ) ) ;
#7893=CARTESIAN_POINT ( 'NONE',  ( 52.25172492374522903, 51.59948385550240602, -7.007379884777227730 ) ) ;
#7898=CARTESIAN_POINT ( 'NONE',  ( 52.57664461997811856, 55.59948385550240602, -8.007379884777229506 ) ) ;
#7901=CARTESIAN_POINT ( 'NONE',  ( 48.02776887271745210, 47.39948385550241028, -5.992620115222778487 ) ) ;
#7903=CARTESIAN_POINT ( 'NONE',  ( 49.97728705011495265, 63.50051614449765935, 7.000000000000000888 ) ) ;
#7906=CARTESIAN_POINT ( 'NONE',  ( 56.66441430157296821, 52.09948385550240602, 2.141517661632100111 ) ) ;
#7910=CARTESIAN_POINT ( 'NONE',  ( 44.05948171654949874, 50.79948385550238754, 4.345558710429105354 ) ) ;
#7915=CARTESIAN_POINT ( 'NONE',  ( 52.29715082351539479, 62.60051614449766078, -6.992620115222796251 ) ) ;
#7922=CARTESIAN_POINT ( 'NONE',  ( 53.50833635130544508, 63.30051614449767072, 4.867452303228181343 ) ) ;
#7926=CARTESIAN_POINT ( 'NONE',  ( 54.68390685589039890, 59.30051614449766362, 6.485486291978072693 ) ) ;
#7946=CARTESIAN_POINT ( 'NONE',  ( 54.13287192849676188, 62.29948385550240886, 5.649768623646098220 ) ) ;
#7948=CARTESIAN_POINT ( 'NONE',  ( 42.39856655714566358, 62.89948385550240317, 2.493737253992119207 ) ) ;
#7949=CARTESIAN_POINT ( 'NONE',  ( 44.05948171654945611, 60.20051614449764799, -4.345558710429044069 ) ) ;
#7958=CARTESIAN_POINT ( 'NONE',  ( 45.90387839640208512, 48.30051614449765651, -5.676469297603124353 ) ) ;
#7959=CARTESIAN_POINT ( 'NONE',  ( 43.33558569842703179, 63.09948385550240602, -2.141517661632099223 ) ) ;
#7964=CARTESIAN_POINT ( 'NONE',  ( 51.92680522751233951, 61.59948385550240602, -6.007379884777223289 ) ) ;
#7966=CARTESIAN_POINT ( 'NONE',  ( 44.05948171654949874, 46.79948385550238754, 4.345558710429105354 ) ) ;
#7968=CARTESIAN_POINT ( 'NONE',  ( 43.18075615816994173, 61.80051614449766362, 4.924951120819380357 ) ) ;
#7970=CARTESIAN_POINT ( 'NONE',  ( 55.96859303347802239, 44.80051614449767072, -4.306917132069484566 ) ) ;
#7976=CARTESIAN_POINT ( 'NONE',  ( 54.65205120807737416, 44.75923773080658918, -4.999999999999772626 ) ) ;
#7982=CARTESIAN_POINT ( 'NONE',  ( 55.96859303347805081, 54.19948385550240033, 4.306917132069425058 ) ) ;
#7986=CARTESIAN_POINT ( 'NONE',  ( 57.60143344285433642, 53.89948385550240317, -2.493737253992118319 ) ) ;
#7989=CARTESIAN_POINT ( 'NONE',  ( 50.02271294988512551, 62.49948385550240459, 7.000000000000000888 ) ) ;
#7992=CARTESIAN_POINT ( 'NONE',  ( 54.09612160359792199, 59.30051614449766362, 5.676469297603124353 ) ) ;
#7994=CARTESIAN_POINT ( 'NONE',  ( 42.63976443033212860, 60.99948385550238328, 0.02388180880522514787 ) ) ;
#8003=CARTESIAN_POINT ( 'NONE',  ( 43.33558569842703179, 49.09948385550240602, -2.141517661632099223 ) ) ;
#8015=CARTESIAN_POINT ( 'NONE',  ( 49.97728705011494554, 63.50051614449765935, 6.000000000000000888 ) ) ;
#8018=CARTESIAN_POINT ( 'NONE',  ( 41.58830220609386430, 60.00051614449765935, -0.02388180880514929535 ) ) ;
#8035=CARTESIAN_POINT ( 'NONE',  ( 47.70284917648453415, 65.39948385550239607, -6.992620115222774047 ) ) ;
#8038=CARTESIAN_POINT ( 'NONE',  ( 43.18075615816989199, 59.19948385550240744, -4.924951120819313743 ) ) ;
#8040=CARTESIAN_POINT ( 'NONE',  ( 45.86712807150329496, 61.70051614449766220, 5.649768623646139964 ) ) ;
#8055=CARTESIAN_POINT ( 'NONE',  ( 44.28664221472220675, 63.09948385550240602, -1.832500667257165317 ) ) ;
#8057=CARTESIAN_POINT ( 'NONE',  ( 44.03140696652192787, 47.19948385550240744, -4.306917132069425058 ) ) ;
#8060=CARTESIAN_POINT ( 'NONE',  ( 45.31609314410960820, 62.30051614449766362, -6.485486291978072693 ) ) ;
#8062=CARTESIAN_POINT ( 'NONE',  ( 53.50833635130544508, 61.30051614449766362, 4.867452303228181343 ) ) ;
#8077=CARTESIAN_POINT ( 'NONE',  ( 55.94051828345050836, 49.79948385550240175, -4.345558710429103577 ) ) ;
#8082=CARTESIAN_POINT ( 'NONE',  ( 52.57664461997811856, 53.59948385550240602, -8.007379884777229506 ) ) ;
#8084=CARTESIAN_POINT ( 'NONE',  ( 45.90387839640214196, 64.69948385550240744, 5.676469297603166098 ) ) ;
#8088=CARTESIAN_POINT ( 'NONE',  ( 42.63976443033212860, 58.00051614449765225, -0.02388180880514948964 ) ) ;
#8090=CARTESIAN_POINT ( 'NONE',  ( 43.34962307344081012, 56.89948385550240317, 2.184720259617164650 ) ) ;
#8098=CARTESIAN_POINT ( 'NONE',  ( 55.94051828345050836, 53.79948385550238754, -4.345558710429104465 ) ) ;
#8109=CARTESIAN_POINT ( 'NONE',  ( 52.25172492374522903, 47.59948385550239891, -7.007379884777225953 ) ) ;
#8111=CARTESIAN_POINT ( 'NONE',  ( 44.88205777487401349, 59.80051614449766362, 3.688883143319584779 ) ) ;
#8117=CARTESIAN_POINT ( 'NONE',  ( 50.02271294988505446, 60.50051614449766646, -8.000000000000001776 ) ) ;
#8121=( LENGTH_UNIT ( ) NAMED_UNIT ( * ) SI_UNIT ( .MILLI., .METRE. ) );
#8137=CARTESIAN_POINT ( 'NONE',  ( 48.07319477248768180, 46.59948385550239891, 6.007379884777225953 ) ) ;
#8141=CARTESIAN_POINT ( 'NONE',  ( 57.60143344285433642, 57.89948385550241028, -2.493737253992118319 ) ) ;
#8142=CARTESIAN_POINT ( 'NONE',  ( 56.65037692655921120, 59.10051614449766078, 2.184720259617097593 ) ) ;
#8152=CARTESIAN_POINT ( 'NONE',  ( 45.86712807150329496, 53.70051614449766220, 5.649768623646139964 ) ) ;
#8162=CARTESIAN_POINT ( 'NONE',  ( 54.72065718078918906, 62.70051614449766220, -6.458785618021089192 ) ) ;
#8164=CARTESIAN_POINT ( 'NONE',  ( 55.08986747509849380, 63.20051614449766220, 3.727524721679155384 ) ) ;
#8178=CARTESIAN_POINT ( 'NONE',  ( 45.90387839640214196, 60.69948385550240033, 5.676469297603166098 ) ) ;
#8183=CARTESIAN_POINT ( 'NONE',  ( 52.62207051974839089, 54.39948385550241028, 7.992620115222770494 ) ) ;
#8188=CARTESIAN_POINT ( 'NONE',  ( 50.02271294988512551, 64.49948385550240459, 7.000000000000000888 ) ) ;
#8191=CARTESIAN_POINT ( 'NONE',  ( 55.96859303347802239, 60.80051614449764941, -4.306917132069484566 ) ) ;
#8193=CARTESIAN_POINT ( 'NONE',  ( 46.45491332379572924, 63.29948385550240175, -4.840751629271157874 ) ) ;
#8195=CARTESIAN_POINT ( 'NONE',  ( 55.96859303347804371, 56.19948385550241454, 4.306917132069425946 ) ) ;
#8202=CARTESIAN_POINT ( 'NONE',  ( 45.86712807150323812, 49.29948385550240175, -5.649768623646098220 ) ) ;
#8213=CARTESIAN_POINT ( 'NONE',  ( 56.65037692655918988, 47.89948385550240317, -2.184720259617163762 ) ) ;
#8216=CARTESIAN_POINT ( 'NONE',  ( 48.07319477248762496, 64.40051614449764372, -6.007379884777208190 ) ) ;
#8233=CARTESIAN_POINT ( 'NONE',  ( 54.09612160359786515, 63.69948385550240744, -5.676469297603166098 ) ) ;
#8236=CARTESIAN_POINT ( 'NONE',  ( 56.65037692655918988, 45.89948385550240317, -2.184720259617163762 ) ) ;
#8237=CARTESIAN_POINT ( 'NONE',  ( 45.90387839640208512, 64.30051614449766362, -5.676469297603124353 ) ) ;
#8246=CARTESIAN_POINT ( 'NONE',  ( 42.63976443033212149, 50.00051614449765935, -0.02388180880514948964 ) ) ;
#8254=CARTESIAN_POINT ( 'NONE',  ( 50.02271294988512551, 48.49948385550240459, 7.000000000000000888 ) ) ;
#8256=CARTESIAN_POINT ( 'NONE',  ( 56.79116909180255135, 45.79948385550240886, -4.963592699179005585 ) ) ;
#8257=CARTESIAN_POINT ( 'NONE',  ( 48.02776887271750184, 63.60051614449764656, 5.992620115222795363 ) ) ;
#8269=CARTESIAN_POINT ( 'NONE',  ( 52.25172492374522903, 57.59948385550240602, -7.007379884777227730 ) ) ;
#8273=CARTESIAN_POINT ( 'NONE',  ( 47.37792948025162332, 53.39948385550241028, -7.992620115222770494 ) ) ;
#8276=CARTESIAN_POINT ( 'NONE',  ( 44.28664221472220675, 51.09948385550240602, -1.832500667257165317 ) ) ;
#8279=CARTESIAN_POINT ( 'NONE',  ( 44.05948171654945611, 62.20051614449764799, -4.345558710429044069 ) ) ;
#8281=CARTESIAN_POINT ( 'NONE',  ( 44.88205777487398507, 65.19948385550240744, -3.688883143319540814 ) ) ;
#8282=CARTESIAN_POINT ( 'NONE',  ( 49.97728705011488159, 59.49948385550240459, -7.000000000000000888 ) ) ;
#8292=CARTESIAN_POINT ( 'NONE',  ( 49.97728705011488159, 61.49948385550240459, -7.000000000000000888 ) ) ;
#8298=CARTESIAN_POINT ( 'NONE',  ( 44.03140696652198471, 63.80051614449764941, 4.306917132069485454 ) ) ;
#8304=CARTESIAN_POINT ( 'NONE',  ( 54.13287192849671214, 44.70051614449766220, -5.649768623646139964 ) ) ;
#8306=CARTESIAN_POINT ( 'NONE',  ( 49.97728705011488159, 45.49948385550240459, -7.000000000000000888 ) ) ;
#8313=SURFACE_SIDE_STYLE ('',( #15581 ) ) ;
#8315=MECHANICAL_DESIGN_GEOMETRIC_PRESENTATION_REPRESENTATION('',(#10189),#19319);
#8330=CARTESIAN_POINT ( 'NONE',  ( 51.97223112728254790, 48.39948385550240317, 5.992620115222778487 ) ) ;
#8332=CARTESIAN_POINT ( 'NONE',  ( 58.41169779390614281, 63.99948385550241170, -0.02388180880523160798 ) ) ;
#8333=CARTESIAN_POINT ( 'NONE',  ( 56.66441430157294690, 62.90051614449765083, -2.141517661632166281 ) ) ;
#8341=CARTESIAN_POINT ( 'NONE',  ( 44.05948171654945611, 50.20051614449765509, -4.345558710429044069 ) ) ;
#8351=CARTESIAN_POINT ( 'NONE',  ( 50.02271294988512551, 50.49948385550240459, 7.000000000000000888 ) ) ;
#8353=CARTESIAN_POINT ( 'NONE',  ( 42.38452918213188525, 47.09948385550240602, -2.450534656007040013 ) ) ;
#8356=CARTESIAN_POINT ( 'NONE',  ( 48.07319477248762496, 64.40051614449764372, -6.007379884777208190 ) ) ;
#8368=CARTESIAN_POINT ( 'NONE',  ( 54.13287192849676188, 58.29948385550240175, 5.649768623646098220 ) ) ;
#8373=CARTESIAN_POINT ( 'NONE',  ( 54.72065718078924590, 58.29948385550240886, 6.458785618021043895 ) ) ;
#8376=CARTESIAN_POINT ( 'NONE',  ( 44.88205777487398507, 53.19948385550240744, -3.688883143319540814 ) ) ;
#8379=CARTESIAN_POINT ( 'NONE',  ( 42.39856655714564226, 46.10051614449766078, -2.493737253992044156 ) ) ;
#8380=CARTESIAN_POINT ( 'NONE',  ( 56.30877334542961421, 63.99948385550241170, -0.02388180880520959434 ) ) ;
#8390=CARTESIAN_POINT ( 'NONE',  ( 44.03140696652192787, 59.19948385550238612, -4.306917132069425058 ) ) ;
#8400=CARTESIAN_POINT ( 'NONE',  ( 44.05948171654949874, 50.79948385550238754, 4.345558710429105354 ) ) ;
#8402=CARTESIAN_POINT ( 'NONE',  ( 42.63976443033212860, 50.00051614449766646, -0.02388180880514948964 ) ) ;
#8425=CARTESIAN_POINT ( 'NONE',  ( 49.97728705011488870, 65.49948385550240459, -6.000000000000000888 ) ) ;
#8430=CARTESIAN_POINT ( 'NONE',  ( 46.49166364869460466, 52.69948385550240744, 4.867452303228209765 ) ) ;
#8432=CARTESIAN_POINT ( 'NONE',  ( 43.20883090819745576, 64.79948385550240175, 4.963592699179006473 ) ) ;
#8434=CARTESIAN_POINT ( 'NONE',  ( 50.02271294988505446, 64.50051614449765225, -7.000000000000000888 ) ) ;
#8445=CARTESIAN_POINT ( 'NONE',  ( 50.02271294988505446, 52.50051614449765935, -7.000000000000000888 ) ) ;
#8450=CARTESIAN_POINT ( 'NONE',  ( 55.41777406314699306, 44.91366546079681399, -4.999999999999999112 ) ) ;
#8455=CARTESIAN_POINT ( 'NONE',  ( 55.94051828345050836, 53.79948385550238754, -4.345558710429104465 ) ) ;
#8458=CARTESIAN_POINT ( 'NONE',  ( 50.02271294988513972, 46.49948385550240459, 8.000000000000001776 ) ) ;
#8460=CARTESIAN_POINT ( 'NONE',  ( 54.13287192849671214, 46.70051614449766220, -5.649768623646139964 ) ) ;
#8474=CARTESIAN_POINT ( 'NONE',  ( 43.34962307344081012, 58.89948385550241028, 2.184720259617164650 ) ) ;
#8475=ORIENTED_EDGE ( 'NONE', *, *, #11067, .T. ) ;
#8479=CARTESIAN_POINT ( 'NONE',  ( 56.81924384183011512, 56.19948385550240744, 4.924951120819313743 ) ) ;
#8482=CARTESIAN_POINT ( 'NONE',  ( 49.97728705011488870, 49.49948385550241170, -6.000000000000000888 ) ) ;
#8489=CARTESIAN_POINT ( 'NONE',  ( 57.60143344285435774, 45.10051614449766788, 2.493737253992045044 ) ) ;
#8490=CARTESIAN_POINT ( 'NONE',  ( 48.02776887271750184, 49.60051614449766788, 5.992620115222795363 ) ) ;
#8500=CARTESIAN_POINT ( 'NONE',  ( 56.66441430157296821, 56.09948385550240602, 2.141517661632100111 ) ) ;
#8513=CARTESIAN_POINT ( 'NONE',  ( 50.02271294988512551, 52.49948385550240459, 7.000000000000000888 ) ) ;
#8515=CARTESIAN_POINT ( 'NONE',  ( 50.02271294988505446, 50.50051614449765935, -7.000000000000000888 ) ) ;
#8531=CARTESIAN_POINT ( 'NONE',  ( 44.30067958973594955, 46.10051614449766078, -1.875703265242155693 ) ) ;
#8534=CARTESIAN_POINT ( 'NONE',  ( 49.97728705011488870, 53.49948385550240459, -6.000000000000000888 ) ) ;
#8536=CARTESIAN_POINT ( 'NONE',  ( 43.33558569842703179, 47.09948385550240602, -2.141517661632099223 ) ) ;
#8537=CARTESIAN_POINT ( 'NONE',  ( 47.37792948025170858, 47.60051614449766078, 7.992620115222797139 ) ) ;
#8546=CARTESIAN_POINT ( 'NONE',  ( 43.34962307344078880, 56.10051614449766078, -2.184720259617096705 ) ) ;
#8550=CARTESIAN_POINT ( 'NONE',  ( 54.89903213687075834, 44.74560054925188268, -5.000000000000007105 ) ) ;
#8555=CARTESIAN_POINT ( 'NONE',  ( 49.97728705011488159, 49.49948385550240459, -7.000000000000000888 ) ) ;
#8557=( BOUNDED_SURFACE ( )  B_SPLINE_SURFACE ( 3, 2, ( 
 ( #11048, #10954, #16963, #3610, #12528, #11141, #12721, #764, #17148, #13983, #15569, #3518, #9672, #18538, #6735, #15671, #9481, #5270, #570, #17056, #2147, #8109, #2257, #5081, #8213, #18724, #11242, #17250, #15772, #2352, #7134, #5561, #6835, #4101, #2833, #16162, #14483, #7031, #5761, #13013, #17443, #8601, #11439, #4001, #1061, #17733, #5662, #14671, #19019, #17541, #9869, #11727, #2740, #8400, #10069, #13112, #2649, #19119, #8797, #12824, #11532, #16067, #14572, #9961, #4288, #1156, #11635, #3908, #17644, #4194, #8513, #10161, #12917, #15965, #11342, #7230, #5371, #8698, #18827, #10256, #1258, #17349, #14769, #15864, #2446, #14381, #966, #2552, #13208, #16257, #6938, #18921, #19221, #5462, #3021, #18228, #10357, #19318, #13505, #1652, #1350, #16550, #15073, #169, #7425, #11927, #7615, #9182, #13593, #3219, #80, #16360, #9265, #7326, #12216, #6144, #4779, #12116, #4687, #15163, #16742, #261, #18124, #10645, #13301, #5858, #3308, #16653, #6057, #1742, #12023, #14967, #4391, #7705, #1448, #2926, #17830, #7520, #10741, #13684, #6241, #11827, #8888, #14869, #3123, #13401, #17335, #9080, #5960, #17933, #4493, #10449, #16453, #8984, #1546, #18024, #4585, #10543, #18414, #6714, #18509, #12311, #15644, #6621, #15448, #15543, #454, #13780, #17126, #9552, #7989, #9359, #3684, #12598, #18607, #6426, #5056, #9649, #7801, #11217, #10833, #17223, #14157, #4955, #1833, #2122, #370, #2228, #2029, #548, #8188, #3591, #8084, #16934, #5147, #3499, #6519, #740, #3786, #12697, #10928 ),
 ( #14061, #6339, #17033, #16838, #9462, #3398, #18700, #15353, #5245, #12405, #13961, #15253, #11027, #18316, #4872, #11120, #12497, #645, #1937, #7901, #13872, #4077, #2527, #3881, #11610, #7102, #1131, #14356, #18993, #4170, #12799, #8670, #5634, #11320, #12985, #10043, #5532, #16041, #11700, #15745, #8482, #3976, #17516, #939, #14642, #11507, #15939, #6813, #8578, #13085, #11413, #14461, #15839, #18899, #14255, #10135, #8276, #2625, #9751, #1228, #1042, #838, #5738, #18799, #17708, #2322, #9839, #6909, #19093, #7201, #5348, #17324, #12897, #13184, #17417, #19199, #2424, #8376, #7005, #14546, #5435, #17620, #16138, #2716, #9940, #14845, #4561, #12093, #16524, #6122, #16428, #13277, #12190, #10230, #15135, #9055, #1713, #3098, #13373, #16231, #10520, #2805, #18098, #10426, #8958, #4660, #11997, #18000, #5934, #7588, #11895, #14941, #9156, #235, #10618, #7398, #2905, #15043, #7303, #6217, #1625, #7680, #8766, #13569, #19395, #3194, #13661, #1425, #17905, #141, #4264, #16625, #14744, #1330, #19293, #13476, #51, #7494, #4465, #5832, #11801, #2997, #17805, #4361, #1521, #6033, #10326, #16331, #8866, #12471, #1909, #15421, #341, #15519, #18386, #616, #17009, #15329, #11363, #7877, #3474, #7964, #16910, #2002, #10902, #6490, #10718, #9437, #13936, #518, #15889, #18482, #5031, #18200, #11004, #14403, #8055, #6399, #4931, #17371, #3561, #9337, #9528, #3372, #13850, #12377, #9890, #2096, #6593, #14032, #12576, #7780, #18584, #16715, #2473, #431, #13756, #15229, #5392, #3931, #8425 ),
 ( #991, #18290, #1809, #6959, #4757, #3276, #6316, #12289, #9239, #4843, #10805, #16809, #5883, #7348, #5486, #8913, #8531, #14894, #11850, #17856, #4417, #10092, #2670, #13230, #2949, #2858, #17755, #11747, #7257, #2761, #8721, #16181, #16087, #4313, #14501, #11657, #7054, #1085, #4214, #7157, #19240, #13322, #14796, #5785, #8622, #10180, #13037, #10282, #13136, #1373, #16285, #14595, #10382, #1183, #17660, #14695, #1283, #8821, #5689, #19341, #11457, #16385, #1469, #12938, #18946, #17467, #4027, #9988, #15985, #2577, #19043, #19145, #5587, #11557, #17568, #4123, #9200, #12052, #18050, #1675, #18345, #6265, #15283, #7637, #18150, #16477, #4805, #5, #4895, #3147, #3047, #4516, #10672, #13619, #4609, #10571, #290, #16575, #9111, #6081, #12335, #10858, #7544, #10476, #18249, #9388, #5988, #14993, #1574, #13429, #15098, #13529, #391, #6359, #1864, #11954, #3429, #9008, #15379, #16865, #196, #17959, #13713, #103, #9293, #6173, #12143, #7828, #15187, #1764, #4710, #10766, #16676, #3242, #7448, #7734, #13809, #12244, #16767, #3331, #4984, #17351, #767, #6837, #478, #6737, #5085, #18630, #3910, #11244, #9577, #2149, #863, #8111, #12531, #3711, #6547, #18542, #15571, #12826, #12724, #9780, #14088, #12627, #10958, #18726, #13893, #18830, #17059, #16966, #18436, #5171, #676, #11051, #3612, #14185, #6649, #11143, #572, #5373, #11345, #2052, #3520, #5272, #9871, #6448, #9484, #15469, #7922, #17150, #8015, #14281, #1960, #15774, #12429, #13986, #9674, #15673, #2259, #8216, #17253 ),
 ( #3814, #2354, #8304, #5464, #12920, #2651, #19321, #5763, #8701, #6940, #1260, #17832, #11637, #15868, #5861, #4196, #10163, #968, #17646, #11441, #19022, #4004, #11829, #17446, #4394, #1063, #5563, #7328, #19122, #18923, #16260, #7233, #16069, #16164, #7033, #14383, #17735, #2743, #8603, #9963, #4291, #13210, #19223, #13016, #5665, #10258, #15967, #14772, #11729, #2555, #14673, #2835, #8800, #1352, #2448, #8402, #14575, #10071, #13303, #11536, #8515, #14485, #1160, #17543, #4104, #7136, #13114, #9085, #13596, #16553, #1549, #7523, #3221, #14969, #13508, #8986, #15257, #1836, #10451, #13403, #1745, #12314, #2929, #17936, #4496, #16362, #18027, #16456, #3312, #9268, #4782, #8890, #6341, #5963, #18319, #7804, #84, #14871, #16656, #1451, #12221, #3126, #15076, #18231, #18127, #4690, #12026, #13688, #4588, #1655, #13785, #10360, #16745, #6060, #10547, #7708, #12302, #7428, #9184, #373, #11931, #15167, #7619, #3025, #172, #6147, #12119, #10649, #264, #6243, #10744, #3688, #18610, #14065, #650, #8088, #2033, #15647, #6429, #3594, #18418, #12408, #15546, #18514, #5150, #5249, #6717, #11123, #7992, #2126, #4958, #2234, #5059, #12700, #9652, #13964, #17226, #552, #9555, #6625, #12601, #17129, #17036, #8191, #16841, #14160, #743, #18703, #2326, #11220, #3791, #4875, #9756, #841, #15748, #12500, #11030, #8279, #14258, #15451, #6817, #9465, #6523, #12803, #10838, #3402, #9362, #15358, #1942, #13875, #7903, #456, #10931, #16939, #3503, #15842, #11704, #2531, #4080, #8581, #17520 ),
 ( #2427, #17624, #16142, #1045, #10048, #5440, #8489, #3885, #19202, #17328, #7105, #18802, #17711, #16046, #9842, #14749, #8379, #1333, #5353, #12901, #3979, #2719, #10233, #14360, #943, #9943, #4268, #7009, #16235, #6915, #18902, #11510, #19097, #11324, #14549, #13088, #4174, #11416, #15942, #5637, #7204, #11614, #1232, #2628, #17420, #7306, #14465, #2809, #10139, #8770, #8675, #14645, #13189, #12989, #18996, #5741, #5535, #1135, #1812, #9243, #3198, #6036, #4663, #12000, #7498, #16336, #7591, #13376, #2908, #10329, #56, #16719, #9159, #6125, #4366, #18101, #15232, #9057, #13281, #3279, #1629, #13571, #17809, #15047, #8869, #16432, #1428, #19297, #14849, #5835, #17909, #3000, #4761, #16528, #7402, #13664, #10622, #13478, #144, #4468, #11805, #15138, #12096, #18004, #19399, #1716, #16628, #7683, #10429, #3101, #239, #5936, #12194, #6220, #11898, #18203, #8961, #14944, #1524, #10721, #4564, #10523, #4935, #621, #12380, #10906, #6402, #12676, #18678, #7880, #10807, #18589, #9725, #345, #15333, #1912, #13759, #15427, #13853, #722, #6692, #2200, #6320, #3758, #3376, #15722, #5221, #16914, #12293, #14036, #18293, #9626, #13940, #12474, #15620, #15523, #2100, #9441, #11097, #2006, #18487, #11195, #7782, #14136, #3477, #18389, #5126, #16813, #4846, #6597, #17201, #9339, #12580, #7968, #433, #521, #6495, #5035, #8060, #11008, #17104, #3663, #8162, #17015, #3566, #9531, #5511, #18876, #13064, #3859, #1020, #15819, #9819, #12962, #15916, #16020, #2694, #4154, #2606, #5415, #18971 ),
 ( #17493, #8559, #4242, #8256, #14439, #2503, #10018, #6886, #1207, #4055, #8458, #18776, #1110, #19072, #3956, #6982, #8353, #11388, #6789, #8648, #817, #14524, #2303, #7182, #11484, #12775, #17688, #5321, #10205, #14232, #2400, #12874, #5614, #13162, #11295, #17302, #17397, #9918, #7081, #19177, #11587, #14331, #14621, #17599, #10118, #16116, #5719, #915, #11685, #10500, #8940, #10307, #18077, #13552, #7570, #1403, #6017, #10600, #19272, #15120, #12075, #17780, #32, #16505, #11979, #3078, #18180, #2785, #14924, #10409, #4541, #7379, #1696, #17983, #2975, #13256, #15022, #125, #17884, #1499, #2887, #5906, #1311, #16603, #14725, #9034, #16208, #7663, #7473, #7280, #12172, #5811, #4739, #8747, #16314, #13352, #6105, #13644, #11777, #4339, #19372, #219, #4448, #6199, #8848, #14823, #13453, #1601, #11875, #4640, #3176, #9136, #16408, #1890, #10987, #18567, #3549, #12560, #3455, #323, #18662, #16699, #2177, #15498, #8141, #9508, #14014, #5109, #6673, #9600, #16994, #2076, #10700, #3263, #12655, #598, #9421, #8038, #15407, #4917, #13737, #5010, #10789, #6299, #7762, #16892, #14116, #6574, #11079, #1792, #17084, #9224, #6475, #15214, #702, #18464, #3640, #12273, #12454, #18272, #13834, #4826, #16792, #3358, #9320, #15309, #15597, #7861, #415, #6380, #1984, #12359, #18369, #10886, #7948, #13916, #503, #997, #5199, #8628, #12943, #18952, #9703, #6964, #798, #8332, #12752, #14601, #6769, #1190, #9801, #14312, #16092, #8432, #2282, #5593, #15994, #5397, #5492, #15797, #3736 ),
 ( #2583, #2378, #14411, #19050, #8236, #4130, #1091, #18749, #11462, #17474, #4033, #9995, #7162, #11169, #17376, #18856, #8536, #890, #10097, #14506, #11369, #14210, #7061, #13042, #6859, #3937, #11269, #12848, #15703, #11562, #5295, #17578, #17177, #2675, #15896, #17280, #13141, #3840, #9895, #2480, #13237, #4320, #16747, #10840, #2768, #8726, #10288, #18321, #1380, #16845, #14700, #17664, #11855, #9, #19153, #14901, #13434, #17964, #5789, #16291, #5997, #7809, #11961, #1838, #17862, #1291, #7906, #5697, #3405, #4522, #9366, #10746, #3314, #13788, #15361, #4877, #9271, #15261, #11663, #4219, #1944, #375, #4425, #6344, #10389, #13327, #12316, #10186, #16186, #8920, #1475, #2955, #2865, #7263, #19247, #16390, #11753, #17760, #7453, #19347, #8828, #14801, #7354, #5889, #18518, #654, #9467, #8195, #9557, #6719, #9654, #12507, #11222, #5060, #8090, #12603, #14067, #6627, #15547, #5152, #458, #18612, #11126, #17131, #15752, #3690, #2127, #13877, #15652, #6431, #12703, #2237, #14163, #2330, #745, #11031, #18706, #17037, #3595, #5251, #8282, #17229, #3795, #9758, #14261, #15453, #844, #4962, #12410, #18420, #554, #2035, #10936, #16942, #3505, #7994, #13966, #6525, #9149, #10613, #16905, #3468, #12088, #15037, #3367, #13931, #4554, #136, #6117, #17994, #230, #18092, #4926, #10895, #6394, #10513, #7959, #7581, #511, #9431, #1708, #16518, #18284, #3091, #13844, #18194, #16709, #426, #334, #6311, #13656, #15324, #6209, #3270, #15415, #11991, #18379, #15129, #16619, #9331, #1619 ) ),
 .UNSPECIFIED., .T., .F., .T. ) 
 B_SPLINE_SURFACE_WITH_KNOTS ( ( 4, 3, 4 ),
 ( 3, 2, 2, 2, 2, 2, 2, 2, 2, 2, 2, 2, 2, 2, 2, 2, 2, 2, 2, 2, 2, 2, 2, 2, 2, 2, 2, 2, 2, 2, 2, 2, 2, 2, 2, 2, 2, 2, 2, 2, 2, 2, 2, 2, 2, 2, 2, 2, 2, 2, 2, 2, 2, 2, 2, 2, 2, 2, 2, 2, 2, 2, 2, 2, 2, 2, 2, 2, 2, 2, 2, 2, 2, 2, 2, 2, 2, 2, 2, 2, 2, 2, 2, 2, 2, 2, 2, 2, 2, 2, 2, 2, 2, 2, 2, 2, 2, 2, 2, 2, 3 ),
 ( 0.000000000000000000, 0.5000000000000000000, 1.000000000000000000 ),
 ( 0.000000000000000000, 0.01000000000000000021, 0.02000000000000000042, 0.02999999999999999889, 0.04000000000000000083, 0.05000000000000000278, 0.05999999999999999778, 0.07000000000000000666, 0.08000000000000000167, 0.08999999999999999667, 0.1000000000000000056, 0.1100000000000000006, 0.1199999999999999956, 0.1300000000000000044, 0.1400000000000000133, 0.1499999999999999944, 0.1600000000000000033, 0.1700000000000000122, 0.1799999999999999933, 0.1900000000000000022, 0.2000000000000000111, 0.2099999999999999922, 0.2200000000000000011, 0.2300000000000000100, 0.2399999999999999911, 0.2500000000000000000, 0.2600000000000000089, 0.2700000000000000178, 0.2800000000000000266, 0.2899999999999999800, 0.2999999999999999889, 0.3099999999999999978, 0.3200000000000000067, 0.3300000000000000155, 0.3400000000000000244, 0.3499999999999999778, 0.3599999999999999867, 0.3699999999999999956, 0.3800000000000000044, 0.3900000000000000133, 0.4000000000000000222, 0.4099999999999999756, 0.4199999999999999845, 0.4299999999999999933, 0.4400000000000000022, 0.4500000000000000111, 0.4600000000000000200, 0.4699999999999999734, 0.4799999999999999822, 0.4899999999999999911, 0.5000000000000000000, 0.5100000000000000089, 0.5200000000000000178, 0.5300000000000000266, 0.5400000000000000355, 0.5500000000000000444, 0.5600000000000000533, 0.5699999999999999512, 0.5799999999999999600, 0.5899999999999999689, 0.5999999999999999778, 0.6099999999999999867, 0.6199999999999999956, 0.6300000000000000044, 0.6400000000000000133, 0.6500000000000000222, 0.6600000000000000311, 0.6700000000000000400, 0.6800000000000000488, 0.6899999999999999467, 0.6999999999999999556, 0.7099999999999999645, 0.7199999999999999734, 0.7299999999999999822, 0.7399999999999999911, 0.7500000000000000000, 0.7600000000000000089, 0.7700000000000000178, 0.7800000000000000266, 0.7900000000000000355, 0.8000000000000000444, 0.8100000000000000533, 0.8199999999999999512, 0.8299999999999999600, 0.8399999999999999689, 0.8499999999999999778, 0.8599999999999999867, 0.8699999999999999956, 0.8800000000000000044, 0.8900000000000000133, 0.9000000000000000222, 0.9100000000000000311, 0.9200000000000000400, 0.9300000000000000488, 0.9399999999999999467, 0.9499999999999999556, 0.9599999999999999645, 0.9699999999999999734, 0.9799999999999999822, 0.9899999999999999911, 1.000000000000000000 ),
 .UNSPECIFIED. ) 
 GEOMETRIC_REPRESENTATION_ITEM ( )  RATIONAL_B_SPLINE_SURFACE ( (
 ( 1.000000000000000000, 0.9510565162951535312, 1.000000000000000000, 0.9510565162951535312, 1.000000000000000000, 0.9510565162951535312, 1.000000000000000000, 0.9510565162951535312, 1.000000000000000000, 0.9510565162951535312, 1.000000000000000000, 0.9510565162951535312, 1.000000000000000000, 0.9510565162951535312, 1.000000000000000000, 0.9510565162951535312, 1.000000000000000000, 0.9510565162951535312, 1.000000000000000000, 0.9510565162951535312, 1.000000000000000000, 0.9510565162951535312, 1.000000000000000000, 0.9510565162951535312, 1.000000000000000000, 0.9510565162951535312, 1.000000000000000000, 0.9510565162951535312, 1.000000000000000000, 0.9510565162951535312, 1.000000000000000000, 0.9510565162951535312, 1.000000000000000000, 0.9510565162951535312, 1.000000000000000000, 0.9510565162951535312, 1.000000000000000000, 0.9510565162951535312, 1.000000000000000000, 0.9510565162951535312, 1.000000000000000000, 0.9510565162951535312, 1.000000000000000000, 0.9510565162951535312, 1.000000000000000000, 0.9510565162951535312, 1.000000000000000000, 0.9510565162951535312, 1.000000000000000000, 0.9510565162951535312, 1.000000000000000000, 0.9510565162951535312, 1.000000000000000000, 0.9510565162951535312, 1.000000000000000000, 0.9510565162951535312, 1.000000000000000000, 0.9510565162951535312, 1.000000000000000000, 0.9510565162951535312, 1.000000000000000000, 0.9510565162951535312, 1.000000000000000000, 0.9510565162951535312, 1.000000000000000000, 0.9510565162951535312, 1.000000000000000000, 0.9510565162951535312, 1.000000000000000000, 0.9510565162951535312, 1.000000000000000000, 0.9510565162951535312, 1.000000000000000000, 0.9510565162951535312, 1.000000000000000000, 0.9510565162951535312, 1.000000000000000000, 0.9510565162951535312, 1.000000000000000000, 0.9510565162951535312, 1.000000000000000000, 0.9510565162951535312, 1.000000000000000000, 0.9510565162951535312, 1.000000000000000000, 0.9510565162951535312, 1.000000000000000000, 0.9510565162951535312, 1.000000000000000000, 0.9510565162951535312, 1.000000000000000000, 0.9510565162951535312, 1.000000000000000000, 0.9510565162951535312, 1.000000000000000000, 0.9510565162951535312, 1.000000000000000000, 0.9510565162951535312, 1.000000000000000000, 0.9510565162951535312, 1.000000000000000000, 0.9510565162951535312, 1.000000000000000000, 0.9510565162951535312, 1.000000000000000000, 0.9510565162951535312, 1.000000000000000000, 0.9510565162951535312, 1.000000000000000000, 0.9510565162951535312, 1.000000000000000000, 0.9510565162951535312, 1.000000000000000000, 0.9510565162951535312, 1.000000000000000000, 0.9510565162951535312, 1.000000000000000000, 0.9510565162951535312, 1.000000000000000000, 0.9510565162951535312, 1.000000000000000000, 0.9510565162951535312, 1.000000000000000000, 0.9510565162951535312, 1.000000000000000000, 0.9510565162951535312, 1.000000000000000000, 0.9510565162951535312, 1.000000000000000000, 0.9510565162951535312, 1.000000000000000000, 0.9510565162951535312, 1.000000000000000000, 0.9510565162951535312, 1.000000000000000000, 0.9510565162951535312, 1.000000000000000000, 0.9510565162951535312, 1.000000000000000000, 0.9510565162951535312, 1.000000000000000000, 0.9510565162951535312, 1.000000000000000000, 0.9510565162951535312, 1.000000000000000000, 0.9510565162951535312, 1.000000000000000000, 0.9510565162951535312, 1.000000000000000000, 0.9510565162951535312, 1.000000000000000000, 0.9510565162951535312, 1.000000000000000000, 0.9510565162951535312, 1.000000000000000000, 0.9510565162951535312, 1.000000000000000000, 0.9510565162951535312, 1.000000000000000000, 0.9510565162951535312, 1.000000000000000000, 0.9510565162951535312, 1.000000000000000000, 0.9510565162951535312, 1.000000000000000000, 0.9510565162951535312, 1.000000000000000000, 0.9510565162951535312, 1.000000000000000000, 0.9510565162951535312, 1.000000000000000000, 0.9510565162951535312, 1.000000000000000000, 0.9510565162951535312, 1.000000000000000000, 0.9510565162951535312, 1.000000000000000000, 0.9510565162951535312, 1.000000000000000000, 0.9510565162951535312, 1.000000000000000000, 0.9510565162951535312, 1.000000000000000000, 0.9510565162951535312, 1.000000000000000000, 0.9510565162951535312, 1.000000000000000000, 0.9510565162951535312, 1.000000000000000000, 0.9510565162951535312, 1.000000000000000000, 0.9510565162951535312, 1.000000000000000000, 0.9510565162951535312, 1.000000000000000000, 0.9510565162951535312, 1.000000000000000000, 0.9510565162951535312, 1.000000000000000000, 0.9510565162951535312, 1.000000000000000000),
 ( 0.3333333333333333703, 0.3170188387650512141, 0.3333333333333333703, 0.3170188387650512141, 0.3333333333333333703, 0.3170188387650512141, 0.3333333333333333703, 0.3170188387650512141, 0.3333333333333333703, 0.3170188387650512141, 0.3333333333333333703, 0.3170188387650512141, 0.3333333333333333703, 0.3170188387650512141, 0.3333333333333333703, 0.3170188387650512141, 0.3333333333333333703, 0.3170188387650512141, 0.3333333333333333703, 0.3170188387650512141, 0.3333333333333333703, 0.3170188387650512141, 0.3333333333333333703, 0.3170188387650512141, 0.3333333333333333703, 0.3170188387650512141, 0.3333333333333333703, 0.3170188387650512141, 0.3333333333333333703, 0.3170188387650512141, 0.3333333333333333703, 0.3170188387650512141, 0.3333333333333333703, 0.3170188387650512141, 0.3333333333333333703, 0.3170188387650512141, 0.3333333333333333703, 0.3170188387650512141, 0.3333333333333333703, 0.3170188387650512141, 0.3333333333333333703, 0.3170188387650512141, 0.3333333333333333703, 0.3170188387650512141, 0.3333333333333333703, 0.3170188387650512141, 0.3333333333333333703, 0.3170188387650512141, 0.3333333333333333703, 0.3170188387650512141, 0.3333333333333333703, 0.3170188387650512141, 0.3333333333333333703, 0.3170188387650512141, 0.3333333333333333703, 0.3170188387650512141, 0.3333333333333333703, 0.3170188387650512141, 0.3333333333333333703, 0.3170188387650512141, 0.3333333333333333703, 0.3170188387650512141, 0.3333333333333333703, 0.3170188387650512141, 0.3333333333333333703, 0.3170188387650512141, 0.3333333333333333703, 0.3170188387650512141, 0.3333333333333333703, 0.3170188387650512141, 0.3333333333333333703, 0.3170188387650512141, 0.3333333333333333703, 0.3170188387650512141, 0.3333333333333333703, 0.3170188387650512141, 0.3333333333333333703, 0.3170188387650512141, 0.3333333333333333703, 0.3170188387650512141, 0.3333333333333333703, 0.3170188387650512141, 0.3333333333333333703, 0.3170188387650512141, 0.3333333333333333703, 0.3170188387650512141, 0.3333333333333333703, 0.3170188387650512141, 0.3333333333333333703, 0.3170188387650512141, 0.3333333333333333703, 0.3170188387650512141, 0.3333333333333333703, 0.3170188387650512141, 0.3333333333333333703, 0.3170188387650512141, 0.3333333333333333703, 0.3170188387650512141, 0.3333333333333333703, 0.3170188387650512141, 0.3333333333333333703, 0.3170188387650512141, 0.3333333333333333703, 0.3170188387650512141, 0.3333333333333333703, 0.3170188387650512141, 0.3333333333333333703, 0.3170188387650512141, 0.3333333333333333703, 0.3170188387650512141, 0.3333333333333333703, 0.3170188387650512141, 0.3333333333333333703, 0.3170188387650512141, 0.3333333333333333703, 0.3170188387650512141, 0.3333333333333333703, 0.3170188387650512141, 0.3333333333333333703, 0.3170188387650512141, 0.3333333333333333703, 0.3170188387650512141, 0.3333333333333333703, 0.3170188387650512141, 0.3333333333333333703, 0.3170188387650512141, 0.3333333333333333703, 0.3170188387650512141, 0.3333333333333333703, 0.3170188387650512141, 0.3333333333333333703, 0.3170188387650512141, 0.3333333333333333703, 0.3170188387650512141, 0.3333333333333333703, 0.3170188387650512141, 0.3333333333333333703, 0.3170188387650512141, 0.3333333333333333703, 0.3170188387650512141, 0.3333333333333333703, 0.3170188387650512141, 0.3333333333333333703, 0.3170188387650512141, 0.3333333333333333703, 0.3170188387650512141, 0.3333333333333333703, 0.3170188387650512141, 0.3333333333333333703, 0.3170188387650512141, 0.3333333333333333703, 0.3170188387650512141, 0.3333333333333333703, 0.3170188387650512141, 0.3333333333333333703, 0.3170188387650512141, 0.3333333333333333703, 0.3170188387650512141, 0.3333333333333333703, 0.3170188387650512141, 0.3333333333333333703, 0.3170188387650512141, 0.3333333333333333703, 0.3170188387650512141, 0.3333333333333333703, 0.3170188387650512141, 0.3333333333333333703, 0.3170188387650512141, 0.3333333333333333703, 0.3170188387650512141, 0.3333333333333333703, 0.3170188387650512141, 0.3333333333333333703, 0.3170188387650512141, 0.3333333333333333703, 0.3170188387650512141, 0.3333333333333333703, 0.3170188387650512141, 0.3333333333333333703, 0.3170188387650512141, 0.3333333333333333703, 0.3170188387650512141, 0.3333333333333333703, 0.3170188387650512141, 0.3333333333333333703, 0.3170188387650512141, 0.3333333333333333703, 0.3170188387650512141, 0.3333333333333333703, 0.3170188387650512141, 0.3333333333333333703, 0.3170188387650512141, 0.3333333333333333703, 0.3170188387650512141, 0.3333333333333333703, 0.3170188387650512141, 0.3333333333333333703, 0.3170188387650512141, 0.3333333333333333703, 0.3170188387650512141, 0.3333333333333333703),
 ( 0.3333333333333333703, 0.3170188387650512141, 0.3333333333333333703, 0.3170188387650512141, 0.3333333333333333703, 0.3170188387650512141, 0.3333333333333333703, 0.3170188387650512141, 0.3333333333333333703, 0.3170188387650512141, 0.3333333333333333703, 0.3170188387650512141, 0.3333333333333333703, 0.3170188387650512141, 0.3333333333333333703, 0.3170188387650512141, 0.3333333333333333703, 0.3170188387650512141, 0.3333333333333333703, 0.3170188387650512141, 0.3333333333333333703, 0.3170188387650512141, 0.3333333333333333703, 0.3170188387650512141, 0.3333333333333333703, 0.3170188387650512141, 0.3333333333333333703, 0.3170188387650512141, 0.3333333333333333703, 0.3170188387650512141, 0.3333333333333333703, 0.3170188387650512141, 0.3333333333333333703, 0.3170188387650512141, 0.3333333333333333703, 0.3170188387650512141, 0.3333333333333333703, 0.3170188387650512141, 0.3333333333333333703, 0.3170188387650512141, 0.3333333333333333703, 0.3170188387650512141, 0.3333333333333333703, 0.3170188387650512141, 0.3333333333333333703, 0.3170188387650512141, 0.3333333333333333703, 0.3170188387650512141, 0.3333333333333333703, 0.3170188387650512141, 0.3333333333333333703, 0.3170188387650512141, 0.3333333333333333703, 0.3170188387650512141, 0.3333333333333333703, 0.3170188387650512141, 0.3333333333333333703, 0.3170188387650512141, 0.3333333333333333703, 0.3170188387650512141, 0.3333333333333333703, 0.3170188387650512141, 0.3333333333333333703, 0.3170188387650512141, 0.3333333333333333703, 0.3170188387650512141, 0.3333333333333333703, 0.3170188387650512141, 0.3333333333333333703, 0.3170188387650512141, 0.3333333333333333703, 0.3170188387650512141, 0.3333333333333333703, 0.3170188387650512141, 0.3333333333333333703, 0.3170188387650512141, 0.3333333333333333703, 0.3170188387650512141, 0.3333333333333333703, 0.3170188387650512141, 0.3333333333333333703, 0.3170188387650512141, 0.3333333333333333703, 0.3170188387650512141, 0.3333333333333333703, 0.3170188387650512141, 0.3333333333333333703, 0.3170188387650512141, 0.3333333333333333703, 0.3170188387650512141, 0.3333333333333333703, 0.3170188387650512141, 0.3333333333333333703, 0.3170188387650512141, 0.3333333333333333703, 0.3170188387650512141, 0.3333333333333333703, 0.3170188387650512141, 0.3333333333333333703, 0.3170188387650512141, 0.3333333333333333703, 0.3170188387650512141, 0.3333333333333333703, 0.3170188387650512141, 0.3333333333333333703, 0.3170188387650512141, 0.3333333333333333703, 0.3170188387650512141, 0.3333333333333333703, 0.3170188387650512141, 0.3333333333333333703, 0.3170188387650512141, 0.3333333333333333703, 0.3170188387650512141, 0.3333333333333333703, 0.3170188387650512141, 0.3333333333333333703, 0.3170188387650512141, 0.3333333333333333703, 0.3170188387650512141, 0.3333333333333333703, 0.3170188387650512141, 0.3333333333333333703, 0.3170188387650512141, 0.3333333333333333703, 0.3170188387650512141, 0.3333333333333333703, 0.3170188387650512141, 0.3333333333333333703, 0.3170188387650512141, 0.3333333333333333703, 0.3170188387650512141, 0.3333333333333333703, 0.3170188387650512141, 0.3333333333333333703, 0.3170188387650512141, 0.3333333333333333703, 0.3170188387650512141, 0.3333333333333333703, 0.3170188387650512141, 0.3333333333333333703, 0.3170188387650512141, 0.3333333333333333703, 0.3170188387650512141, 0.3333333333333333703, 0.3170188387650512141, 0.3333333333333333703, 0.3170188387650512141, 0.3333333333333333703, 0.3170188387650512141, 0.3333333333333333703, 0.3170188387650512141, 0.3333333333333333703, 0.3170188387650512141, 0.3333333333333333703, 0.3170188387650512141, 0.3333333333333333703, 0.3170188387650512141, 0.3333333333333333703, 0.3170188387650512141, 0.3333333333333333703, 0.3170188387650512141, 0.3333333333333333703, 0.3170188387650512141, 0.3333333333333333703, 0.3170188387650512141, 0.3333333333333333703, 0.3170188387650512141, 0.3333333333333333703, 0.3170188387650512141, 0.3333333333333333703, 0.3170188387650512141, 0.3333333333333333703, 0.3170188387650512141, 0.3333333333333333703, 0.3170188387650512141, 0.3333333333333333703, 0.3170188387650512141, 0.3333333333333333703, 0.3170188387650512141, 0.3333333333333333703, 0.3170188387650512141, 0.3333333333333333703, 0.3170188387650512141, 0.3333333333333333703, 0.3170188387650512141, 0.3333333333333333703, 0.3170188387650512141, 0.3333333333333333703, 0.3170188387650512141, 0.3333333333333333703, 0.3170188387650512141, 0.3333333333333333703, 0.3170188387650512141, 0.3333333333333333703, 0.3170188387650512141, 0.3333333333333333703, 0.3170188387650512141, 0.3333333333333333703, 0.3170188387650512141, 0.3333333333333333703),
 ( 1.000000000000000000, 0.9510565162951535312, 1.000000000000000000, 0.9510565162951535312, 1.000000000000000000, 0.9510565162951535312, 1.000000000000000000, 0.9510565162951535312, 1.000000000000000000, 0.9510565162951535312, 1.000000000000000000, 0.9510565162951535312, 1.000000000000000000, 0.9510565162951535312, 1.000000000000000000, 0.9510565162951535312, 1.000000000000000000, 0.9510565162951535312, 1.000000000000000000, 0.9510565162951535312, 1.000000000000000000, 0.9510565162951535312, 1.000000000000000000, 0.9510565162951535312, 1.000000000000000000, 0.9510565162951535312, 1.000000000000000000, 0.9510565162951535312, 1.000000000000000000, 0.9510565162951535312, 1.000000000000000000, 0.9510565162951535312, 1.000000000000000000, 0.9510565162951535312, 1.000000000000000000, 0.9510565162951535312, 1.000000000000000000, 0.9510565162951535312, 1.000000000000000000, 0.9510565162951535312, 1.000000000000000000, 0.9510565162951535312, 1.000000000000000000, 0.9510565162951535312, 1.000000000000000000, 0.9510565162951535312, 1.000000000000000000, 0.9510565162951535312, 1.000000000000000000, 0.9510565162951535312, 1.000000000000000000, 0.9510565162951535312, 1.000000000000000000, 0.9510565162951535312, 1.000000000000000000, 0.9510565162951535312, 1.000000000000000000, 0.9510565162951535312, 1.000000000000000000, 0.9510565162951535312, 1.000000000000000000, 0.9510565162951535312, 1.000000000000000000, 0.9510565162951535312, 1.000000000000000000, 0.9510565162951535312, 1.000000000000000000, 0.9510565162951535312, 1.000000000000000000, 0.9510565162951535312, 1.000000000000000000, 0.9510565162951535312, 1.000000000000000000, 0.9510565162951535312, 1.000000000000000000, 0.9510565162951535312, 1.000000000000000000, 0.9510565162951535312, 1.000000000000000000, 0.9510565162951535312, 1.000000000000000000, 0.9510565162951535312, 1.000000000000000000, 0.9510565162951535312, 1.000000000000000000, 0.9510565162951535312, 1.000000000000000000, 0.9510565162951535312, 1.000000000000000000, 0.9510565162951535312, 1.000000000000000000, 0.9510565162951535312, 1.000000000000000000, 0.9510565162951535312, 1.000000000000000000, 0.9510565162951535312, 1.000000000000000000, 0.9510565162951535312, 1.000000000000000000, 0.9510565162951535312, 1.000000000000000000, 0.9510565162951535312, 1.000000000000000000, 0.9510565162951535312, 1.000000000000000000, 0.9510565162951535312, 1.000000000000000000, 0.9510565162951535312, 1.000000000000000000, 0.9510565162951535312, 1.000000000000000000, 0.9510565162951535312, 1.000000000000000000, 0.9510565162951535312, 1.000000000000000000, 0.9510565162951535312, 1.000000000000000000, 0.9510565162951535312, 1.000000000000000000, 0.9510565162951535312, 1.000000000000000000, 0.9510565162951535312, 1.000000000000000000, 0.9510565162951535312, 1.000000000000000000, 0.9510565162951535312, 1.000000000000000000, 0.9510565162951535312, 1.000000000000000000, 0.9510565162951535312, 1.000000000000000000, 0.9510565162951535312, 1.000000000000000000, 0.9510565162951535312, 1.000000000000000000, 0.9510565162951535312, 1.000000000000000000, 0.9510565162951535312, 1.000000000000000000, 0.9510565162951535312, 1.000000000000000000, 0.9510565162951535312, 1.000000000000000000, 0.9510565162951535312, 1.000000000000000000, 0.9510565162951535312, 1.000000000000000000, 0.9510565162951535312, 1.000000000000000000, 0.9510565162951535312, 1.000000000000000000, 0.9510565162951535312, 1.000000000000000000, 0.9510565162951535312, 1.000000000000000000, 0.9510565162951535312, 1.000000000000000000, 0.9510565162951535312, 1.000000000000000000, 0.9510565162951535312, 1.000000000000000000, 0.9510565162951535312, 1.000000000000000000, 0.9510565162951535312, 1.000000000000000000, 0.9510565162951535312, 1.000000000000000000, 0.9510565162951535312, 1.000000000000000000, 0.9510565162951535312, 1.000000000000000000, 0.9510565162951535312, 1.000000000000000000, 0.9510565162951535312, 1.000000000000000000, 0.9510565162951535312, 1.000000000000000000, 0.9510565162951535312, 1.000000000000000000, 0.9510565162951535312, 1.000000000000000000, 0.9510565162951535312, 1.000000000000000000, 0.9510565162951535312, 1.000000000000000000, 0.9510565162951535312, 1.000000000000000000, 0.9510565162951535312, 1.000000000000000000, 0.9510565162951535312, 1.000000000000000000, 0.9510565162951535312, 1.000000000000000000, 0.9510565162951535312, 1.000000000000000000, 0.9510565162951535312, 1.000000000000000000, 0.9510565162951535312, 1.000000000000000000, 0.9510565162951535312, 1.000000000000000000),
 ( 0.3333333333333333703, 0.3170188387650512141, 0.3333333333333333703, 0.3170188387650512141, 0.3333333333333333703, 0.3170188387650512141, 0.3333333333333333703, 0.3170188387650512141, 0.3333333333333333703, 0.3170188387650512141, 0.3333333333333333703, 0.3170188387650512141, 0.3333333333333333703, 0.3170188387650512141, 0.3333333333333333703, 0.3170188387650512141, 0.3333333333333333703, 0.3170188387650512141, 0.3333333333333333703, 0.3170188387650512141, 0.3333333333333333703, 0.3170188387650512141, 0.3333333333333333703, 0.3170188387650512141, 0.3333333333333333703, 0.3170188387650512141, 0.3333333333333333703, 0.3170188387650512141, 0.3333333333333333703, 0.3170188387650512141, 0.3333333333333333703, 0.3170188387650512141, 0.3333333333333333703, 0.3170188387650512141, 0.3333333333333333703, 0.3170188387650512141, 0.3333333333333333703, 0.3170188387650512141, 0.3333333333333333703, 0.3170188387650512141, 0.3333333333333333703, 0.3170188387650512141, 0.3333333333333333703, 0.3170188387650512141, 0.3333333333333333703, 0.3170188387650512141, 0.3333333333333333703, 0.3170188387650512141, 0.3333333333333333703, 0.3170188387650512141, 0.3333333333333333703, 0.3170188387650512141, 0.3333333333333333703, 0.3170188387650512141, 0.3333333333333333703, 0.3170188387650512141, 0.3333333333333333703, 0.3170188387650512141, 0.3333333333333333703, 0.3170188387650512141, 0.3333333333333333703, 0.3170188387650512141, 0.3333333333333333703, 0.3170188387650512141, 0.3333333333333333703, 0.3170188387650512141, 0.3333333333333333703, 0.3170188387650512141, 0.3333333333333333703, 0.3170188387650512141, 0.3333333333333333703, 0.3170188387650512141, 0.3333333333333333703, 0.3170188387650512141, 0.3333333333333333703, 0.3170188387650512141, 0.3333333333333333703, 0.3170188387650512141, 0.3333333333333333703, 0.3170188387650512141, 0.3333333333333333703, 0.3170188387650512141, 0.3333333333333333703, 0.3170188387650512141, 0.3333333333333333703, 0.3170188387650512141, 0.3333333333333333703, 0.3170188387650512141, 0.3333333333333333703, 0.3170188387650512141, 0.3333333333333333703, 0.3170188387650512141, 0.3333333333333333703, 0.3170188387650512141, 0.3333333333333333703, 0.3170188387650512141, 0.3333333333333333703, 0.3170188387650512141, 0.3333333333333333703, 0.3170188387650512141, 0.3333333333333333703, 0.3170188387650512141, 0.3333333333333333703, 0.3170188387650512141, 0.3333333333333333703, 0.3170188387650512141, 0.3333333333333333703, 0.3170188387650512141, 0.3333333333333333703, 0.3170188387650512141, 0.3333333333333333703, 0.3170188387650512141, 0.3333333333333333703, 0.3170188387650512141, 0.3333333333333333703, 0.3170188387650512141, 0.3333333333333333703, 0.3170188387650512141, 0.3333333333333333703, 0.3170188387650512141, 0.3333333333333333703, 0.3170188387650512141, 0.3333333333333333703, 0.3170188387650512141, 0.3333333333333333703, 0.3170188387650512141, 0.3333333333333333703, 0.3170188387650512141, 0.3333333333333333703, 0.3170188387650512141, 0.3333333333333333703, 0.3170188387650512141, 0.3333333333333333703, 0.3170188387650512141, 0.3333333333333333703, 0.3170188387650512141, 0.3333333333333333703, 0.3170188387650512141, 0.3333333333333333703, 0.3170188387650512141, 0.3333333333333333703, 0.3170188387650512141, 0.3333333333333333703, 0.3170188387650512141, 0.3333333333333333703, 0.3170188387650512141, 0.3333333333333333703, 0.3170188387650512141, 0.3333333333333333703, 0.3170188387650512141, 0.3333333333333333703, 0.3170188387650512141, 0.3333333333333333703, 0.3170188387650512141, 0.3333333333333333703, 0.3170188387650512141, 0.3333333333333333703, 0.3170188387650512141, 0.3333333333333333703, 0.3170188387650512141, 0.3333333333333333703, 0.3170188387650512141, 0.3333333333333333703, 0.3170188387650512141, 0.3333333333333333703, 0.3170188387650512141, 0.3333333333333333703, 0.3170188387650512141, 0.3333333333333333703, 0.3170188387650512141, 0.3333333333333333703, 0.3170188387650512141, 0.3333333333333333703, 0.3170188387650512141, 0.3333333333333333703, 0.3170188387650512141, 0.3333333333333333703, 0.3170188387650512141, 0.3333333333333333703, 0.3170188387650512141, 0.3333333333333333703, 0.3170188387650512141, 0.3333333333333333703, 0.3170188387650512141, 0.3333333333333333703, 0.3170188387650512141, 0.3333333333333333703, 0.3170188387650512141, 0.3333333333333333703, 0.3170188387650512141, 0.3333333333333333703, 0.3170188387650512141, 0.3333333333333333703, 0.3170188387650512141, 0.3333333333333333703, 0.3170188387650512141, 0.3333333333333333703, 0.3170188387650512141, 0.3333333333333333703, 0.3170188387650512141, 0.3333333333333333703),
 ( 0.3333333333333333703, 0.3170188387650512141, 0.3333333333333333703, 0.3170188387650512141, 0.3333333333333333703, 0.3170188387650512141, 0.3333333333333333703, 0.3170188387650512141, 0.3333333333333333703, 0.3170188387650512141, 0.3333333333333333703, 0.3170188387650512141, 0.3333333333333333703, 0.3170188387650512141, 0.3333333333333333703, 0.3170188387650512141, 0.3333333333333333703, 0.3170188387650512141, 0.3333333333333333703, 0.3170188387650512141, 0.3333333333333333703, 0.3170188387650512141, 0.3333333333333333703, 0.3170188387650512141, 0.3333333333333333703, 0.3170188387650512141, 0.3333333333333333703, 0.3170188387650512141, 0.3333333333333333703, 0.3170188387650512141, 0.3333333333333333703, 0.3170188387650512141, 0.3333333333333333703, 0.3170188387650512141, 0.3333333333333333703, 0.3170188387650512141, 0.3333333333333333703, 0.3170188387650512141, 0.3333333333333333703, 0.3170188387650512141, 0.3333333333333333703, 0.3170188387650512141, 0.3333333333333333703, 0.3170188387650512141, 0.3333333333333333703, 0.3170188387650512141, 0.3333333333333333703, 0.3170188387650512141, 0.3333333333333333703, 0.3170188387650512141, 0.3333333333333333703, 0.3170188387650512141, 0.3333333333333333703, 0.3170188387650512141, 0.3333333333333333703, 0.3170188387650512141, 0.3333333333333333703, 0.3170188387650512141, 0.3333333333333333703, 0.3170188387650512141, 0.3333333333333333703, 0.3170188387650512141, 0.3333333333333333703, 0.3170188387650512141, 0.3333333333333333703, 0.3170188387650512141, 0.3333333333333333703, 0.3170188387650512141, 0.3333333333333333703, 0.3170188387650512141, 0.3333333333333333703, 0.3170188387650512141, 0.3333333333333333703, 0.3170188387650512141, 0.3333333333333333703, 0.3170188387650512141, 0.3333333333333333703, 0.3170188387650512141, 0.3333333333333333703, 0.3170188387650512141, 0.3333333333333333703, 0.3170188387650512141, 0.3333333333333333703, 0.3170188387650512141, 0.3333333333333333703, 0.3170188387650512141, 0.3333333333333333703, 0.3170188387650512141, 0.3333333333333333703, 0.3170188387650512141, 0.3333333333333333703, 0.3170188387650512141, 0.3333333333333333703, 0.3170188387650512141, 0.3333333333333333703, 0.3170188387650512141, 0.3333333333333333703, 0.3170188387650512141, 0.3333333333333333703, 0.3170188387650512141, 0.3333333333333333703, 0.3170188387650512141, 0.3333333333333333703, 0.3170188387650512141, 0.3333333333333333703, 0.3170188387650512141, 0.3333333333333333703, 0.3170188387650512141, 0.3333333333333333703, 0.3170188387650512141, 0.3333333333333333703, 0.3170188387650512141, 0.3333333333333333703, 0.3170188387650512141, 0.3333333333333333703, 0.3170188387650512141, 0.3333333333333333703, 0.3170188387650512141, 0.3333333333333333703, 0.3170188387650512141, 0.3333333333333333703, 0.3170188387650512141, 0.3333333333333333703, 0.3170188387650512141, 0.3333333333333333703, 0.3170188387650512141, 0.3333333333333333703, 0.3170188387650512141, 0.3333333333333333703, 0.3170188387650512141, 0.3333333333333333703, 0.3170188387650512141, 0.3333333333333333703, 0.3170188387650512141, 0.3333333333333333703, 0.3170188387650512141, 0.3333333333333333703, 0.3170188387650512141, 0.3333333333333333703, 0.3170188387650512141, 0.3333333333333333703, 0.3170188387650512141, 0.3333333333333333703, 0.3170188387650512141, 0.3333333333333333703, 0.3170188387650512141, 0.3333333333333333703, 0.3170188387650512141, 0.3333333333333333703, 0.3170188387650512141, 0.3333333333333333703, 0.3170188387650512141, 0.3333333333333333703, 0.3170188387650512141, 0.3333333333333333703, 0.3170188387650512141, 0.3333333333333333703, 0.3170188387650512141, 0.3333333333333333703, 0.3170188387650512141, 0.3333333333333333703, 0.3170188387650512141, 0.3333333333333333703, 0.3170188387650512141, 0.3333333333333333703, 0.3170188387650512141, 0.3333333333333333703, 0.3170188387650512141, 0.3333333333333333703, 0.3170188387650512141, 0.3333333333333333703, 0.3170188387650512141, 0.3333333333333333703, 0.3170188387650512141, 0.3333333333333333703, 0.3170188387650512141, 0.3333333333333333703, 0.3170188387650512141, 0.3333333333333333703, 0.3170188387650512141, 0.3333333333333333703, 0.3170188387650512141, 0.3333333333333333703, 0.3170188387650512141, 0.3333333333333333703, 0.3170188387650512141, 0.3333333333333333703, 0.3170188387650512141, 0.3333333333333333703, 0.3170188387650512141, 0.3333333333333333703, 0.3170188387650512141, 0.3333333333333333703, 0.3170188387650512141, 0.3333333333333333703, 0.3170188387650512141, 0.3333333333333333703, 0.3170188387650512141, 0.3333333333333333703, 0.3170188387650512141, 0.3333333333333333703),
 ( 1.000000000000000000, 0.9510565162951535312, 1.000000000000000000, 0.9510565162951535312, 1.000000000000000000, 0.9510565162951535312, 1.000000000000000000, 0.9510565162951535312, 1.000000000000000000, 0.9510565162951535312, 1.000000000000000000, 0.9510565162951535312, 1.000000000000000000, 0.9510565162951535312, 1.000000000000000000, 0.9510565162951535312, 1.000000000000000000, 0.9510565162951535312, 1.000000000000000000, 0.9510565162951535312, 1.000000000000000000, 0.9510565162951535312, 1.000000000000000000, 0.9510565162951535312, 1.000000000000000000, 0.9510565162951535312, 1.000000000000000000, 0.9510565162951535312, 1.000000000000000000, 0.9510565162951535312, 1.000000000000000000, 0.9510565162951535312, 1.000000000000000000, 0.9510565162951535312, 1.000000000000000000, 0.9510565162951535312, 1.000000000000000000, 0.9510565162951535312, 1.000000000000000000, 0.9510565162951535312, 1.000000000000000000, 0.9510565162951535312, 1.000000000000000000, 0.9510565162951535312, 1.000000000000000000, 0.9510565162951535312, 1.000000000000000000, 0.9510565162951535312, 1.000000000000000000, 0.9510565162951535312, 1.000000000000000000, 0.9510565162951535312, 1.000000000000000000, 0.9510565162951535312, 1.000000000000000000, 0.9510565162951535312, 1.000000000000000000, 0.9510565162951535312, 1.000000000000000000, 0.9510565162951535312, 1.000000000000000000, 0.9510565162951535312, 1.000000000000000000, 0.9510565162951535312, 1.000000000000000000, 0.9510565162951535312, 1.000000000000000000, 0.9510565162951535312, 1.000000000000000000, 0.9510565162951535312, 1.000000000000000000, 0.9510565162951535312, 1.000000000000000000, 0.9510565162951535312, 1.000000000000000000, 0.9510565162951535312, 1.000000000000000000, 0.9510565162951535312, 1.000000000000000000, 0.9510565162951535312, 1.000000000000000000, 0.9510565162951535312, 1.000000000000000000, 0.9510565162951535312, 1.000000000000000000, 0.9510565162951535312, 1.000000000000000000, 0.9510565162951535312, 1.000000000000000000, 0.9510565162951535312, 1.000000000000000000, 0.9510565162951535312, 1.000000000000000000, 0.9510565162951535312, 1.000000000000000000, 0.9510565162951535312, 1.000000000000000000, 0.9510565162951535312, 1.000000000000000000, 0.9510565162951535312, 1.000000000000000000, 0.9510565162951535312, 1.000000000000000000, 0.9510565162951535312, 1.000000000000000000, 0.9510565162951535312, 1.000000000000000000, 0.9510565162951535312, 1.000000000000000000, 0.9510565162951535312, 1.000000000000000000, 0.9510565162951535312, 1.000000000000000000, 0.9510565162951535312, 1.000000000000000000, 0.9510565162951535312, 1.000000000000000000, 0.9510565162951535312, 1.000000000000000000, 0.9510565162951535312, 1.000000000000000000, 0.9510565162951535312, 1.000000000000000000, 0.9510565162951535312, 1.000000000000000000, 0.9510565162951535312, 1.000000000000000000, 0.9510565162951535312, 1.000000000000000000, 0.9510565162951535312, 1.000000000000000000, 0.9510565162951535312, 1.000000000000000000, 0.9510565162951535312, 1.000000000000000000, 0.9510565162951535312, 1.000000000000000000, 0.9510565162951535312, 1.000000000000000000, 0.9510565162951535312, 1.000000000000000000, 0.9510565162951535312, 1.000000000000000000, 0.9510565162951535312, 1.000000000000000000, 0.9510565162951535312, 1.000000000000000000, 0.9510565162951535312, 1.000000000000000000, 0.9510565162951535312, 1.000000000000000000, 0.9510565162951535312, 1.000000000000000000, 0.9510565162951535312, 1.000000000000000000, 0.9510565162951535312, 1.000000000000000000, 0.9510565162951535312, 1.000000000000000000, 0.9510565162951535312, 1.000000000000000000, 0.9510565162951535312, 1.000000000000000000, 0.9510565162951535312, 1.000000000000000000, 0.9510565162951535312, 1.000000000000000000, 0.9510565162951535312, 1.000000000000000000, 0.9510565162951535312, 1.000000000000000000, 0.9510565162951535312, 1.000000000000000000, 0.9510565162951535312, 1.000000000000000000, 0.9510565162951535312, 1.000000000000000000, 0.9510565162951535312, 1.000000000000000000, 0.9510565162951535312, 1.000000000000000000, 0.9510565162951535312, 1.000000000000000000, 0.9510565162951535312, 1.000000000000000000, 0.9510565162951535312, 1.000000000000000000, 0.9510565162951535312, 1.000000000000000000, 0.9510565162951535312, 1.000000000000000000, 0.9510565162951535312, 1.000000000000000000, 0.9510565162951535312, 1.000000000000000000, 0.9510565162951535312, 1.000000000000000000, 0.9510565162951535312, 1.000000000000000000, 0.9510565162951535312, 1.000000000000000000) ) ) 
 REPRESENTATION_ITEM ( '' )  SURFACE ( )  );
#8559=CARTESIAN_POINT ( 'NONE',  ( 52.57664461997811856, 45.59948385550240602, -8.007379884777229506 ) ) ;
#8561=CARTESIAN_POINT ( 'NONE',  ( 44.05948171654945611, 46.20051614449766930, -4.345558710429044069 ) ) ;
#8576=CARTESIAN_POINT ( 'NONE',  ( 54.72065718078924590, 56.29948385550240886, 6.458785618021043895 ) ) ;
#8578=CARTESIAN_POINT ( 'NONE',  ( 53.54508667620428497, 50.29948385550240886, 4.840751629271157874 ) ) ;
#8581=CARTESIAN_POINT ( 'NONE',  ( 47.74827507625469281, 64.40051614449765793, -7.007379884777203749 ) ) ;
#8583=CARTESIAN_POINT ( 'NONE',  ( 43.69122665457040000, 50.00051614449765935, -0.02388180880515696977 ) ) ;
#8591=CARTESIAN_POINT ( 'NONE',  ( 42.63976443033212860, 58.99948385550239038, 0.02388180880522514787 ) ) ;
#8601=CARTESIAN_POINT ( 'NONE',  ( 52.25172492374522903, 49.59948385550240602, -7.007379884777225953 ) ) ;
#8603=CARTESIAN_POINT ( 'NONE',  ( 45.90387839640208512, 48.30051614449765651, -5.676469297603124353 ) ) ;
#8622=CARTESIAN_POINT ( 'NONE',  ( 55.71335778527780036, 48.90051614449766504, -1.832500667257213056 ) ) ;
#8626=CARTESIAN_POINT ( 'NONE',  ( 44.30067958973596376, 50.89948385550240317, 1.875703265242204099 ) ) ;
#8628=CARTESIAN_POINT ( 'NONE',  ( 47.37792948025162332, 63.39948385550238896, -7.992620115222770494 ) ) ;
#8629=CARTESIAN_POINT ( 'NONE',  ( 45.27934281921082516, 47.70051614449766220, 6.458785618021089192 ) ) ;
#8646=CARTESIAN_POINT ( 'NONE',  ( 43.33558569842703179, 51.09948385550240602, -2.141517661632099223 ) ) ;
#8648=CARTESIAN_POINT ( 'NONE',  ( 47.37792948025162332, 47.39948385550241028, -7.992620115222770494 ) ) ;
#8650=CARTESIAN_POINT ( 'NONE',  ( 47.70284917648459100, 49.60051614449763946, 6.992620115222796251 ) ) ;
#8666=CARTESIAN_POINT ( 'NONE',  ( 58.41169779390614281, 59.99948385550241170, -0.02388180880523160798 ) ) ;
#8670=CARTESIAN_POINT ( 'NONE',  ( 48.07319477248768180, 48.59948385550239891, 6.007379884777225953 ) ) ;
#8675=CARTESIAN_POINT ( 'NONE',  ( 49.97728705011495265, 49.50051614449766646, 8.000000000000001776 ) ) ;
#8676=CARTESIAN_POINT ( 'NONE',  ( 44.88205777487401349, 49.80051614449765651, 3.688883143319584779 ) ) ;
#8686=CARTESIAN_POINT ( 'NONE',  ( 44.03140696652192787, 57.19948385550238612, -4.306917132069425058 ) ) ;
#8698=CARTESIAN_POINT ( 'NONE',  ( 44.03140696652192787, 53.19948385550238612, -4.306917132069425058 ) ) ;
#8701=CARTESIAN_POINT ( 'NONE',  ( 54.09612160359792199, 45.30051614449766362, 5.676469297603124353 ) ) ;
#8721=CARTESIAN_POINT ( 'NONE',  ( 49.97728705011494554, 47.50051614449765935, 6.000000000000000888 ) ) ;
#8724=CARTESIAN_POINT ( 'NONE',  ( 48.07319477248768180, 50.59948385550240602, 6.007379884777225953 ) ) ;
#8726=CARTESIAN_POINT ( 'NONE',  ( 57.36023556966787851, 49.99948385550238328, -0.02388180880522424582 ) ) ;
#8727=CARTESIAN_POINT ( 'NONE',  ( 54.68390685589039890, 45.30051614449766362, 6.485486291978072693 ) ) ;
#8745=CARTESIAN_POINT ( 'NONE',  ( 47.70284917648453415, 53.39948385550238186, -6.992620115222774047 ) ) ;
#8747=CARTESIAN_POINT ( 'NONE',  ( 43.20883090819745576, 54.79948385550240175, 4.963592699179006473 ) ) ;
#8749=CARTESIAN_POINT ( 'NONE',  ( 47.70284917648459100, 45.60051614449765367, 6.992620115222796251 ) ) ;
#8764=CARTESIAN_POINT ( 'NONE',  ( 54.68390685589033495, 57.69948385550241454, -6.485486291978119766 ) ) ;
#8766=CARTESIAN_POINT ( 'NONE',  ( 53.50833635130540955, 57.69948385550241454, -4.867452303228209765 ) ) ;
#8770=CARTESIAN_POINT ( 'NONE',  ( 52.57664461997821093, 49.40051614449766504, 8.007379884777206414 ) ) ;
#8772=CARTESIAN_POINT ( 'NONE',  ( 43.69122665457040000, 52.00051614449766646, -0.02388180880515696977 ) ) ;
#8797=CARTESIAN_POINT ( 'NONE',  ( 45.86712807150323812, 51.29948385550240175, -5.649768623646098220 ) ) ;
#8800=CARTESIAN_POINT ( 'NONE',  ( 45.86712807150329496, 49.70051614449766220, 5.649768623646139964 ) ) ;
#8810=AXIS2_PLACEMENT_3D ( 'NONE', #18105, #12295, #4666 ) ;
#8812=CARTESIAN_POINT ( 'NONE',  ( 45.90387839640214196, 48.69948385550240744, 5.676469297603166098 ) ) ;
#8821=CARTESIAN_POINT ( 'NONE',  ( 44.91013252490150620, 50.20051614449766220, -3.727524721679154940 ) ) ;
#8826=CARTESIAN_POINT ( 'NONE',  ( 48.07319477248768180, 60.59948385550240602, 6.007379884777225953 ) ) ;
#8828=CARTESIAN_POINT ( 'NONE',  ( 49.97728705011488159, 55.49948385550240459, -7.000000000000000888 ) ) ;
#8829=CARTESIAN_POINT ( 'NONE',  ( 57.60143344285435774, 51.10051614449766078, 2.493737253992045044 ) ) ;
#8834=DIRECTION ( 'NONE',  ( 0.000000000000000000, 0.000000000000000000, 1.000000000000000000 ) ) ;
#8845=CARTESIAN_POINT ( 'NONE',  ( 50.02271294988512551, 56.49948385550240459, 7.000000000000000888 ) ) ;
#8848=CARTESIAN_POINT ( 'NONE',  ( 57.60143344285433642, 55.89948385550241028, -2.493737253992118319 ) ) ;
#8850=CARTESIAN_POINT ( 'NONE',  ( 42.63976443033212860, 46.00051614449766646, -0.02388180880514948964 ) ) ;
#8866=CARTESIAN_POINT ( 'NONE',  ( 53.54508667620428497, 60.29948385550240175, 4.840751629271157874 ) ) ;
#8869=CARTESIAN_POINT ( 'NONE',  ( 57.61547081786810764, 52.90051614449766504, -2.450534656007114176 ) ) ;
#8870=CARTESIAN_POINT ( 'NONE',  ( 46.49166364869456913, 48.30051614449765651, -4.867452303228181343 ) ) ;
#8881=CARTESIAN_POINT ( 'NONE',  ( 43.33558569842703179, 47.09948385550240602, -2.141517661632099223 ) ) ;
#8888=CARTESIAN_POINT ( 'NONE',  ( 54.09612160359786515, 59.69948385550240033, -5.676469297603166098 ) ) ;
#8890=CARTESIAN_POINT ( 'NONE',  ( 47.70284917648459100, 53.60051614449765367, 6.992620115222796251 ) ) ;
#8901=CARTESIAN_POINT ( 'NONE',  ( 49.97728705011486738, 63.49948385550241170, -8.000000000000001776 ) ) ;
#8905=ADVANCED_FACE ( 'NONE', ( #15816 ), #14557, .T. ) ;
#8907=CARTESIAN_POINT ( 'NONE',  ( 54.09612160359792199, 59.30051614449766362, 5.676469297603124353 ) ) ;
#8913=CARTESIAN_POINT ( 'NONE',  ( 43.69122665457040000, 46.00051614449764514, -0.02388180880515696977 ) ) ;
#8918=CARTESIAN_POINT ( 'NONE',  ( 55.11794222512601493, 56.19948385550240744, 3.688883143319541702 ) ) ;
#8920=CARTESIAN_POINT ( 'NONE',  ( 52.29715082351547295, 54.39948385550239607, 6.992620115222774047 ) ) ;
#8921=CARTESIAN_POINT ( 'NONE',  ( 54.68390685589039890, 51.30051614449765651, 6.485486291978072693 ) ) ;
#8938=CARTESIAN_POINT ( 'NONE',  ( 43.33558569842703179, 61.09948385550240602, -2.141517661632099223 ) ) ;
#8940=CARTESIAN_POINT ( 'NONE',  ( 50.02271294988513972, 50.49948385550239749, 8.000000000000001776 ) ) ;
#8942=CARTESIAN_POINT ( 'NONE',  ( 43.33558569842706021, 53.90051614449765793, 2.141517661632167169 ) ) ;
#8958=CARTESIAN_POINT ( 'NONE',  ( 55.69932041026404335, 55.89948385550241028, -1.875703265242203432 ) ) ;
#8961=CARTESIAN_POINT ( 'NONE',  ( 42.39856655714564226, 56.10051614449766078, -2.493737253992044156 ) ) ;
#8962=CARTESIAN_POINT ( 'NONE',  ( 48.02776887271750184, 55.60051614449765367, 5.992620115222795363 ) ) ;
#8972=CARTESIAN_POINT ( 'NONE',  ( 54.13287192849676188, 64.29948385550241596, 5.649768623646098220 ) ) ;
#8976=CARTESIAN_POINT ( 'NONE',  ( 52.29715082351547295, 46.39948385550240317, 6.992620115222774047 ) ) ;
#8981=CARTESIAN_POINT ( 'NONE',  ( 45.31609314410960820, 64.30051614449766362, -6.485486291978072693 ) ) ;
#8984=CARTESIAN_POINT ( 'NONE',  ( 44.05948171654949874, 60.79948385550240886, 4.345558710429105354 ) ) ;
#8986=CARTESIAN_POINT ( 'NONE',  ( 42.63976443033212860, 52.00051614449766646, -0.02388180880514948964 ) ) ;
#8997=CARTESIAN_POINT ( 'NONE',  ( 43.20883090819745576, 62.79948385550240175, 4.963592699179006473 ) ) ;
#9003=CARTESIAN_POINT ( 'NONE',  ( 52.29715082351539479, 56.60051614449766078, -6.992620115222796251 ) ) ;
#9008=CARTESIAN_POINT ( 'NONE',  ( 44.91013252490150620, 56.20051614449766220, -3.727524721679154940 ) ) ;
#9011=CARTESIAN_POINT ( 'NONE',  ( 53.50833635130540955, 57.69948385550241454, -4.867452303228209765 ) ) ;
#9013=CARTESIAN_POINT ( 'NONE',  ( 47.42335538002180328, 56.40051614449765793, -8.007379884777206414 ) ) ;
#9032=CARTESIAN_POINT ( 'NONE',  ( 42.63976443033212860, 56.99948385550241170, 0.02388180880522514787 ) ) ;
#9034=CARTESIAN_POINT ( 'NONE',  ( 58.41169779390614281, 53.99948385550241170, -0.02388180880523160798 ) ) ;
#9036=CARTESIAN_POINT ( 'NONE',  ( 43.33558569842706021, 51.90051614449765793, 2.141517661632167169 ) ) ;
#9055=CARTESIAN_POINT ( 'NONE',  ( 43.69122665457040000, 54.99948385550239749, 0.02388180880521036456 ) ) ;
#9057=CARTESIAN_POINT ( 'NONE',  ( 43.20883090819742023, 52.20051614449766220, -4.963592699178938972 ) ) ;
#9058=CARTESIAN_POINT ( 'NONE',  ( 55.71335778527780036, 54.90051614449765793, -1.832500667257213056 ) ) ;
#9066=CARTESIAN_POINT ( 'NONE',  ( 55.96859303347804371, 62.19948385550240744, 4.306917132069425946 ) ) ;
#9077=CARTESIAN_POINT ( 'NONE',  ( 41.58830220609386430, 46.99948385550239749, 0.02388180880523263147 ) ) ;
#9080=CARTESIAN_POINT ( 'NONE',  ( 55.96859303347804371, 60.19948385550240744, 4.306917132069425946 ) ) ;
#9085=CARTESIAN_POINT ( 'NONE',  ( 55.94051828345053679, 51.20051614449766220, 4.345558710429044069 ) ) ;
#9098=CARTESIAN_POINT ( 'NONE',  ( 57.36023556966787851, 47.99948385550239038, -0.02388180880522424582 ) ) ;
#9106=CARTESIAN_POINT ( 'NONE',  ( 52.25172492374528588, 59.40051614449765793, 7.007379884777204637 ) ) ;
#9111=CARTESIAN_POINT ( 'NONE',  ( 46.49166364869456913, 54.30051614449765651, -4.867452303228181343 ) ) ;
#9115=CARTESIAN_POINT ( 'NONE',  ( 55.08986747509847248, 57.79948385550240175, -3.727524721679197572 ) ) ;
#9118=CARTESIAN_POINT ( 'NONE',  ( 50.02271294988505446, 52.50051614449766646, -8.000000000000001776 ) ) ;
#9130=CARTESIAN_POINT ( 'NONE',  ( 54.09612160359786515, 63.69948385550240744, -5.676469297603166098 ) ) ;
#9134=CARTESIAN_POINT ( 'NONE',  ( 47.74827507625478518, 58.59948385550238470, 7.007379884777227730 ) ) ;
#9136=CARTESIAN_POINT ( 'NONE',  ( 47.42335538002188144, 56.59948385550239891, 8.007379884777233059 ) ) ;
#9139=CARTESIAN_POINT ( 'NONE',  ( 44.05948171654945611, 54.20051614449764799, -4.345558710429044069 ) ) ;
#9149=CARTESIAN_POINT ( 'NONE',  ( 45.86712807150323812, 61.29948385550240886, -5.649768623646098220 ) ) ;
#9156=CARTESIAN_POINT ( 'NONE',  ( 46.49166364869460466, 56.69948385550240744, 4.867452303228209765 ) ) ;
#9159=CARTESIAN_POINT ( 'NONE',  ( 45.27934281921082516, 51.70051614449765509, 6.458785618021089192 ) ) ;
#9161=CARTESIAN_POINT ( 'NONE',  ( 51.97223112728249816, 56.60051614449765367, -5.992620115222793586 ) ) ;
#9175=CARTESIAN_POINT ( 'NONE',  ( 47.74827507625477807, 50.59948385550239891, 7.007379884777229506 ) ) ;
#9180=CARTESIAN_POINT ( 'NONE',  ( 45.27934281921082516, 63.70051614449766930, 6.458785618021089192 ) ) ;
#9182=CARTESIAN_POINT ( 'NONE',  ( 55.96859303347804371, 56.19948385550241454, 4.306917132069425946 ) ) ;
#9184=CARTESIAN_POINT ( 'NONE',  ( 45.90387839640208512, 56.30051614449765651, -5.676469297603124353 ) ) ;
#9191=CARTESIAN_POINT ( 'NONE',  ( 45.31609314410967926, 62.69948385550240744, 6.485486291978119766 ) ) ;
#9195=CARTESIAN_POINT ( 'NONE',  ( 49.97728705011495265, 59.50051614449765935, 7.000000000000000888 ) ) ;
#9200=CARTESIAN_POINT ( 'NONE',  ( 44.30067958973594955, 52.10051614449766788, -1.875703265242155693 ) ) ;
#9205=CARTESIAN_POINT ( 'NONE',  ( 56.30877334542961421, 59.99948385550241170, -0.02388180880520959434 ) ) ;
#9208=CARTESIAN_POINT ( 'NONE',  ( 45.27934281921082516, 53.70051614449766220, 6.458785618021089192 ) ) ;
#9217=CARTESIAN_POINT ( 'NONE',  ( 44.05948171654949874, 62.79948385550240886, 4.345558710429104465 ) ) ;
#9222=CARTESIAN_POINT ( 'NONE',  ( 55.94051828345050836, 59.79948385550238754, -4.345558710429104465 ) ) ;
#9224=CARTESIAN_POINT ( 'NONE',  ( 47.42335538002188144, 60.59948385550240602, 8.007379884777233059 ) ) ;
#9225=CARTESIAN_POINT ( 'NONE',  ( 55.94051828345053679, 53.20051614449766220, 4.345558710429044069 ) ) ;
#9232=CARTESIAN_POINT ( 'NONE',  ( 47.70284917648459810, 45.60051614449765367, 6.992620115222797139 ) ) ;
#9239=CARTESIAN_POINT ( 'NONE',  ( 53.50833635130544508, 45.30051614449766362, 4.867452303228181343 ) ) ;
#9243=CARTESIAN_POINT ( 'NONE',  ( 47.42335538002180328, 50.40051614449766504, -8.007379884777206414 ) ) ;
#9245=CARTESIAN_POINT ( 'NONE',  ( 55.69932041026405045, 55.10051614449765367, 1.875703265242156359 ) ) ;
#9257=CARTESIAN_POINT ( 'NONE',  ( 44.05948171654949874, 52.79948385550240175, 4.345558710429104465 ) ) ;
#9262=CARTESIAN_POINT ( 'NONE',  ( 54.72065718078918906, 62.70051614449766220, -6.458785618021089192 ) ) ;
#9263=CARTESIAN_POINT ( 'NONE',  ( 50.76502259767569569, 44.99999999999998579, -6.467049654501940914 ) ) ;
#9265=CARTESIAN_POINT ( 'NONE',  ( 45.90387839640214196, 56.69948385550240744, 5.676469297603166098 ) ) ;
#9268=CARTESIAN_POINT ( 'NONE',  ( 52.25172492374527877, 53.40051614449765793, 7.007379884777203749 ) ) ;
#9271=CARTESIAN_POINT ( 'NONE',  ( 43.33558569842703179, 53.09948385550240602, -2.141517661632099223 ) ) ;
#9279=CARTESIAN_POINT ( 'NONE',  ( 43.34962307344081012, 50.89948385550241028, 2.184720259617164650 ) ) ;
#9287=CARTESIAN_POINT ( 'NONE',  ( 57.36023556966787851, 57.00051614449766646, 0.02388180880515038476 ) ) ;
#9293=CARTESIAN_POINT ( 'NONE',  ( 55.71335778527780036, 56.90051614449767214, -1.832500667257213056 ) ) ;
#9297=CARTESIAN_POINT ( 'NONE',  ( 53.54508667620424234, 44.70051614449765509, -4.840751629271188961 ) ) ;
#9299=CARTESIAN_POINT ( 'NONE',  ( 47.42335538002180328, 58.40051614449765793, -8.007379884777206414 ) ) ;
#9318=CARTESIAN_POINT ( 'NONE',  ( 49.97728705011488870, 47.49948385550240459, -6.000000000000000888 ) ) ;
#9320=CARTESIAN_POINT ( 'NONE',  ( 57.60143344285433642, 61.89948385550241738, -2.493737253992118319 ) ) ;
#9321=CARTESIAN_POINT ( 'NONE',  ( 47.70284917648459100, 51.60051614449765367, 6.992620115222796251 ) ) ;
#9330=CARTESIAN_POINT ( 'NONE',  ( 55.96859303347802239, 48.80051614449765651, -4.306917132069484566 ) ) ;
#9331=CARTESIAN_POINT ( 'NONE',  ( 47.70284917648453415, 65.39948385550239607, -6.992620115222774047 ) ) ;
#9337=CARTESIAN_POINT ( 'NONE',  ( 51.92680522751233951, 63.59948385550239891, -6.007379884777223289 ) ) ;
#9339=CARTESIAN_POINT ( 'NONE',  ( 47.37792948025170858, 61.60051614449765367, 7.992620115222797139 ) ) ;
#9340=CARTESIAN_POINT ( 'NONE',  ( 46.45491332379576477, 57.70051614449766930, 4.840751629271188961 ) ) ;
#9353=CARTESIAN_POINT ( 'NONE',  ( 43.33558569842703179, 53.09948385550240602, -2.141517661632099223 ) ) ;
#9357=CARTESIAN_POINT ( 'NONE',  ( 54.68390685589033495, 47.69948385550240744, -6.485486291978119766 ) ) ;
#9359=CARTESIAN_POINT ( 'NONE',  ( 47.74827507625478518, 62.59948385550240602, 7.007379884777227730 ) ) ;
#9362=CARTESIAN_POINT ( 'NONE',  ( 56.65037692655921120, 63.10051614449766078, 2.184720259617097593 ) ) ;
#9366=CARTESIAN_POINT ( 'NONE',  ( 50.02271294988512551, 52.49948385550240459, 7.000000000000000888 ) ) ;
#9374=CARTESIAN_POINT ( 'NONE',  ( 50.02271294988512551, 50.49948385550240459, 7.000000000000000888 ) ) ;
#9382=CARTESIAN_POINT ( 'NONE',  ( 45.90387839640208512, 64.30051614449766362, -5.676469297603124353 ) ) ;
#9388=CARTESIAN_POINT ( 'NONE',  ( 56.30877334542961421, 55.00051614449766646, 0.02388180880515774693 ) ) ;
#9394=CARTESIAN_POINT ( 'NONE',  ( 56.79116909180259398, 57.20051614449766220, 4.963592699178938972 ) ) ;
#9418=CARTESIAN_POINT ( 'NONE',  ( 53.54508667620428497, 46.29948385550240886, 4.840751629271157874 ) ) ;
#9421=CARTESIAN_POINT ( 'NONE',  ( 42.38452918213188525, 59.09948385550240602, -2.450534656007040013 ) ) ;
#9422=CARTESIAN_POINT ( 'NONE',  ( 45.86712807150329496, 59.70051614449766220, 5.649768623646139964 ) ) ;
#9430=CARTESIAN_POINT ( 'NONE',  ( 47.70284917648459810, 47.60051614449766078, 6.992620115222797139 ) ) ;
#9431=CARTESIAN_POINT ( 'NONE',  ( 47.70284917648453415, 63.39948385550240317, -6.992620115222774047 ) ) ;
#9437=CARTESIAN_POINT ( 'NONE',  ( 55.11794222512601493, 62.19948385550240744, 3.688883143319541702 ) ) ;
#9439=CARTESIAN_POINT ( 'NONE',  ( 56.65037692655918988, 45.89948385550240317, -2.184720259617163762 ) ) ;
#9441=CARTESIAN_POINT ( 'NONE',  ( 43.20883090819742023, 60.20051614449766220, -4.963592699178938972 ) ) ;
#9443=CARTESIAN_POINT ( 'NONE',  ( 50.02271294988506156, 64.50051614449766646, -6.000000000000000888 ) ) ;
#9456=CARTESIAN_POINT ( 'NONE',  ( 44.05948171654949874, 54.79948385550240886, 4.345558710429104465 ) ) ;
#9460=CARTESIAN_POINT ( 'NONE',  ( 50.02271294988513972, 50.49948385550239749, 8.000000000000001776 ) ) ;
#9462=CARTESIAN_POINT ( 'NONE',  ( 55.69932041026404335, 45.89948385550240317, -1.875703265242203432 ) ) ;
#9465=CARTESIAN_POINT ( 'NONE',  ( 52.29715082351538769, 62.60051614449766078, -6.992620115222796251 ) ) ;
#9467=CARTESIAN_POINT ( 'NONE',  ( 56.66441430157296821, 56.09948385550240602, 2.141517661632100111 ) ) ;
#9473=CARTESIAN_POINT ( 'NONE',  ( 44.03140696652192787, 53.19948385550238612, -4.306917132069425058 ) ) ;
#9481=CARTESIAN_POINT ( 'NONE',  ( 43.33558569842703179, 47.09948385550240602, -2.141517661632099223 ) ) ;
#9484=CARTESIAN_POINT ( 'NONE',  ( 55.69932041026405045, 63.10051614449766078, 1.875703265242156359 ) ) ;
#9488=CARTESIAN_POINT ( 'NONE',  ( 56.79116909180259398, 61.20051614449766220, 4.963592699178938972 ) ) ;
#9506=CARTESIAN_POINT ( 'NONE',  ( 45.90387839640214196, 64.69948385550240744, 5.676469297603166098 ) ) ;
#9508=CARTESIAN_POINT ( 'NONE',  ( 58.41169779390614281, 57.99948385550241170, -0.02388180880523160798 ) ) ;
#9509=CARTESIAN_POINT ( 'NONE',  ( 47.74827507625469281, 60.40051614449767214, -7.007379884777203749 ) ) ;
#9522=CARTESIAN_POINT ( 'NONE',  ( 42.63976443033212149, 46.00051614449765225, -0.02388180880514948964 ) ) ;
#9528=CARTESIAN_POINT ( 'NONE',  ( 53.50833635130540955, 63.69948385550240033, -4.867452303228209765 ) ) ;
#9531=CARTESIAN_POINT ( 'NONE',  ( 58.41169779390614281, 63.00051614449766646, 0.02388180880515032231 ) ) ;
#9533=CARTESIAN_POINT ( 'NONE',  ( 46.49166364869456913, 64.30051614449766362, -4.867452303228181343 ) ) ;
#9545=CARTESIAN_POINT ( 'NONE',  ( 43.33558569842703179, 55.09948385550241312, -2.141517661632099223 ) ) ;
#9549=CARTESIAN_POINT ( 'NONE',  ( 57.60143344285433642, 49.89948385550241028, -2.493737253992118319 ) ) ;
#9552=CARTESIAN_POINT ( 'NONE',  ( 52.29715082351547295, 62.39948385550239607, 6.992620115222774047 ) ) ;
#9555=CARTESIAN_POINT ( 'NONE',  ( 45.90387839640208512, 60.30051614449766362, -5.676469297603124353 ) ) ;
#9557=CARTESIAN_POINT ( 'NONE',  ( 54.13287192849676188, 56.29948385550240175, 5.649768623646098220 ) ) ;
#9566=CARTESIAN_POINT ( 'NONE',  ( 55.96859303347804371, 50.19948385550240744, 4.306917132069425946 ) ) ;
#9573=DIRECTION ( 'NONE',  ( -0.04542589977017699732, 0.9989677110047501252, 0.000000000000000000 ) ) ;
#9577=CARTESIAN_POINT ( 'NONE',  ( 49.97728705011494554, 59.50051614449765935, 6.000000000000000888 ) ) ;
#9581=CARTESIAN_POINT ( 'NONE',  ( 47.37792948025170858, 61.60051614449765367, 7.992620115222797139 ) ) ;
#9597=CARTESIAN_POINT ( 'NONE',  ( 45.90387839640214196, 62.69948385550240744, 5.676469297603166098 ) ) ;
#9600=CARTESIAN_POINT ( 'NONE',  ( 52.62207051974839089, 58.39948385550241028, 7.992620115222770494 ) ) ;
#9601=CARTESIAN_POINT ( 'NONE',  ( 52.29715082351538769, 58.60051614449766078, -6.992620115222796251 ) ) ;
#9602=CARTESIAN_POINT ( 'NONE',  ( 49.97728705011488159, 65.49948385550240459, -7.000000000000000888 ) ) ;
#9623=CARTESIAN_POINT ( 'NONE',  ( 50.02271294988512551, 46.49948385550240459, 7.000000000000000888 ) ) ;
#9626=CARTESIAN_POINT ( 'NONE',  ( 47.37792948025170858, 59.60051614449765367, 7.992620115222797139 ) ) ;
#9627=CARTESIAN_POINT ( 'NONE',  ( 55.08986747509849380, 61.20051614449766220, 3.727524721679155384 ) ) ;
#9631=VERTEX_POINT ( 'NONE', #14689 ) ;
#9641=CARTESIAN_POINT ( 'NONE',  ( 57.36023556966787851, 55.99948385550239749, -0.02388180880522424582 ) ) ;
#9647=CARTESIAN_POINT ( 'NONE',  ( 45.27934281921075410, 53.29948385550240886, -6.458785618021043895 ) ) ;
#9649=CARTESIAN_POINT ( 'NONE',  ( 44.03140696652192787, 63.19948385550240744, -4.306917132069425058 ) ) ;
#9652=CARTESIAN_POINT ( 'NONE',  ( 43.33558569842706021, 59.90051614449766504, 2.141517661632167169 ) ) ;
#9653=CARTESIAN_POINT ( 'NONE',  ( 55.08986747509847248, 63.79948385550241596, -3.727524721679197572 ) ) ;
#9654=CARTESIAN_POINT ( 'NONE',  ( 50.02271294988512551, 56.49948385550240459, 7.000000000000000888 ) ) ;
#9662=CARTESIAN_POINT ( 'NONE',  ( 50.02271294988512551, 54.49948385550240459, 7.000000000000000888 ) ) ;
#9668=CARTESIAN_POINT ( 'NONE',  ( 56.66441430157294690, 62.90051614449765083, -2.141517661632166281 ) ) ;
#9672=CARTESIAN_POINT ( 'NONE',  ( 45.90387839640214196, 46.69948385550240744, 5.676469297603166098 ) ) ;
#9674=CARTESIAN_POINT ( 'NONE',  ( 44.30067958973594955, 64.10051614449766078, -1.875703265242155693 ) ) ;
#9680=CARTESIAN_POINT ( 'NONE',  ( 42.39856655714564226, 58.10051614449765367, -2.493737253992044156 ) ) ;
#9700=CARTESIAN_POINT ( 'NONE',  ( 44.30067958973596376, 46.89948385550240317, 1.875703265242204099 ) ) ;
#9703=CARTESIAN_POINT ( 'NONE',  ( 54.68390685589033495, 63.69948385550240033, -6.485486291978119766 ) ) ;
#9704=CARTESIAN_POINT ( 'NONE',  ( 43.34962307344078880, 64.10051614449766078, -2.184720259617096705 ) ) ;
#9714=CARTESIAN_POINT ( 'NONE',  ( 54.13287192849671214, 54.70051614449766220, -5.649768623646139964 ) ) ;
#9715=CARTESIAN_POINT ( 'NONE',  ( 54.56344682779376143, 44.99999999999996447, -5.899875555194201482 ) ) ;
#9725=CARTESIAN_POINT ( 'NONE',  ( 45.27934281921082516, 57.70051614449766930, 6.458785618021089192 ) ) ;
#9727=CARTESIAN_POINT ( 'NONE',  ( 55.71335778527780036, 62.90051614449765083, -1.832500667257213056 ) ) ;
#9742=CARTESIAN_POINT ( 'NONE',  ( 44.05948171654949874, 56.79948385550239465, 4.345558710429104465 ) ) ;
#9746=CARTESIAN_POINT ( 'NONE',  ( 54.72065718078924590, 52.29948385550240886, 6.458785618021043895 ) ) ;
#9751=CARTESIAN_POINT ( 'NONE',  ( 46.45491332379572924, 51.29948385550240175, -4.840751629271157874 ) ) ;
#9756=CARTESIAN_POINT ( 'NONE',  ( 45.86712807150329496, 61.70051614449766220, 5.649768623646139964 ) ) ;
#9757=CARTESIAN_POINT ( 'NONE',  ( 43.69122665457040000, 62.99948385550241170, 0.02388180880521036456 ) ) ;
#9758=CARTESIAN_POINT ( 'NONE',  ( 55.94051828345050836, 59.79948385550238754, -4.345558710429104465 ) ) ;
#9769=CARTESIAN_POINT ( 'NONE',  ( 45.90387839640214196, 56.69948385550240744, 5.676469297603166098 ) ) ;
#9780=CARTESIAN_POINT ( 'NONE',  ( 51.97223112728249816, 60.60051614449765367, -5.992620115222793586 ) ) ;
#9799=CARTESIAN_POINT ( 'NONE',  ( 44.28664221472220675, 49.09948385550241312, -1.832500667257165317 ) ) ;
#9801=CARTESIAN_POINT ( 'NONE',  ( 50.02271294988513972, 64.49948385550239038, 8.000000000000001776 ) ) ;
#9802=CARTESIAN_POINT ( 'NONE',  ( 43.34962307344078880, 60.10051614449766078, -2.184720259617096705 ) ) ;
#9809=CARTESIAN_POINT ( 'NONE',  ( 43.33558569842706021, 51.90051614449765793, 2.141517661632167169 ) ) ;
#9811=CARTESIAN_POINT ( 'NONE',  ( 55.13865474201621453, 45.00000000000007816, -5.383573523308436748 ) ) ;
#9817=CARTESIAN_POINT ( 'NONE',  ( 56.66441430157296821, 46.09948385550240602, 2.141517661632100111 ) ) ;
#9819=CARTESIAN_POINT ( 'NONE',  ( 45.27934281921082516, 63.70051614449766930, 6.458785618021089192 ) ) ;
#9821=CARTESIAN_POINT ( 'NONE',  ( 56.30877334542961421, 61.00051614449765935, 0.02388180880515774693 ) ) ;
#9832=CARTESIAN_POINT ( 'NONE',  ( 56.66441430157296821, 58.09948385550240602, 2.141517661632100111 ) ) ;
#9836=CARTESIAN_POINT ( 'NONE',  ( 43.20883090819745576, 58.79948385550240175, 4.963592699179006473 ) ) ;
#9839=CARTESIAN_POINT ( 'NONE',  ( 55.71335778527780747, 52.09948385550241312, 1.832500667257165983 ) ) ;
#9842=CARTESIAN_POINT ( 'NONE',  ( 42.38452918213190657, 45.90051614449766504, 2.450534656007115508 ) ) ;
#9843=CARTESIAN_POINT ( 'NONE',  ( 49.97728705011488870, 63.49948385550241170, -6.000000000000000888 ) ) ;
#9856=CARTESIAN_POINT ( 'NONE',  ( 49.97728705011488159, 59.49948385550240459, -7.000000000000000888 ) ) ;
#9869=CARTESIAN_POINT ( 'NONE',  ( 50.02271294988512551, 50.49948385550240459, 7.000000000000000888 ) ) ;
#9871=CARTESIAN_POINT ( 'NONE',  ( 55.71335778527780036, 62.90051614449765083, -1.832500667257213056 ) ) ;
#9878=SHAPE_REPRESENTATION_RELATIONSHIP ( 'NONE' , 'NONE' ,  #1926, #780 ) ;
#9890=CARTESIAN_POINT ( 'NONE',  ( 55.71335778527780747, 64.09948385550239891, 1.832500667257165983 ) ) ;
#9893=CARTESIAN_POINT ( 'NONE',  ( 55.11794222512601493, 50.19948385550241454, 3.688883143319541702 ) ) ;
#9895=CARTESIAN_POINT ( 'NONE',  ( 45.86712807150323812, 49.29948385550240175, -5.649768623646098220 ) ) ;
#9896=CARTESIAN_POINT ( 'NONE',  ( 57.60143344285435774, 45.10051614449766788, 2.493737253992045044 ) ) ;
#9906=CARTESIAN_POINT ( 'NONE',  ( 43.33558569842706021, 55.90051614449765793, 2.141517661632167169 ) ) ;
#9910=ORIENTED_EDGE ( 'NONE', *, *, #1141, .F. ) ;
#9915=CARTESIAN_POINT ( 'NONE',  ( 55.94051828345050836, 49.79948385550240175, -4.345558710429104465 ) ) ;
#9918=CARTESIAN_POINT ( 'NONE',  ( 43.18075615816989199, 49.19948385550240744, -4.924951120819313743 ) ) ;
#9920=CARTESIAN_POINT ( 'NONE',  ( 55.94051828345053679, 51.20051614449766220, 4.345558710429044069 ) ) ;
#9922=CARTESIAN_POINT ( 'NONE',  ( -74.99999999999997158, 45.00000000000001421, 15.00000000000000000 ) ) ;
#9932=CARTESIAN_POINT ( 'NONE',  ( 56.66441430157296821, 56.09948385550240602, 2.141517661632100111 ) ) ;
#9937=CARTESIAN_POINT ( 'NONE',  ( 45.31609314410967926, 56.69948385550240744, 6.485486291978119766 ) ) ;
#9940=CARTESIAN_POINT ( 'NONE',  ( 55.69932041026404335, 53.89948385550240317, -1.875703265242203432 ) ) ;
#9943=CARTESIAN_POINT ( 'NONE',  ( 58.41169779390614281, 47.00051614449766646, 0.02388180880515032231 ) ) ;
#9944=CARTESIAN_POINT ( 'NONE',  ( 43.69122665457040000, 64.99948385550240459, 0.02388180880521036456 ) ) ;
#9953=CARTESIAN_POINT ( 'NONE',  ( 52.25172492374522903, 55.59948385550241312, -7.007379884777225953 ) ) ;
#9961=CARTESIAN_POINT ( 'NONE',  ( 55.94051828345050836, 51.79948385550240175, -4.345558710429104465 ) ) ;
#9963=CARTESIAN_POINT ( 'NONE',  ( 47.74827507625469281, 48.40051614449764372, -7.007379884777203749 ) ) ;
#9988=CARTESIAN_POINT ( 'NONE',  ( 55.08986747509849380, 51.20051614449766220, 3.727524721679155384 ) ) ;
#9993=CARTESIAN_POINT ( 'NONE',  ( 44.30067958973596376, 48.89948385550241028, 1.875703265242204099 ) ) ;
#9995=CARTESIAN_POINT ( 'NONE',  ( 47.74827507625478518, 46.59948385550239891, 7.007379884777227730 ) ) ;
#9997=CARTESIAN_POINT ( 'NONE',  ( 43.20883090819742023, 46.20051614449766220, -4.963592699178938972 ) ) ;
#10007=CARTESIAN_POINT ( 'NONE',  ( 55.96859303347802239, 54.80051614449764941, -4.306917132069484566 ) ) ;
#10015=CARTESIAN_POINT ( 'NONE',  ( 42.63976443033212860, 52.99948385550240459, 0.02388180880522514787 ) ) ;
#10018=CARTESIAN_POINT ( 'NONE',  ( 57.61547081786812896, 46.09948385550240602, 2.450534656007040901 ) ) ;
#10020=CARTESIAN_POINT ( 'NONE',  ( 52.25172492374527877, 45.40051614449766504, 7.007379884777203749 ) ) ;
#10039=CARTESIAN_POINT ( 'NONE',  ( 58.41169779390614281, 61.99948385550241170, -0.02388180880523160798 ) ) ;
#10043=CARTESIAN_POINT ( 'NONE',  ( 43.69122665457040000, 48.99948385550241170, 0.02388180880521036456 ) ) ;
#10048=CARTESIAN_POINT ( 'NONE',  ( 57.61547081786810764, 44.90051614449765793, -2.450534656007114176 ) ) ;
#10049=CARTESIAN_POINT ( 'NONE',  ( 46.45491332379576477, 47.70051614449766220, 4.840751629271188961 ) ) ;
#10057=CARTESIAN_POINT ( 'NONE',  ( 43.34962307344081012, 58.89948385550241028, 2.184720259617164650 ) ) ;
#10069=CARTESIAN_POINT ( 'NONE',  ( 43.34962307344081012, 50.89948385550241028, 2.184720259617164650 ) ) ;
#10071=CARTESIAN_POINT ( 'NONE',  ( 44.05948171654945611, 50.20051614449764088, -4.345558710429044069 ) ) ;
#10092=CARTESIAN_POINT ( 'NONE',  ( 51.97223112728249816, 46.60051614449764656, -5.992620115222793586 ) ) ;
#10095=CARTESIAN_POINT ( 'NONE',  ( 55.69932041026404335, 53.89948385550240317, -1.875703265242203432 ) ) ;
#10097=CARTESIAN_POINT ( 'NONE',  ( 45.86712807150323812, 47.29948385550240886, -5.649768623646098220 ) ) ;
#10098=CARTESIAN_POINT ( 'NONE',  ( 52.57664461997821093, 45.40051614449765793, 8.007379884777206414 ) ) ;
#10116=CARTESIAN_POINT ( 'NONE',  ( 50.02271294988512551, 54.49948385550240459, 7.000000000000000888 ) ) ;
#10118=CARTESIAN_POINT ( 'NONE',  ( 57.60143344285433642, 49.89948385550241028, -2.493737253992118319 ) ) ;
#10120=CARTESIAN_POINT ( 'NONE',  ( 56.65037692655921120, 47.10051614449766078, 2.184720259617097593 ) ) ;
#10133=CARTESIAN_POINT ( 'NONE',  ( 45.31609314410967926, 58.69948385550240033, 6.485486291978119766 ) ) ;
#10135=CARTESIAN_POINT ( 'NONE',  ( 43.69122665457040000, 50.99948385550241170, 0.02388180880521036456 ) ) ;
#10139=CARTESIAN_POINT ( 'NONE',  ( 54.68390685589039890, 49.30051614449766362, 6.485486291978072693 ) ) ;
#10141=CARTESIAN_POINT ( 'NONE',  ( 51.92680522751238925, 47.40051614449765793, 6.007379884777208190 ) ) ;
#10150=CARTESIAN_POINT ( 'NONE',  ( 52.25172492374522903, 57.59948385550241312, -7.007379884777225953 ) ) ;
#10161=CARTESIAN_POINT ( 'NONE',  ( 47.74827507625478518, 52.59948385550239180, 7.007379884777227730 ) ) ;
#10163=CARTESIAN_POINT ( 'NONE',  ( 43.34962307344078880, 46.10051614449766078, -2.184720259617096705 ) ) ;
#10180=CARTESIAN_POINT ( 'NONE',  ( 56.30877334542961421, 49.00051614449765935, 0.02388180880515774693 ) ) ;
#10184=CARTESIAN_POINT ( 'NONE',  ( 46.49166364869460466, 48.69948385550241454, 4.867452303228209765 ) ) ;
#10186=CARTESIAN_POINT ( 'NONE',  ( 55.96859303347804371, 54.19948385550240033, 4.306917132069425946 ) ) ;
#10187=CARTESIAN_POINT ( 'NONE',  ( 49.97728705011495265, 49.50051614449766646, 8.000000000000001776 ) ) ;
#10189=STYLED_ITEM('',(#19468),#2030);
#10202=CARTESIAN_POINT ( 'NONE',  ( 44.03140696652192787, 55.19948385550238612, -4.306917132069425058 ) ) ;
#10205=CARTESIAN_POINT ( 'NONE',  ( 54.72065718078924590, 48.29948385550240175, 6.458785618021043895 ) ) ;
#10207=CARTESIAN_POINT ( 'NONE',  ( 57.36023556966787851, 49.00051614449763804, 0.02388180880515038476 ) ) ;
#10226=CARTESIAN_POINT ( 'NONE',  ( 43.20883090819745576, 56.79948385550240175, 4.963592699179006473 ) ) ;
#10230=CARTESIAN_POINT ( 'NONE',  ( 44.91013252490152752, 54.79948385550240175, 3.727524721679198461 ) ) ;
#10233=CARTESIAN_POINT ( 'NONE',  ( 54.72065718078918906, 46.70051614449766220, -6.458785618021089192 ) ) ;
#10235=CARTESIAN_POINT ( 'NONE',  ( 55.69932041026405045, 51.10051614449766078, 1.875703265242156359 ) ) ;
#10244=CARTESIAN_POINT ( 'NONE',  ( 44.05948171654949874, 64.79948385550240175, 4.345558710429105354 ) ) ;
#10245=CIRCLE ( 'NONE', #544, 0.4999999999999972244 ) ;
#10256=CARTESIAN_POINT ( 'NONE',  ( 47.70284917648453415, 53.39948385550238186, -6.992620115222774047 ) ) ;
#10258=CARTESIAN_POINT ( 'NONE',  ( 57.36023556966787851, 49.00051614449763804, 0.02388180880515038476 ) ) ;
#10268=CARTESIAN_POINT ( 'NONE',  ( 50.02271294988512551, 48.49948385550240459, 7.000000000000000888 ) ) ;
#10282=CARTESIAN_POINT ( 'NONE',  ( 55.08986747509849380, 49.20051614449766220, 3.727524721679155384 ) ) ;
#10286=CARTESIAN_POINT ( 'NONE',  ( 51.97223112728254790, 60.39948385550241028, 5.992620115222778487 ) ) ;
#10288=CARTESIAN_POINT ( 'NONE',  ( 56.66441430157296821, 50.09948385550240602, 2.141517661632100111 ) ) ;
#10289=CARTESIAN_POINT ( 'NONE',  ( 43.20883090819742023, 50.20051614449766220, -4.963592699178938972 ) ) ;
#10305=CARTESIAN_POINT ( 'NONE',  ( 44.05948171654949874, 54.79948385550241596, 4.345558710429105354 ) ) ;
#10307=CARTESIAN_POINT ( 'NONE',  ( 47.42335538002188144, 50.59948385550240602, 8.007379884777233059 ) ) ;
#10309=CARTESIAN_POINT ( 'NONE',  ( 54.09612160359792199, 47.30051614449765651, 5.676469297603124353 ) ) ;
#10322=DIRECTION ( 'NONE',  ( 0.04542589977017006536, -0.9989677110047503472, 0.000000000000000000 ) ) ;
#10326=CARTESIAN_POINT ( 'NONE',  ( 55.71335778527780747, 60.09948385550240602, 1.832500667257165983 ) ) ;
#10329=CARTESIAN_POINT ( 'NONE',  ( 52.57664461997821093, 51.40051614449767214, 8.007379884777206414 ) ) ;
#10331=CARTESIAN_POINT ( 'NONE',  ( 46.49166364869456913, 50.30051614449766362, -4.867452303228181343 ) ) ;
#10343=PLANE ( 'NONE',  #4692 ) ;
#10348=CARTESIAN_POINT ( 'NONE',  ( 47.74827507625477807, 48.59948385550239891, 7.007379884777229506 ) ) ;
#10357=CARTESIAN_POINT ( 'NONE',  ( 43.33558569842703179, 55.09948385550241312, -2.141517661632099223 ) ) ;
#10359=AXIS2_PLACEMENT_3D ( 'NONE', #2871, #8834, #16191 ) ;
#10360=CARTESIAN_POINT ( 'NONE',  ( 47.70284917648459100, 55.60051614449764656, 6.992620115222796251 ) ) ;
#10373=CARTESIAN_POINT ( 'NONE',  ( 44.05948171654949874, 48.79948385550238754, 4.345558710429105354 ) ) ;
#10378=CARTESIAN_POINT ( 'NONE',  ( 45.90387839640208512, 56.30051614449765651, -5.676469297603124353 ) ) ;
#10382=CARTESIAN_POINT ( 'NONE',  ( 46.45491332379576477, 49.70051614449766220, 4.840751629271188961 ) ) ;
#10387=CARTESIAN_POINT ( 'NONE',  ( 48.07319477248768180, 54.59948385550240602, 6.007379884777225953 ) ) ;
#10389=CARTESIAN_POINT ( 'NONE',  ( 56.65037692655918988, 53.89948385550240317, -2.184720259617163762 ) ) ;
#10390=CARTESIAN_POINT ( 'NONE',  ( 56.79116909180259398, 55.20051614449766220, 4.963592699178938972 ) ) ;
#10397=B_SPLINE_CURVE_WITH_KNOTS ( 'NONE', 3,
 ( #13504, #10448, #17932, #3020, #18023, #12310, #4584, #6056, #2925, #9263, #16549, #4490 ),
 .UNSPECIFIED., .F., .F.,
 ( 4, 2, 2, 2, 2, 4 ),
 ( 0.01755862241325779893, 0.01812962329865995884, 0.01870062418406211874, 0.01984262595486643854, 0.02098462772567075835, 0.02212662949647507815 ),
 .UNSPECIFIED. ) ;
#10406=CARTESIAN_POINT ( 'NONE',  ( 54.13287192849676188, 56.29948385550240175, 5.649768623646098220 ) ) ;
#10409=CARTESIAN_POINT ( 'NONE',  ( 52.62207051974839089, 52.39948385550241028, 7.992620115222770494 ) ) ;
#10411=CARTESIAN_POINT ( 'NONE',  ( 45.90387839640208512, 52.30051614449766362, -5.676469297603124353 ) ) ;
#10426=CARTESIAN_POINT ( 'NONE',  ( 55.08986747509847248, 55.79948385550239465, -3.727524721679197572 ) ) ;
#10429=CARTESIAN_POINT ( 'NONE',  ( 54.68390685589039890, 55.30051614449765651, 6.485486291978072693 ) ) ;
#10430=CARTESIAN_POINT ( 'NONE',  ( 44.28664221472221385, 47.90051614449765793, 1.832500667257213722 ) ) ;
#10437=CARTESIAN_POINT ( 'NONE',  ( 56.65037692655918988, 61.89948385550241028, -2.184720259617163762 ) ) ;
#10441=CARTESIAN_POINT ( 'NONE',  ( 54.09612160359786515, 45.69948385550240744, -5.676469297603166098 ) ) ;
#10446=CARTESIAN_POINT ( 'NONE',  ( 43.18075615816989199, 47.19948385550240744, -4.924951120819313743 ) ) ;
#10448=CARTESIAN_POINT ( 'NONE',  ( 54.08601618280673051, 45.00000000000005684, -5.120135501906166731 ) ) ;
#10449=CARTESIAN_POINT ( 'NONE',  ( 47.74827507625478518, 60.59948385550239891, 7.007379884777227730 ) ) ;
#10451=CARTESIAN_POINT ( 'NONE',  ( 45.90387839640208512, 52.30051614449766362, -5.676469297603124353 ) ) ;
#10463=CARTESIAN_POINT ( 'NONE',  ( 49.97728705011488159, 47.49948385550240459, -7.000000000000000888 ) ) ;
#10469=CARTESIAN_POINT ( 'NONE',  ( 47.70284917648459810, 57.60051614449765367, 6.992620115222797139 ) ) ;
#10476=CARTESIAN_POINT ( 'NONE',  ( 55.11794222512599362, 54.80051614449764941, -3.688883143319583446 ) ) ;
#10479=CARTESIAN_POINT ( 'NONE',  ( 44.88205777487398507, 57.19948385550241454, -3.688883143319540814 ) ) ;
#10482=CARTESIAN_POINT ( 'NONE',  ( 56.79116909180259398, 51.20051614449766220, 4.963592699178938972 ) ) ;
#10494=CARTESIAN_POINT ( 'NONE',  ( 56.66441430157296821, 64.09948385550239891, 2.141517661632100111 ) ) ;
#10498=CARTESIAN_POINT ( 'NONE',  ( 57.36023556966787851, 57.99948385550239038, -0.02388180880522424582 ) ) ;
#10500=CARTESIAN_POINT ( 'NONE',  ( 52.62207051974839089, 50.39948385550241738, 7.992620115222770494 ) ) ;
#10502=CARTESIAN_POINT ( 'NONE',  ( 43.33558569842706021, 55.90051614449765793, 2.141517661632167169 ) ) ;
#10513=CARTESIAN_POINT ( 'NONE',  ( 42.63976443033212860, 62.99948385550241170, 0.02388180880522514787 ) ) ;
#10520=CARTESIAN_POINT ( 'NONE',  ( 49.97728705011488870, 55.49948385550241170, -6.000000000000000888 ) ) ;
#10523=CARTESIAN_POINT ( 'NONE',  ( 52.62207051974829852, 56.60051614449765367, -7.992620115222797139 ) ) ;
#10525=CARTESIAN_POINT ( 'NONE',  ( 55.69932041026405045, 53.10051614449767499, 1.875703265242156359 ) ) ;
#10535=CARTESIAN_POINT ( 'NONE',  ( 42.63976443033212149, 48.99948385550241170, 0.02388180880522514787 ) ) ;
#10540=CARTESIAN_POINT ( 'NONE',  ( 47.42335538002180328, 64.40051614449764372, -8.007379884777206414 ) ) ;
#10543=CARTESIAN_POINT ( 'NONE',  ( 44.03140696652192787, 61.19948385550239323, -4.306917132069425058 ) ) ;
#10547=CARTESIAN_POINT ( 'NONE',  ( 43.33558569842706021, 55.90051614449765793, 2.141517661632167169 ) ) ;
#10558=CARTESIAN_POINT ( 'NONE',  ( 41.58830220609386430, 62.99948385550241170, 0.02388180880523263147 ) ) ;
#10564=CARTESIAN_POINT ( 'NONE',  ( 45.90387839640208512, 62.30051614449766362, -5.676469297603124353 ) ) ;
#10569=AXIS2_PLACEMENT_3D ( 'NONE', #6491, #12472, #5218 ) ;
#10571=CARTESIAN_POINT ( 'NONE',  ( 43.69122665457040000, 54.00051614449765935, -0.02388180880515696977 ) ) ;
#10574=CARTESIAN_POINT ( 'NONE',  ( 51.92680522751233951, 57.59948385550240602, -6.007379884777223289 ) ) ;
#10576=CARTESIAN_POINT ( 'NONE',  ( 56.81924384183006538, 52.80051614449766362, -4.924951120819380357 ) ) ;
#10592=CARTESIAN_POINT ( 'NONE',  ( 54.13287192849676188, 64.29948385550241596, 5.649768623646098220 ) ) ;
#10597=CARTESIAN_POINT ( 'NONE',  ( 49.97728705011488159, 61.49948385550240459, -7.000000000000000888 ) ) ;
#10600=CARTESIAN_POINT ( 'NONE',  ( 43.18075615816989199, 51.19948385550240744, -4.924951120819313743 ) ) ;
#10603=CARTESIAN_POINT ( 'NONE',  ( 42.63976443033212860, 56.00051614449765935, -0.02388180880514948964 ) ) ;
#10613=CARTESIAN_POINT ( 'NONE',  ( 47.70284917648453415, 61.39948385550241738, -6.992620115222774047 ) ) ;
#10618=CARTESIAN_POINT ( 'NONE',  ( 44.30067958973596376, 56.89948385550240317, 1.875703265242204099 ) ) ;
#10622=CARTESIAN_POINT ( 'NONE',  ( 42.39856655714564226, 54.10051614449766078, -2.493737253992044156 ) ) ;
#10623=CARTESIAN_POINT ( 'NONE',  ( 53.54508667620424234, 54.70051614449765509, -4.840751629271188961 ) ) ;
#10639=CARTESIAN_POINT ( 'NONE',  ( 44.03140696652193498, 47.19948385550240744, -4.306917132069424170 ) ) ;
#10643=CARTESIAN_POINT ( 'NONE',  ( 57.61547081786810764, 62.90051614449765083, -2.450534656007114176 ) ) ;
#10645=CARTESIAN_POINT ( 'NONE',  ( 55.94051828345050836, 57.79948385550238754, -4.345558710429104465 ) ) ;
#10649=CARTESIAN_POINT ( 'NONE',  ( 55.94051828345053679, 57.20051614449766930, 4.345558710429044069 ) ) ;
#10660=CARTESIAN_POINT ( 'NONE',  ( 45.86712807150323812, 47.29948385550240886, -5.649768623646098220 ) ) ;
#10667=CARTESIAN_POINT ( 'NONE',  ( 50.02271294988505446, 56.50051614449766646, -7.000000000000000888 ) ) ;
#10672=CARTESIAN_POINT ( 'NONE',  ( 46.45491332379576477, 53.70051614449766220, 4.840751629271188961 ) ) ;
#10675=CARTESIAN_POINT ( 'NONE',  ( 55.08986747509847248, 59.79948385550240175, -3.727524721679197572 ) ) ;
#10679=CARTESIAN_POINT ( 'NONE',  ( 57.60143344285435774, 55.10051614449765367, 2.493737253992045044 ) ) ;
#10692=CARTESIAN_POINT ( 'NONE',  ( 52.25172492374522903, 61.59948385550239891, -7.007379884777227730 ) ) ;
#10697=CARTESIAN_POINT ( 'NONE',  ( 56.65037692655918988, 59.89948385550241028, -2.184720259617163762 ) ) ;
#10700=CARTESIAN_POINT ( 'NONE',  ( 45.31609314410967926, 58.69948385550240033, 6.485486291978119766 ) ) ;
#10702=CARTESIAN_POINT ( 'NONE',  ( 55.96859303347802239, 54.80051614449764230, -4.306917132069484566 ) ) ;
#10710=CARTESIAN_POINT ( 'NONE',  ( 55.94051828345054389, 49.20051614449766220, 4.345558710429044957 ) ) ;
#10718=CARTESIAN_POINT ( 'NONE',  ( 55.71335778527780747, 62.09948385550240602, 1.832500667257165983 ) ) ;
#10721=CARTESIAN_POINT ( 'NONE',  ( 47.42335538002180328, 56.40051614449765793, -8.007379884777206414 ) ) ;
#10722=CARTESIAN_POINT ( 'NONE',  ( 55.08986747509849380, 57.20051614449766220, 3.727524721679155384 ) ) ;
#10735=CARTESIAN_POINT ( 'NONE',  ( 50.02271294988512551, 50.49948385550240459, 7.000000000000000888 ) ) ;
#10739=CARTESIAN_POINT ( 'NONE',  ( 57.60143344285433642, 47.89948385550240317, -2.493737253992118319 ) ) ;
#10741=CARTESIAN_POINT ( 'NONE',  ( 45.86712807150323812, 59.29948385550240175, -5.649768623646098220 ) ) ;
#10744=CARTESIAN_POINT ( 'NONE',  ( 49.97728705011495265, 57.50051614449766646, 7.000000000000000888 ) ) ;
#10746=CARTESIAN_POINT ( 'NONE',  ( 47.74827507625478518, 52.59948385550239180, 7.007379884777227730 ) ) ;
#10757=CARTESIAN_POINT ( 'NONE',  ( 43.34962307344081012, 54.89948385550240317, 2.184720259617164650 ) ) ;
#10762=CARTESIAN_POINT ( 'NONE',  ( 55.96859303347802239, 60.80051614449765651, -4.306917132069484566 ) ) ;
#10766=CARTESIAN_POINT ( 'NONE',  ( 48.02776887271750184, 57.60051614449765367, 5.992620115222795363 ) ) ;
#10771=CARTESIAN_POINT ( 'NONE',  ( 55.69932041026405045, 45.10051614449766788, 1.875703265242156359 ) ) ;
#10773=CARTESIAN_POINT ( 'NONE',  ( 58.41169779390614281, 53.00051614449765935, 0.02388180880515032231 ) ) ;
#10787=CARTESIAN_POINT ( 'NONE',  ( 44.88205777487398507, 47.19948385550240744, -3.688883143319540814 ) ) ;
#10789=CARTESIAN_POINT ( 'NONE',  ( 54.68390685589033495, 59.69948385550240744, -6.485486291978119766 ) ) ;
#10790=CARTESIAN_POINT ( 'NONE',  ( 56.66441430157294690, 56.90051614449766504, -2.141517661632166281 ) ) ;
#10798=CARTESIAN_POINT ( 'NONE',  ( 52.25172492374528588, 47.40051614449765793, 7.007379884777204637 ) ) ;
#10805=CARTESIAN_POINT ( 'NONE',  ( 49.97728705011494554, 45.50051614449766646, 6.000000000000000888 ) ) ;
#10807=CARTESIAN_POINT ( 'NONE',  ( 49.97728705011495265, 57.50051614449766646, 8.000000000000001776 ) ) ;
#10810=CARTESIAN_POINT ( 'NONE',  ( 55.71335778527780036, 52.90051614449766504, -1.832500667257213056 ) ) ;
#10826=CARTESIAN_POINT ( 'NONE',  ( 45.90387839640214196, 54.69948385550240744, 5.676469297603166098 ) ) ;
#10830=CARTESIAN_POINT ( 'NONE',  ( 42.38452918213188525, 49.09948385550241312, -2.450534656007040013 ) ) ;
#10833=CARTESIAN_POINT ( 'NONE',  ( 49.97728705011488159, 63.49948385550241170, -7.000000000000000888 ) ) ;
#10838=CARTESIAN_POINT ( 'NONE',  ( 56.66441430157294690, 62.90051614449765083, -2.141517661632166281 ) ) ;
#10840=CARTESIAN_POINT ( 'NONE',  ( 55.94051828345050836, 49.79948385550240175, -4.345558710429104465 ) ) ;
#10847=CARTESIAN_POINT ( 'NONE',  ( 52.29715082351547295, 52.39948385550241738, 6.992620115222774047 ) ) ;
#10858=CARTESIAN_POINT ( 'NONE',  ( 51.97223112728249816, 54.60051614449766788, -5.992620115222793586 ) ) ;
#10863=CARTESIAN_POINT ( 'NONE',  ( 57.60143344285435774, 61.10051614449766788, 2.493737253992045044 ) ) ;
#10880=CARTESIAN_POINT ( 'NONE',  ( 45.86712807150323812, 63.29948385550240886, -5.649768623646098220 ) ) ;
#10884=CARTESIAN_POINT ( 'NONE',  ( 42.63976443033212860, 64.99948385550240459, 0.02388180880522514787 ) ) ;
#10886=CARTESIAN_POINT ( 'NONE',  ( 43.20883090819745576, 62.79948385550240175, 4.963592699179006473 ) ) ;
#10887=CARTESIAN_POINT ( 'NONE',  ( 56.65037692655921120, 63.10051614449766078, 2.184720259617097593 ) ) ;
#10895=CARTESIAN_POINT ( 'NONE',  ( 44.05948171654949874, 62.79948385550241596, 4.345558710429105354 ) ) ;
#10902=CARTESIAN_POINT ( 'NONE',  ( 55.69932041026404335, 61.89948385550241738, -1.875703265242203432 ) ) ;
#10904=CARTESIAN_POINT ( 'NONE',  ( 54.13287192849676188, 48.29948385550240175, 5.649768623646098220 ) ) ;
#10906=CARTESIAN_POINT ( 'NONE',  ( 58.41169779390614281, 57.00051614449766646, 0.02388180880515032231 ) ) ;
#10907=CARTESIAN_POINT ( 'NONE',  ( 53.50833635130544508, 55.30051614449765651, 4.867452303228181343 ) ) ;
#10921=CARTESIAN_POINT ( 'NONE',  ( 49.97728705011488159, 55.49948385550240459, -7.000000000000000888 ) ) ;
#10926=CARTESIAN_POINT ( 'NONE',  ( 47.42335538002188144, 50.59948385550240602, 8.007379884777233059 ) ) ;
#10928=CARTESIAN_POINT ( 'NONE',  ( 49.97728705011488159, 65.49948385550240459, -7.000000000000000888 ) ) ;
#10931=CARTESIAN_POINT ( 'NONE',  ( 45.86712807150329496, 63.70051614449766220, 5.649768623646139964 ) ) ;
#10936=CARTESIAN_POINT ( 'NONE',  ( 45.90387839640214196, 60.69948385550240033, 5.676469297603166098 ) ) ;
#10944=CARTESIAN_POINT ( 'NONE',  ( 54.09612160359786515, 51.69948385550240744, -5.676469297603166098 ) ) ;
#10954=CARTESIAN_POINT ( 'NONE',  ( 52.25172492374522903, 45.59948385550240602, -7.007379884777225953 ) ) ;
#10958=CARTESIAN_POINT ( 'NONE',  ( 55.71335778527780036, 60.90051614449766504, -1.832500667257213056 ) ) ;
#10964=CARTESIAN_POINT ( 'NONE',  ( 58.41169779390614281, 59.00051614449766646, 0.02388180880515032231 ) ) ;
#10985=CARTESIAN_POINT ( 'NONE',  ( 52.29715082351547295, 64.39948385550239607, 6.992620115222774047 ) ) ;
#10987=CARTESIAN_POINT ( 'NONE',  ( 42.39856655714566358, 56.89948385550240317, 2.493737253992119207 ) ) ;
#10988=CARTESIAN_POINT ( 'NONE',  ( 56.65037692655921120, 61.10051614449766078, 2.184720259617097593 ) ) ;
#11004=CARTESIAN_POINT ( 'NONE',  ( 44.30067958973596376, 62.89948385550240317, 1.875703265242204099 ) ) ;
#11006=CARTESIAN_POINT ( 'NONE',  ( 43.33558569842703179, 47.09948385550240602, -2.141517661632099223 ) ) ;
#11008=CARTESIAN_POINT ( 'NONE',  ( 47.42335538002180328, 62.40051614449765793, -8.007379884777206414 ) ) ;
#11009=CARTESIAN_POINT ( 'NONE',  ( 56.65037692655921120, 45.10051614449766078, 2.184720259617097593 ) ) ;
#11020=CARTESIAN_POINT ( 'NONE',  ( 42.63976443033212149, 54.99948385550239749, 0.02388180880522514787 ) ) ;
#11025=CARTESIAN_POINT ( 'NONE',  ( 43.18075615816989199, 53.19948385550240744, -4.924951120819313743 ) ) ;
#11027=CARTESIAN_POINT ( 'NONE',  ( 46.49166364869460466, 46.69948385550240744, 4.867452303228209765 ) ) ;
#11030=CARTESIAN_POINT ( 'NONE',  ( 43.34962307344078880, 62.10051614449766078, -2.184720259617096705 ) ) ;
#11031=CARTESIAN_POINT ( 'NONE',  ( 42.63976443033212860, 58.99948385550239038, 0.02388180880522514787 ) ) ;
#11039=CARTESIAN_POINT ( 'NONE',  ( 42.63976443033212860, 48.99948385550240459, 0.02388180880522514787 ) ) ;
#11048=CARTESIAN_POINT ( 'NONE',  ( 49.97728705011488159, 45.49948385550240459, -7.000000000000000888 ) ) ;
#11051=CARTESIAN_POINT ( 'NONE',  ( 44.88205777487401349, 61.80051614449766362, 3.688883143319584779 ) ) ;
#11053=EDGE_CURVE ( 'NONE', #9631, #11812, #15313, .T. ) ;
#11056=CARTESIAN_POINT ( 'NONE',  ( 49.97728705011495265, 61.50051614449766646, 8.000000000000001776 ) ) ;
#11067=EDGE_CURVE ( 'NONE', #7311, #2212, #5996, .T. ) ;
#11077=CARTESIAN_POINT ( 'NONE',  ( 51.97223112728254790, 46.39948385550240317, 5.992620115222778487 ) ) ;
#11079=CARTESIAN_POINT ( 'NONE',  ( 54.72065718078924590, 60.29948385550240175, 6.458785618021043895 ) ) ;
#11080=CARTESIAN_POINT ( 'NONE',  ( 54.09612160359792199, 63.30051614449766362, 5.676469297603124353 ) ) ;
#11094=CARTESIAN_POINT ( 'NONE',  ( 57.36023556966787851, 47.99948385550239038, -0.02388180880522424582 ) ) ;
#11097=CARTESIAN_POINT ( 'NONE',  ( 45.31609314410960820, 60.30051614449767072, -6.485486291978072693 ) ) ;
#11099=CARTESIAN_POINT ( 'NONE',  ( 46.45491332379576477, 61.70051614449766220, 4.840751629271188961 ) ) ;
#11111=CARTESIAN_POINT ( 'NONE',  ( 56.65037692655918988, 51.89948385550241028, -2.184720259617163762 ) ) ;
#11116=CARTESIAN_POINT ( 'NONE',  ( 52.62207051974839089, 52.39948385550241028, 7.992620115222770494 ) ) ;
#11120=CARTESIAN_POINT ( 'NONE',  ( 43.69122665457040000, 46.99948385550239749, 0.02388180880521036456 ) ) ;
#11123=CARTESIAN_POINT ( 'NONE',  ( 55.94051828345053679, 59.20051614449766220, 4.345558710429044069 ) ) ;
#11124=CARTESIAN_POINT ( 'NONE',  ( 49.97728705011488870, 61.49948385550241170, -6.000000000000000888 ) ) ;
#11126=CARTESIAN_POINT ( 'NONE',  ( 54.09612160359786515, 57.69948385550240744, -5.676469297603166098 ) ) ;
#11132=CARTESIAN_POINT ( 'NONE',  ( 57.36023556966787851, 53.99948385550239038, -0.02388180880522424582 ) ) ;
#11141=CARTESIAN_POINT ( 'NONE',  ( 57.36023556966787851, 45.99948385550238328, -0.02388180880522424582 ) ) ;
#11143=CARTESIAN_POINT ( 'NONE',  ( 44.91013252490150620, 62.20051614449766220, -3.727524721679154940 ) ) ;
#11147=CARTESIAN_POINT ( 'NONE',  ( 54.72065718078918906, 60.70051614449766930, -6.458785618021089192 ) ) ;
#11166=CARTESIAN_POINT ( 'NONE',  ( 44.05948171654949874, 64.79948385550240175, 4.345558710429105354 ) ) ;
#11169=CARTESIAN_POINT ( 'NONE',  ( 44.05948171654949874, 46.79948385550238754, 4.345558710429105354 ) ) ;
#11170=CARTESIAN_POINT ( 'NONE',  ( 52.25172492374527877, 61.40051614449765083, 7.007379884777203749 ) ) ;
#11183=CARTESIAN_POINT ( 'NONE',  ( 43.34962307344078880, 50.10051614449766078, -2.184720259617096705 ) ) ;
#11195=CARTESIAN_POINT ( 'NONE',  ( 52.62207051974829852, 60.60051614449765367, -7.992620115222797139 ) ) ;
#11196=CARTESIAN_POINT ( 'NONE',  ( 46.49166364869456913, 62.30051614449766362, -4.867452303228181343 ) ) ;
#11211=CARTESIAN_POINT ( 'NONE',  ( 44.03140696652193498, 59.19948385550240033, -4.306917132069424170 ) ) ;
#11215=CARTESIAN_POINT ( 'NONE',  ( 57.61547081786812896, 50.09948385550240602, 2.450534656007040901 ) ) ;
#11217=CARTESIAN_POINT ( 'NONE',  ( 47.70284917648453415, 63.39948385550240317, -6.992620115222774047 ) ) ;
#11220=CARTESIAN_POINT ( 'NONE',  ( 52.25172492374527877, 61.40051614449765083, 7.007379884777203749 ) ) ;
#11221=CARTESIAN_POINT ( 'NONE',  ( 46.45491332379576477, 45.70051614449766220, 4.840751629271188961 ) ) ;
#11222=CARTESIAN_POINT ( 'NONE',  ( 45.90387839640214196, 56.69948385550240744, 5.676469297603166098 ) ) ;
#11224=CARTESIAN_POINT ( 'NONE',  ( 49.99999999999997158, 45.00000000000001421, -6.500000000000004441 ) ) ;
#11231=CARTESIAN_POINT ( 'NONE',  ( 44.03140696652192787, 61.19948385550239323, -4.306917132069425058 ) ) ;
#11242=CARTESIAN_POINT ( 'NONE',  ( 56.66441430157296821, 48.09948385550240602, 2.141517661632100111 ) ) ;
#11244=CARTESIAN_POINT ( 'NONE',  ( 51.92680522751238925, 59.40051614449765793, 6.007379884777208190 ) ) ;
#11265=CARTESIAN_POINT ( 'NONE',  ( 50.02271294988511841, 48.49948385550241170, 6.000000000000000888 ) ) ;
#11269=CARTESIAN_POINT ( 'NONE',  ( 56.66441430157296821, 48.09948385550240602, 2.141517661632100111 ) ) ;
#11271=CARTESIAN_POINT ( 'NONE',  ( 50.02271294988505446, 60.50051614449765935, -7.000000000000000888 ) ) ;
#11283=CARTESIAN_POINT ( 'NONE',  ( 49.97728705011495265, 53.50051614449765935, 7.000000000000000888 ) ) ;
#11284=CARTESIAN_POINT ( 'NONE',  ( 52.07576163693497051, 45.00000000000001421, -7.275735003127095979 ) ) ;
#11292=CARTESIAN_POINT ( 'NONE',  ( 44.05948171654949874, 48.79948385550238754, 4.345558710429105354 ) ) ;
#11295=CARTESIAN_POINT ( 'NONE',  ( 42.39856655714566358, 48.89948385550241028, 2.493737253992119207 ) ) ;
#11298=CARTESIAN_POINT ( 'NONE',  ( 44.28664221472221385, 59.90051614449767214, 1.832500667257213722 ) ) ;
#11300=DIRECTION ( 'NONE',  ( 0.000000000000000000, -0.000000000000000000, 1.000000000000000000 ) ) ;
#11313=CARTESIAN_POINT ( 'NONE',  ( 57.36023556966787851, 57.99948385550240459, -0.02388180880522424582 ) ) ;
#11317=CARTESIAN_POINT ( 'NONE',  ( 56.79116909180255135, 51.79948385550240175, -4.963592699179005585 ) ) ;
#11320=CARTESIAN_POINT ( 'NONE',  ( 44.91013252490152752, 48.79948385550240175, 3.727524721679198461 ) ) ;
#11324=CARTESIAN_POINT ( 'NONE',  ( 43.18075615816994173, 47.80051614449764941, 4.924951120819380357 ) ) ;
#11326=CARTESIAN_POINT ( 'NONE',  ( 51.92680522751238925, 45.40051614449765793, 6.007379884777208190 ) ) ;
#11334=CARTESIAN_POINT ( 'NONE',  ( 54.13287192849676188, 58.29948385550240175, 5.649768623646098220 ) ) ;
#11342=CARTESIAN_POINT ( 'NONE',  ( 43.34962307344081012, 52.89948385550240317, 2.184720259617164650 ) ) ;
#11345=CARTESIAN_POINT ( 'NONE',  ( 50.02271294988506156, 62.50051614449767357, -6.000000000000000888 ) ) ;
#11361=CARTESIAN_POINT ( 'NONE',  ( 54.23491683972284960, 45.00000000000001421, -4.999999999999999112 ) ) ;
#11363=CARTESIAN_POINT ( 'NONE',  ( 46.45491332379572924, 61.29948385550240886, -4.840751629271157874 ) ) ;
#11367=CARTESIAN_POINT ( 'NONE',  ( 46.45491332379572924, 51.29948385550240175, -4.840751629271157874 ) ) ;
#11369=CARTESIAN_POINT ( 'NONE',  ( 49.97728705011488159, 47.49948385550240459, -7.000000000000000888 ) ) ;
#11370=CARTESIAN_POINT ( 'NONE',  ( 50.02271294988505446, 50.50051614449765935, -8.000000000000001776 ) ) ;
#11378=CARTESIAN_POINT ( 'NONE',  ( 45.86712807150329496, 55.70051614449766220, 5.649768623646139964 ) ) ;
#11386=CARTESIAN_POINT ( 'NONE',  ( 44.05948171654949874, 50.79948385550238754, 4.345558710429105354 ) ) ;
#11388=CARTESIAN_POINT ( 'NONE',  ( 43.18075615816989199, 47.19948385550240744, -4.924951120819313743 ) ) ;
#11390=CARTESIAN_POINT ( 'NONE',  ( 54.09612160359792199, 45.30051614449766362, 5.676469297603124353 ) ) ;
#11404=CARTESIAN_POINT ( 'NONE',  ( 47.74827507625477807, 56.59948385550240602, 7.007379884777229506 ) ) ;
#11409=CARTESIAN_POINT ( 'NONE',  ( 52.57664461997811856, 57.59948385550240602, -8.007379884777229506 ) ) ;
#11413=CARTESIAN_POINT ( 'NONE',  ( 50.02271294988511841, 50.49948385550239749, 6.000000000000000888 ) ) ;
#11416=CARTESIAN_POINT ( 'NONE',  ( 43.20883090819742023, 48.20051614449766930, -4.963592699178938972 ) ) ;
#11419=CARTESIAN_POINT ( 'NONE',  ( 53.50833635130540955, 63.69948385550240033, -4.867452303228209765 ) ) ;
#11428=CARTESIAN_POINT ( 'NONE',  ( 50.02271294988512551, 60.49948385550240459, 7.000000000000000888 ) ) ;
#11439=CARTESIAN_POINT ( 'NONE',  ( 54.09612160359786515, 49.69948385550240744, -5.676469297603166098 ) ) ;
#11441=CARTESIAN_POINT ( 'NONE',  ( 47.74827507625469281, 46.40051614449764372, -7.007379884777203749 ) ) ;
#11457=CARTESIAN_POINT ( 'NONE',  ( 50.02271294988506156, 50.50051614449765935, -6.000000000000000888 ) ) ;
#11460=CARTESIAN_POINT ( 'NONE',  ( 48.02776887271745210, 49.39948385550241028, -5.992620115222778487 ) ) ;
#11462=CARTESIAN_POINT ( 'NONE',  ( 54.13287192849676188, 46.29948385550240886, 5.649768623646098220 ) ) ;
#11463=CARTESIAN_POINT ( 'NONE',  ( 56.81924384183006538, 46.80051614449766362, -4.924951120819380357 ) ) ;
#11475=CARTESIAN_POINT ( 'NONE',  ( 57.36023556966787851, 53.00051614449765225, 0.02388180880515038476 ) ) ;
#11482=CARTESIAN_POINT ( 'NONE',  ( 55.96859303347804371, 52.19948385550240033, 4.306917132069425946 ) ) ;
#11484=CARTESIAN_POINT ( 'NONE',  ( 57.60143344285433642, 47.89948385550240317, -2.493737253992118319 ) ) ;
#11486=CARTESIAN_POINT ( 'NONE',  ( 45.90387839640208512, 50.30051614449766362, -5.676469297603124353 ) ) ;
#11499=CARTESIAN_POINT ( 'NONE',  ( 56.66441430157296821, 60.09948385550240602, 2.141517661632100111 ) ) ;
#11504=CARTESIAN_POINT ( 'NONE',  ( 45.27934281921075410, 61.29948385550240886, -6.458785618021043895 ) ) ;
#11507=CARTESIAN_POINT ( 'NONE',  ( 56.30877334542961421, 49.99948385550240459, -0.02388180880520959434 ) ) ;
#11510=CARTESIAN_POINT ( 'NONE',  ( 47.37792948025170858, 47.60051614449766078, 7.992620115222797139 ) ) ;
#11511=CARTESIAN_POINT ( 'NONE',  ( 55.08986747509849380, 47.20051614449766220, 3.727524721679155384 ) ) ;
#11522=CARTESIAN_POINT ( 'NONE',  ( 44.05948171654949874, 58.79948385550240886, 4.345558710429105354 ) ) ;
#11532=CARTESIAN_POINT ( 'NONE',  ( 49.97728705011488159, 51.49948385550240459, -7.000000000000000888 ) ) ;
#11536=CARTESIAN_POINT ( 'NONE',  ( 47.74827507625469281, 50.40051614449764372, -7.007379884777203749 ) ) ;
#11557=CARTESIAN_POINT ( 'NONE',  ( 44.88205777487401349, 51.80051614449766362, 3.688883143319584779 ) ) ;
#11560=CARTESIAN_POINT ( 'NONE',  ( 43.69122665457040000, 50.99948385550241170, 0.02388180880521036456 ) ) ;
#11562=CARTESIAN_POINT ( 'NONE',  ( 52.29715082351547295, 48.39948385550240317, 6.992620115222774047 ) ) ;
#11564=CARTESIAN_POINT ( 'NONE',  ( 42.38452918213190657, 45.90051614449766504, 2.450534656007115508 ) ) ;
#11575=CARTESIAN_POINT ( 'NONE',  ( 55.96859303347802239, 52.80051614449765651, -4.306917132069484566 ) ) ;
#11585=CARTESIAN_POINT ( 'NONE',  ( 45.90387839640214196, 52.69948385550240033, 5.676469297603166098 ) ) ;
#11587=CARTESIAN_POINT ( 'NONE',  ( 49.97728705011486738, 49.49948385550241170, -8.000000000000001776 ) ) ;
#11590=CARTESIAN_POINT ( 'NONE',  ( 52.25172492374527877, 49.40051614449766504, 7.007379884777203749 ) ) ;
#11606=CARTESIAN_POINT ( 'NONE',  ( 50.02271294988513972, 60.49948385550240459, 8.000000000000001776 ) ) ;
#11610=CARTESIAN_POINT ( 'NONE',  ( 55.69932041026404335, 47.89948385550240317, -1.875703265242203432 ) ) ;
#11614=CARTESIAN_POINT ( 'NONE',  ( 52.62207051974829852, 48.60051614449766788, -7.992620115222797139 ) ) ;
#11615=CARTESIAN_POINT ( 'NONE',  ( 56.30877334542961421, 49.00051614449765935, 0.02388180880515774693 ) ) ;
#11622=CARTESIAN_POINT ( 'NONE',  ( 43.33558569842703179, 57.09948385550240602, -2.141517661632099223 ) ) ;
#11635=CARTESIAN_POINT ( 'NONE',  ( 56.66441430157296821, 52.09948385550240602, 2.141517661632100111 ) ) ;
#11637=CARTESIAN_POINT ( 'NONE',  ( 45.86712807150329496, 45.70051614449766220, 5.649768623646139964 ) ) ;
#11657=CARTESIAN_POINT ( 'NONE',  ( 43.69122665457040000, 48.00051614449766646, -0.02388180880515696977 ) ) ;
#11661=CARTESIAN_POINT ( 'NONE',  ( 44.30067958973596376, 52.89948385550241028, 1.875703265242204099 ) ) ;
#11663=CARTESIAN_POINT ( 'NONE',  ( 45.86712807150323812, 53.29948385550240886, -5.649768623646098220 ) ) ;
#11664=CARTESIAN_POINT ( 'NONE',  ( 58.41169779390614281, 49.00051614449765935, 0.02388180880515032231 ) ) ;
#11683=CARTESIAN_POINT ( 'NONE',  ( 56.65037692655918988, 53.89948385550240317, -2.184720259617163762 ) ) ;
#11685=CARTESIAN_POINT ( 'NONE',  ( 54.72065718078924590, 50.29948385550240886, 6.458785618021043895 ) ) ;
#11686=CARTESIAN_POINT ( 'NONE',  ( 55.94051828345053679, 47.20051614449766220, 4.345558710429044069 ) ) ;
#11698=CARTESIAN_POINT ( 'NONE',  ( 57.60143344285433642, 61.89948385550241738, -2.493737253992118319 ) ) ;
#11700=CARTESIAN_POINT ( 'NONE',  ( 46.45491332379572924, 49.29948385550240886, -4.840751629271157874 ) ) ;
#11704=CARTESIAN_POINT ( 'NONE',  ( 43.34962307344078880, 64.10051614449766078, -2.184720259617096705 ) ) ;
#11706=CARTESIAN_POINT ( 'NONE',  ( 51.97223112728249816, 46.60051614449764656, -5.992620115222793586 ) ) ;
#11721=CARTESIAN_POINT ( 'NONE',  ( 54.09612160359786515, 47.69948385550240744, -5.676469297603166098 ) ) ;
#11727=CARTESIAN_POINT ( 'NONE',  ( 47.74827507625478518, 50.59948385550238470, 7.007379884777227730 ) ) ;
#11729=CARTESIAN_POINT ( 'NONE',  ( 54.09612160359792199, 49.30051614449765651, 5.676469297603124353 ) ) ;
#11739=CARTESIAN_POINT ( 'NONE',  ( 55.96859303347804371, 48.19948385550240033, 4.306917132069425946 ) ) ;
#11747=CARTESIAN_POINT ( 'NONE',  ( 55.08986747509849380, 47.20051614449766220, 3.727524721679155384 ) ) ;
#11751=CARTESIAN_POINT ( 'NONE',  ( 46.49166364869460466, 58.69948385550240033, 4.867452303228209765 ) ) ;
#11753=CARTESIAN_POINT ( 'NONE',  ( 43.33558569842703179, 55.09948385550241312, -2.141517661632099223 ) ) ;
#11754=CARTESIAN_POINT ( 'NONE',  ( 42.39856655714564226, 50.10051614449766078, -2.493737253992044156 ) ) ;
#11773=CARTESIAN_POINT ( 'NONE',  ( 43.34962307344081012, 48.89948385550240317, 2.184720259617164650 ) ) ;
#11777=CARTESIAN_POINT ( 'NONE',  ( 45.27934281921075410, 55.29948385550240175, -6.458785618021043895 ) ) ;
#11779=CARTESIAN_POINT ( 'NONE',  ( 54.13287192849671214, 50.70051614449766220, -5.649768623646139964 ) ) ;
#11797=CARTESIAN_POINT ( 'NONE',  ( 54.72065718078924590, 62.29948385550241596, 6.458785618021043895 ) ) ;
#11801=CARTESIAN_POINT ( 'NONE',  ( 49.97728705011488870, 59.49948385550240459, -6.000000000000000888 ) ) ;
#11805=CARTESIAN_POINT ( 'NONE',  ( 50.02271294988505446, 54.50051614449765935, -8.000000000000001776 ) ) ;
#11806=CARTESIAN_POINT ( 'NONE',  ( 44.88205777487401349, 51.80051614449766362, 3.688883143319584779 ) ) ;
#11812=VERTEX_POINT ( 'NONE', #19193 ) ;
#11815=CARTESIAN_POINT ( 'NONE',  ( 42.63976443033212860, 64.99948385550240459, 0.02388180880522514787 ) ) ;
#11820=CARTESIAN_POINT ( 'NONE',  ( 56.65037692655918988, 45.89948385550240317, -2.184720259617163762 ) ) ;
#11827=CARTESIAN_POINT ( 'NONE',  ( 52.25172492374522903, 59.59948385550240602, -7.007379884777225953 ) ) ;
#11829=CARTESIAN_POINT ( 'NONE',  ( 54.13287192849671214, 46.70051614449766220, -5.649768623646139964 ) ) ;
#11839=CARTESIAN_POINT ( 'NONE',  ( 49.97728705011488159, 45.49948385550240459, -7.000000000000000888 ) ) ;
#11850=CARTESIAN_POINT ( 'NONE',  ( 46.49166364869456913, 46.30051614449766362, -4.867452303228181343 ) ) ;
#11853=CARTESIAN_POINT ( 'NONE',  ( 44.30067958973596376, 58.89948385550241028, 1.875703265242204099 ) ) ;
#11855=CARTESIAN_POINT ( 'NONE',  ( 45.90387839640214196, 50.69948385550240744, 5.676469297603166098 ) ) ;
#11856=CARTESIAN_POINT ( 'NONE',  ( 54.72065718078918906, 56.70051614449766930, -6.458785618021089192 ) ) ;
#11873=CARTESIAN_POINT ( 'NONE',  ( 45.86712807150323812, 59.29948385550240175, -5.649768623646098220 ) ) ;
#11875=CARTESIAN_POINT ( 'NONE',  ( 54.72065718078924590, 56.29948385550240886, 6.458785618021043895 ) ) ;
#11877=CARTESIAN_POINT ( 'NONE',  ( 54.13287192849671214, 52.70051614449766220, -5.649768623646139964 ) ) ;
#11895=CARTESIAN_POINT ( 'NONE',  ( 50.02271294988511841, 56.49948385550240459, 6.000000000000000888 ) ) ;
#11898=CARTESIAN_POINT ( 'NONE',  ( 42.38452918213190657, 55.90051614449766504, 2.450534656007115508 ) ) ;
#11900=CARTESIAN_POINT ( 'NONE',  ( 51.92680522751238925, 49.40051614449766504, 6.007379884777208190 ) ) ;
#11913=CARTESIAN_POINT ( 'NONE',  ( 52.29715082351547295, 62.39948385550239607, 6.992620115222774047 ) ) ;
#11923=CARTESIAN_POINT ( 'NONE',  ( 58.41169779390614281, 47.99948385550239038, -0.02388180880523160798 ) ) ;
#11927=CARTESIAN_POINT ( 'NONE',  ( 57.36023556966787851, 55.99948385550239038, -0.02388180880522424582 ) ) ;
#11931=CARTESIAN_POINT ( 'NONE',  ( 50.02271294988505446, 56.50051614449766646, -7.000000000000000888 ) ) ;
#11943=CARTESIAN_POINT ( 'NONE',  ( 56.65037692655918988, 45.89948385550240317, -2.184720259617163762 ) ) ;
#11949=CARTESIAN_POINT ( 'NONE',  ( 56.66441430157294690, 56.90051614449766504, -2.141517661632166281 ) ) ;
#11954=CARTESIAN_POINT ( 'NONE',  ( 43.69122665457040000, 56.00051614449765935, -0.02388180880515696977 ) ) ;
#11959=CARTESIAN_POINT ( 'NONE',  ( 55.69932041026404335, 57.89948385550241028, -1.875703265242203432 ) ) ;
#11961=CARTESIAN_POINT ( 'NONE',  ( 54.09612160359786515, 51.69948385550240744, -5.676469297603166098 ) ) ;
#11962=CARTESIAN_POINT ( 'NONE',  ( 45.31609314410960820, 54.30051614449765651, -6.485486291978072693 ) ) ;
#11973=CARTESIAN_POINT ( 'NONE',  ( 55.94051828345050836, 61.79948385550240175, -4.345558710429103577 ) ) ;
#11977=CARTESIAN_POINT ( 'NONE',  ( 56.65037692655918988, 55.89948385550240317, -2.184720259617163762 ) ) ;
#11979=CARTESIAN_POINT ( 'NONE',  ( 57.60143344285433642, 51.89948385550241028, -2.493737253992118319 ) ) ;
#11981=CARTESIAN_POINT ( 'NONE',  ( 47.74827507625469281, 56.40051614449766504, -7.007379884777203749 ) ) ;
#11991=CARTESIAN_POINT ( 'NONE',  ( 42.63976443033212860, 64.99948385550240459, 0.02388180880522514787 ) ) ;
#11997=CARTESIAN_POINT ( 'NONE',  ( 55.71335778527780747, 56.09948385550240602, 1.832500667257165983 ) ) ;
#12000=CARTESIAN_POINT ( 'NONE',  ( 56.81924384183006538, 50.80051614449766362, -4.924951120819380357 ) ) ;
#12001=CARTESIAN_POINT ( 'NONE',  ( 46.49166364869456913, 56.30051614449766362, -4.867452303228181343 ) ) ;
#12018=CARTESIAN_POINT ( 'NONE',  ( 42.39856655714564226, 64.10051614449766078, -2.493737253992044156 ) ) ;
#12022=ADVANCED_FACE ( 'NONE', ( #4461 ), #137, .T. ) ;
#12023=CARTESIAN_POINT ( 'NONE',  ( 50.02271294988512551, 58.49948385550241170, 7.000000000000000888 ) ) ;
#12026=CARTESIAN_POINT ( 'NONE',  ( 56.65037692655921120, 55.10051614449766078, 2.184720259617097593 ) ) ;
#12039=CARTESIAN_POINT ( 'NONE',  ( 44.03140696652192787, 47.19948385550240744, -4.306917132069425058 ) ) ;
#12045=CARTESIAN_POINT ( 'NONE',  ( 49.97728705011495265, 57.50051614449766646, 7.000000000000000888 ) ) ;
#12052=CARTESIAN_POINT ( 'NONE',  ( 44.91013252490150620, 52.20051614449766220, -3.727524721679154940 ) ) ;
#12055=CARTESIAN_POINT ( 'NONE',  ( 55.69932041026404335, 55.89948385550241028, -1.875703265242203432 ) ) ;
#12057=CARTESIAN_POINT ( 'NONE',  ( 42.39856655714564226, 54.10051614449766078, -2.493737253992044156 ) ) ;
#12068=CARTESIAN_POINT ( 'NONE',  ( 43.34962307344081012, 64.89948385550239607, 2.184720259617164650 ) ) ;
#12073=CARTESIAN_POINT ( 'NONE',  ( 47.70284917648453415, 61.39948385550241738, -6.992620115222774047 ) ) ;
#12075=CARTESIAN_POINT ( 'NONE',  ( 49.97728705011486738, 51.49948385550240459, -8.000000000000001776 ) ) ;
#12077=CARTESIAN_POINT ( 'NONE',  ( 54.13287192849671214, 54.70051614449766220, -5.649768623646139964 ) ) ;
#12088=CARTESIAN_POINT ( 'NONE',  ( 54.09612160359786515, 61.69948385550240744, -5.676469297603166098 ) ) ;
#12093=CARTESIAN_POINT ( 'NONE',  ( 55.11794222512601493, 54.19948385550241454, 3.688883143319541702 ) ) ;
#12096=CARTESIAN_POINT ( 'NONE',  ( 54.72065718078918906, 54.70051614449765509, -6.458785618021089192 ) ) ;
#12097=CARTESIAN_POINT ( 'NONE',  ( 46.45491332379576477, 55.70051614449766220, 4.840751629271188961 ) ) ;
#12103=ORIENTED_EDGE ( 'NONE', *, *, #11067, .F. ) ;
#12104=CARTESIAN_POINT ( 'NONE',  ( 44.03140696652192787, 63.19948385550240744, -4.306917132069425058 ) ) ;
#12108=CARTESIAN_POINT ( 'NONE',  ( 56.66441430157296821, 46.09948385550240602, 2.141517661632100111 ) ) ;
#12113=CARTESIAN_POINT ( 'NONE',  ( 42.39856655714566358, 48.89948385550241028, 2.493737253992119207 ) ) ;
#12116=CARTESIAN_POINT ( 'NONE',  ( 44.03140696652192787, 57.19948385550238612, -4.306917132069425058 ) ) ;
#12119=CARTESIAN_POINT ( 'NONE',  ( 56.65037692655921120, 57.10051614449766078, 2.184720259617097593 ) ) ;
#12131=CARTESIAN_POINT ( 'NONE',  ( 55.96859303347804371, 46.19948385550238612, 4.306917132069425946 ) ) ;
#12138=CARTESIAN_POINT ( 'NONE',  ( 56.66441430157294690, 60.90051614449766504, -2.141517661632166281 ) ) ;
#12143=CARTESIAN_POINT ( 'NONE',  ( 55.69932041026405045, 57.10051614449766788, 1.875703265242156359 ) ) ;
#12149=CARTESIAN_POINT ( 'NONE',  ( 55.71335778527780747, 56.09948385550240602, 1.832500667257165983 ) ) ;
#12151=CARTESIAN_POINT ( 'NONE',  ( 52.62207051974829852, 54.60051614449766788, -7.992620115222797139 ) ) ;
#12154=COLOUR_RGB ( '',0.8941176470588234615, 0.8941176470588234615, 0.8941176470588234615 ) ;
#12158=SHAPE_DEFINITION_REPRESENTATION ( #2748, #1926 ) ;
#12164=CARTESIAN_POINT ( 'NONE',  ( 55.94051828345050836, 63.79948385550240886, -4.345558710429103577 ) ) ;
#12170=CARTESIAN_POINT ( 'NONE',  ( 52.29715082351547295, 56.39948385550238896, 6.992620115222774047 ) ) ;
#12172=CARTESIAN_POINT ( 'NONE',  ( 50.02271294988513972, 54.49948385550240459, 8.000000000000001776 ) ) ;
#12175=CARTESIAN_POINT ( 'NONE',  ( 56.66441430157294690, 54.90051614449765793, -2.141517661632166281 ) ) ;
#12180=CARTESIAN_POINT ( 'NONE',  ( 54.09612160359792199, 49.30051614449765651, 5.676469297603124353 ) ) ;
#12190=CARTESIAN_POINT ( 'NONE',  ( 46.49166364869460466, 54.69948385550240033, 4.867452303228209765 ) ) ;
#12194=CARTESIAN_POINT ( 'NONE',  ( 45.27934281921082516, 55.70051614449766220, 6.458785618021089192 ) ) ;
#12195=CARTESIAN_POINT ( 'NONE',  ( 44.88205777487401349, 55.80051614449766362, 3.688883143319584779 ) ) ;
#12199=ORIENTED_EDGE ( 'NONE', *, *, #18385, .F. ) ;
#12207=CARTESIAN_POINT ( 'NONE',  ( 47.74827507625477807, 52.59948385550239891, 7.007379884777229506 ) ) ;
#12212=CARTESIAN_POINT ( 'NONE',  ( 52.62207051974839089, 48.39948385550240317, 7.992620115222770494 ) ) ;
#12216=CARTESIAN_POINT ( 'NONE',  ( 43.34962307344081012, 56.89948385550240317, 2.184720259617164650 ) ) ;
#12221=CARTESIAN_POINT ( 'NONE',  ( 50.02271294988505446, 54.50051614449765935, -7.000000000000000888 ) ) ;
#12231=CARTESIAN_POINT ( 'NONE',  ( 56.66441430157296821, 52.09948385550240602, 2.141517661632100111 ) ) ;
#12239=CARTESIAN_POINT ( 'NONE',  ( 50.02271294988505446, 60.50051614449765935, -7.000000000000000888 ) ) ;
#12244=CARTESIAN_POINT ( 'NONE',  ( 44.91013252490150620, 58.20051614449766220, -3.727524721679154940 ) ) ;
#12247=CARTESIAN_POINT ( 'NONE',  ( 55.69932041026404335, 63.89948385550240317, -1.875703265242203432 ) ) ;
#12251=CARTESIAN_POINT ( 'NONE',  ( 42.39856655714564226, 56.10051614449766078, -2.493737253992044156 ) ) ;
#12264=CARTESIAN_POINT ( 'NONE',  ( 57.36023556966787851, 61.99948385550240459, -0.02388180880522424582 ) ) ;
#12268=EDGE_CURVE ( 'NONE', #9631, #14352, #6419, .T. ) ;
#12271=CARTESIAN_POINT ( 'NONE',  ( 56.66441430157296821, 58.09948385550240602, 2.141517661632100111 ) ) ;
#12273=CARTESIAN_POINT ( 'NONE',  ( 43.18075615816989199, 61.19948385550241454, -4.924951120819313743 ) ) ;
#12274=CARTESIAN_POINT ( 'NONE',  ( 44.03140696652198471, 55.80051614449766362, 4.306917132069485454 ) ) ;
#12282=CARTESIAN_POINT ( 'NONE',  ( 44.05948171654945611, 46.20051614449766220, -4.345558710429044069 ) ) ;
#12289=CARTESIAN_POINT ( 'NONE',  ( 55.08986747509849380, 45.20051614449766220, 3.727524721679155384 ) ) ;
#12293=CARTESIAN_POINT ( 'NONE',  ( 54.68390685589039890, 59.30051614449766362, 6.485486291978072693 ) ) ;
#12294=CARTESIAN_POINT ( 'NONE',  ( 56.30877334542961421, 57.00051614449766646, 0.02388180880515774693 ) ) ;
#12295=DIRECTION ( 'NONE',  ( -1.224646799147353207E-16, 0.000000000000000000, -1.000000000000000000 ) ) ;
#12302=CARTESIAN_POINT ( 'NONE',  ( 43.34962307344078880, 56.10051614449766078, -2.184720259617096705 ) ) ;
#12305=CARTESIAN_POINT ( 'NONE',  ( 54.13287192849676188, 54.29948385550240886, 5.649768623646098220 ) ) ;
#12309=CARTESIAN_POINT ( 'NONE',  ( 52.57664461997811856, 47.59948385550239891, -8.007379884777229506 ) ) ;
#12310=CARTESIAN_POINT ( 'NONE',  ( 52.95539523038642926, 45.00000000000002132, -5.827023132204991462 ) ) ;
#12311=CARTESIAN_POINT ( 'NONE',  ( 52.25172492374522903, 61.59948385550239891, -7.007379884777225953 ) ) ;
#12314=CARTESIAN_POINT ( 'NONE',  ( 52.29715082351538769, 52.60051614449766788, -6.992620115222796251 ) ) ;
#12316=CARTESIAN_POINT ( 'NONE',  ( 56.66441430157296821, 54.09948385550240602, 2.141517661632100111 ) ) ;
#12325=CARTESIAN_POINT ( 'NONE',  ( 50.02271294988512551, 52.49948385550240459, 7.000000000000000888 ) ) ;
#12331=CARTESIAN_POINT ( 'NONE',  ( 42.63976443033212149, 60.00051614449765225, -0.02388180880514948964 ) ) ;
#12335=CARTESIAN_POINT ( 'NONE',  ( 50.02271294988506156, 54.50051614449765935, -6.000000000000000888 ) ) ;
#12341=CARTESIAN_POINT ( 'NONE',  ( 58.41169779390614281, 61.00051614449765935, 0.02388180880515032231 ) ) ;
#12352=CARTESIAN_POINT ( 'NONE',  ( 49.97728705011488159, 65.49948385550240459, -7.000000000000000888 ) ) ;
#12357=CARTESIAN_POINT ( 'NONE',  ( 49.97728705011488159, 65.49948385550240459, -7.000000000000000888 ) ) ;
#12359=CARTESIAN_POINT ( 'NONE',  ( 47.42335538002188144, 62.59948385550238470, 8.007379884777233059 ) ) ;
#12361=CARTESIAN_POINT ( 'NONE',  ( 45.90387839640208512, 58.30051614449766362, -5.676469297603124353 ) ) ;
#12369=CARTESIAN_POINT ( 'NONE',  ( 45.90387839640208512, 46.30051614449766362, -5.676469297603124353 ) ) ;
#12377=CARTESIAN_POINT ( 'NONE',  ( 56.30877334542961421, 63.99948385550241170, -0.02388180880520959434 ) ) ;
#12379=CARTESIAN_POINT ( 'NONE',  ( 55.96859303347804371, 46.19948385550238612, 4.306917132069425946 ) ) ;
#12380=CARTESIAN_POINT ( 'NONE',  ( 57.61547081786810764, 56.90051614449767214, -2.450534656007114176 ) ) ;
#12383=CARTESIAN_POINT ( 'NONE',  ( 43.69122665457040000, 58.00051614449765935, -0.02388180880515696977 ) ) ;
#12397=CARTESIAN_POINT ( 'NONE',  ( 44.05948171654949874, 50.79948385550239465, 4.345558710429104465 ) ) ;
#12403=CARTESIAN_POINT ( 'NONE',  ( 58.41169779390614281, 55.99948385550241170, -0.02388180880523160798 ) ) ;
#12405=CARTESIAN_POINT ( 'NONE',  ( 51.97223112728254790, 46.39948385550240317, 5.992620115222778487 ) ) ;
#12408=CARTESIAN_POINT ( 'NONE',  ( 52.29715082351538769, 58.60051614449766078, -6.992620115222796251 ) ) ;
#12410=CARTESIAN_POINT ( 'NONE',  ( 54.13287192849676188, 60.29948385550240886, 5.649768623646098220 ) ) ;
#12417=CARTESIAN_POINT ( 'NONE',  ( 43.34962307344081012, 48.89948385550240317, 2.184720259617164650 ) ) ;
#12429=CARTESIAN_POINT ( 'NONE',  ( 44.28664221472221385, 63.90051614449765793, 1.832500667257213722 ) ) ;
#12434=CARTESIAN_POINT ( 'NONE',  ( 45.31609314410960820, 60.30051614449767072, -6.485486291978072693 ) ) ;
#12452=CARTESIAN_POINT ( 'NONE',  ( 43.33558569842703179, 63.09948385550240602, -2.141517661632099223 ) ) ;
#12454=CARTESIAN_POINT ( 'NONE',  ( 45.27934281921075410, 61.29948385550240886, -6.458785618021043895 ) ) ;
#12455=CARTESIAN_POINT ( 'NONE',  ( 43.34962307344078880, 58.10051614449766078, -2.184720259617096705 ) ) ;
#12471=CARTESIAN_POINT ( 'NONE',  ( 51.97223112728254790, 60.39948385550241028, 5.992620115222778487 ) ) ;
#12472=DIRECTION ( 'NONE',  ( 0.9989677110047502362, 0.04542589977017699732, -6.931730960091013400E-15 ) ) ;
#12474=CARTESIAN_POINT ( 'NONE',  ( 43.18075615816994173, 59.80051614449766362, 4.924951120819380357 ) ) ;
#12475=CARTESIAN_POINT ( 'NONE',  ( 46.45491332379576477, 59.70051614449766220, 4.840751629271188961 ) ) ;
#12489=CARTESIAN_POINT ( 'NONE',  ( 56.66441430157296821, 52.09948385550240602, 2.141517661632100111 ) ) ;
#12494=CARTESIAN_POINT ( 'NONE',  ( 45.27934281921075410, 51.29948385550240175, -6.458785618021043895 ) ) ;
#12497=CARTESIAN_POINT ( 'NONE',  ( 44.28664221472220675, 47.09948385550240602, -1.832500667257165317 ) ) ;
#12500=CARTESIAN_POINT ( 'NONE',  ( 42.63976443033212860, 62.00051614449764514, -0.02388180880514948964 ) ) ;
#12507=CARTESIAN_POINT ( 'NONE',  ( 47.74827507625478518, 56.59948385550238470, 7.007379884777227730 ) ) ;
#12516=CARTESIAN_POINT ( 'NONE',  ( 47.74827507625478518, 52.59948385550239180, 7.007379884777227730 ) ) ;
#12525=CARTESIAN_POINT ( 'NONE',  ( 55.96859303347802239, 62.80051614449766362, -4.306917132069484566 ) ) ;
#12528=CARTESIAN_POINT ( 'NONE',  ( 56.65037692655918988, 45.89948385550240317, -2.184720259617163762 ) ) ;
#12530=AXIS2_PLACEMENT_3D ( 'NONE', #18708, #14555, #12705 ) ;
#12531=CARTESIAN_POINT ( 'NONE',  ( 44.28664221472221385, 59.90051614449767214, 1.832500667257213722 ) ) ;
#12536=CARTESIAN_POINT ( 'NONE',  ( 56.81924384183006538, 58.80051614449766362, -4.924951120819380357 ) ) ;
#12558=CARTESIAN_POINT ( 'NONE',  ( 56.30877334542961421, 45.99948385550240459, -0.02388180880520959434 ) ) ;
#12560=CARTESIAN_POINT ( 'NONE',  ( 43.18075615816989199, 57.19948385550241454, -4.924951120819313743 ) ) ;
#12561=CARTESIAN_POINT ( 'NONE',  ( 42.63976443033212860, 60.00051614449764514, -0.02388180880514948964 ) ) ;
#12570=CARTESIAN_POINT ( 'NONE',  ( 44.05948171654945611, 48.20051614449764799, -4.345558710429044069 ) ) ;
#12576=CARTESIAN_POINT ( 'NONE',  ( 50.02271294988511841, 64.49948385550239038, 6.000000000000000888 ) ) ;
#12578=CARTESIAN_POINT ( 'NONE',  ( 47.74827507625478518, 46.59948385550239891, 7.007379884777227730 ) ) ;
#12580=CARTESIAN_POINT ( 'NONE',  ( 45.27934281921082516, 61.70051614449766220, 6.458785618021089192 ) ) ;
#12581=CARTESIAN_POINT ( 'NONE',  ( 55.11794222512599362, 60.80051614449766362, -3.688883143319583446 ) ) ;
#12592=CARTESIAN_POINT ( 'NONE',  ( 52.29715082351547295, 54.39948385550239607, 6.992620115222774047 ) ) ;
#12596=CARTESIAN_POINT ( 'NONE',  ( 42.39856655714566358, 52.89948385550241028, 2.493737253992119207 ) ) ;
#12598=CARTESIAN_POINT ( 'NONE',  ( 44.05948171654949874, 62.79948385550241596, 4.345558710429105354 ) ) ;
#12601=CARTESIAN_POINT ( 'NONE',  ( 50.02271294988505446, 60.50051614449765935, -7.000000000000000888 ) ) ;
#12602=CARTESIAN_POINT ( 'NONE',  ( 55.08986747509849380, 45.20051614449766220, 3.727524721679155384 ) ) ;
#12603=CARTESIAN_POINT ( 'NONE',  ( 42.63976443033212860, 56.99948385550241170, 0.02388180880522514787 ) ) ;
#12613=CARTESIAN_POINT ( 'NONE',  ( 49.97728705011488159, 53.49948385550240459, -7.000000000000000888 ) ) ;
#12627=CARTESIAN_POINT ( 'NONE',  ( 55.11794222512599362, 60.80051614449766362, -3.688883143319583446 ) ) ;
#12632=CARTESIAN_POINT ( 'NONE',  ( 41.58830220609386430, 58.00051614449765935, -0.02388180880514929535 ) ) ;
#12637=( NAMED_UNIT ( * ) SI_UNIT ( $, .STERADIAN. ) SOLID_ANGLE_UNIT ( ) );
#12653=CARTESIAN_POINT ( 'NONE',  ( 56.65037692655918988, 61.89948385550241028, -2.184720259617163762 ) ) ;
#12655=CARTESIAN_POINT ( 'NONE',  ( 42.39856655714566358, 58.89948385550241028, 2.493737253992119207 ) ) ;
#12656=CARTESIAN_POINT ( 'NONE',  ( 44.05948171654945611, 58.20051614449764799, -4.345558710429044069 ) ) ;
#12665=CARTESIAN_POINT ( 'NONE',  ( 52.29715082351539479, 52.60051614449766078, -6.992620115222796251 ) ) ;
#12676=CARTESIAN_POINT ( 'NONE',  ( 56.79116909180259398, 57.20051614449766220, 4.963592699178938972 ) ) ;
#12678=CARTESIAN_POINT ( 'NONE',  ( 43.69122665457040000, 60.00051614449765935, -0.02388180880515696977 ) ) ;
#12690=CARTESIAN_POINT ( 'NONE',  ( 42.63976443033212149, 58.99948385550239038, 0.02388180880522514787 ) ) ;
#12694=CARTESIAN_POINT ( 'NONE',  ( 42.39856655714566358, 54.89948385550240317, 2.493737253992119207 ) ) ;
#12697=CARTESIAN_POINT ( 'NONE',  ( 47.70284917648453415, 65.39948385550239607, -6.992620115222774047 ) ) ;
#12700=CARTESIAN_POINT ( 'NONE',  ( 44.03140696652198471, 59.80051614449766362, 4.306917132069485454 ) ) ;
#12701=CARTESIAN_POINT ( 'NONE',  ( 56.30877334542961421, 61.99948385550241170, -0.02388180880520959434 ) ) ;
#12703=CARTESIAN_POINT ( 'NONE',  ( 50.02271294988512551, 58.49948385550241170, 7.000000000000000888 ) ) ;
#12705=DIRECTION ( 'NONE',  ( -0.04542589977017699732, 0.9989677110047501252, 0.000000000000000000 ) ) ;
#12707=VERTEX_POINT ( 'NONE', #9602 ) ;
#12711=CARTESIAN_POINT ( 'NONE',  ( 45.86712807150323812, 55.29948385550240175, -5.649768623646098220 ) ) ;
#12718=CARTESIAN_POINT ( 'NONE',  ( 47.70284917648459810, 63.60051614449766078, 6.992620115222797139 ) ) ;
#12721=CARTESIAN_POINT ( 'NONE',  ( 56.66441430157296821, 46.09948385550240602, 2.141517661632100111 ) ) ;
#12724=CARTESIAN_POINT ( 'NONE',  ( 50.02271294988506156, 60.50051614449766646, -6.000000000000000888 ) ) ;
#12732=PRESENTATION_STYLE_ASSIGNMENT (( #3530 ) ) ;
#12738=CARTESIAN_POINT ( 'NONE',  ( 62.49999999999998579, 45.00000000000001421, -5.000000000000000000 ) ) ;
#12750=CARTESIAN_POINT ( 'NONE',  ( 44.91013252490152752, 46.79948385550240886, 3.727524721679198461 ) ) ;
#12752=CARTESIAN_POINT ( 'NONE',  ( 57.61547081786812896, 64.09948385550239891, 2.450534656007040901 ) ) ;
#12753=CARTESIAN_POINT ( 'NONE',  ( 56.66441430157294690, 58.90051614449766504, -2.141517661632166281 ) ) ;
#12763=CARTESIAN_POINT ( 'NONE',  ( 50.02271294988505446, 50.50051614449765935, -7.000000000000000888 ) ) ;
#12772=CARTESIAN_POINT ( 'NONE',  ( 56.66441430157296821, 48.09948385550240602, 2.141517661632100111 ) ) ;
#12775=CARTESIAN_POINT ( 'NONE',  ( 58.41169779390614281, 47.99948385550239038, -0.02388180880523160798 ) ) ;
#12776=CARTESIAN_POINT ( 'NONE',  ( 44.30067958973594955, 64.10051614449766078, -1.875703265242155693 ) ) ;
#12778=FACE_OUTER_BOUND ( 'NONE', #13514, .T. ) ;
#12791=CARTESIAN_POINT ( 'NONE',  ( 54.09612160359786515, 55.69948385550240744, -5.676469297603166098 ) ) ;
#12797=CARTESIAN_POINT ( 'NONE',  ( 54.72065718078924590, 50.29948385550240886, 6.458785618021043895 ) ) ;
#12799=CARTESIAN_POINT ( 'NONE',  ( 50.02271294988511841, 48.49948385550241170, 6.000000000000000888 ) ) ;
#12803=CARTESIAN_POINT ( 'NONE',  ( 55.96859303347802239, 62.80051614449766362, -4.306917132069484566 ) ) ;
#12804=CARTESIAN_POINT ( 'NONE',  ( 46.49166364869460466, 62.69948385550240744, 4.867452303228209765 ) ) ;
#12812=CARTESIAN_POINT ( 'NONE',  ( 52.25172492374522903, 61.59948385550239891, -7.007379884777225953 ) ) ;
#12824=CARTESIAN_POINT ( 'NONE',  ( 47.70284917648453415, 51.39948385550238896, -6.992620115222774047 ) ) ;
#12826=CARTESIAN_POINT ( 'NONE',  ( 48.07319477248762496, 60.40051614449765793, -6.007379884777208190 ) ) ;
#12844=CARTESIAN_POINT ( 'NONE',  ( 53.50833635130540955, 49.69948385550240744, -4.867452303228209765 ) ) ;
#12848=CARTESIAN_POINT ( 'NONE',  ( 55.96859303347804371, 48.19948385550240033, 4.306917132069425946 ) ) ;
#12849=CARTESIAN_POINT ( 'NONE',  ( 45.31609314410960820, 50.30051614449766362, -6.485486291978072693 ) ) ;
#12862=CARTESIAN_POINT ( 'NONE',  ( 49.97728705011495265, 55.50051614449766646, 7.000000000000000888 ) ) ;
#12872=CARTESIAN_POINT ( 'NONE',  ( 56.66441430157296821, 54.09948385550240602, 2.141517661632100111 ) ) ;
#12874=CARTESIAN_POINT ( 'NONE',  ( 47.42335538002188144, 48.59948385550239891, 8.007379884777233059 ) ) ;
#12876=CARTESIAN_POINT ( 'NONE',  ( 54.13287192849671214, 44.70051614449766220, -5.649768623646139964 ) ) ;
#12890=CARTESIAN_POINT ( 'NONE',  ( 43.33558569842703179, 57.09948385550240602, -2.141517661632099223 ) ) ;
#12895=CARTESIAN_POINT ( 'NONE',  ( 52.62207051974839089, 62.39948385550240317, 7.992620115222770494 ) ) ;
#12897=CARTESIAN_POINT ( 'NONE',  ( 46.49166364869460466, 52.69948385550240744, 4.867452303228209765 ) ) ;
#12901=CARTESIAN_POINT ( 'NONE',  ( 47.42335538002180328, 46.40051614449765793, -8.007379884777206414 ) ) ;
#12902=CARTESIAN_POINT ( 'NONE',  ( 43.69122665457040000, 60.99948385550241170, 0.02388180880521036456 ) ) ;
#12909=CARTESIAN_POINT ( 'NONE',  ( 43.34962307344081012, 56.89948385550240317, 2.184720259617164650 ) ) ;
#12917=CARTESIAN_POINT ( 'NONE',  ( 45.90387839640214196, 52.69948385550240033, 5.676469297603166098 ) ) ;
#12920=CARTESIAN_POINT ( 'NONE',  ( 56.66441430157294690, 44.90051614449765793, -2.141517661632166281 ) ) ;
#12938=CARTESIAN_POINT ( 'NONE',  ( 55.11794222512599362, 50.80051614449766362, -3.688883143319583446 ) ) ;
#12941=CARTESIAN_POINT ( 'NONE',  ( 51.92680522751233951, 51.59948385550240602, -6.007379884777223289 ) ) ;
#12943=CARTESIAN_POINT ( 'NONE',  ( 49.97728705011486738, 63.49948385550241170, -8.000000000000001776 ) ) ;
#12944=CARTESIAN_POINT ( 'NONE',  ( 54.72065718078918906, 48.70051614449766930, -6.458785618021089192 ) ) ;
#12952=CARTESIAN_POINT ( 'NONE',  ( 43.33558569842706021, 49.90051614449766504, 2.141517661632167169 ) ) ;
#12960=CARTESIAN_POINT ( 'NONE',  ( 52.29715082351547295, 50.39948385550240317, 6.992620115222774047 ) ) ;
#12962=CARTESIAN_POINT ( 'NONE',  ( 43.18075615816994173, 63.80051614449766362, 4.924951120819380357 ) ) ;
#12964=CARTESIAN_POINT ( 'NONE',  ( 52.29715082351538769, 46.60051614449766078, -6.992620115222796251 ) ) ;
#12977=CARTESIAN_POINT ( 'NONE',  ( 54.09612160359786515, 59.69948385550240033, -5.676469297603166098 ) ) ;
#12981=CARTESIAN_POINT ( 'NONE',  ( 52.62207051974839089, 60.39948385550241028, 7.992620115222770494 ) ) ;
#12985=CARTESIAN_POINT ( 'NONE',  ( 44.30067958973596376, 48.89948385550241028, 1.875703265242204099 ) ) ;
#12989=CARTESIAN_POINT ( 'NONE',  ( 43.18075615816994173, 49.80051614449765651, 4.924951120819380357 ) ) ;
#12991=CARTESIAN_POINT ( 'NONE',  ( 55.69932041026405045, 49.10051614449766788, 1.875703265242156359 ) ) ;
#13004=CARTESIAN_POINT ( 'NONE',  ( 55.94051828345050836, 57.79948385550238754, -4.345558710429104465 ) ) ;
#13013=CARTESIAN_POINT ( 'NONE',  ( 47.70284917648453415, 49.39948385550238896, -6.992620115222774047 ) ) ;
#13016=CARTESIAN_POINT ( 'NONE',  ( 55.96859303347802239, 48.80051614449766362, -4.306917132069484566 ) ) ;
#13037=CARTESIAN_POINT ( 'NONE',  ( 55.69932041026405045, 49.10051614449766788, 1.875703265242156359 ) ) ;
#13040=CARTESIAN_POINT ( 'NONE',  ( 53.50833635130540955, 53.69948385550240744, -4.867452303228209765 ) ) ;
#13042=CARTESIAN_POINT ( 'NONE',  ( 55.94051828345050836, 47.79948385550240886, -4.345558710429104465 ) ) ;
#13043=CARTESIAN_POINT ( 'NONE',  ( 50.02271294988505446, 44.50051614449765935, -8.000000000000001776 ) ) ;
#13054=CARTESIAN_POINT ( 'NONE',  ( 45.90387839640208512, 50.30051614449766362, -5.676469297603124353 ) ) ;
#13062=CARTESIAN_POINT ( 'NONE',  ( 44.05948171654949874, 52.79948385550240175, 4.345558710429105354 ) ) ;
#13064=CARTESIAN_POINT ( 'NONE',  ( 54.68390685589039890, 63.30051614449767072, 6.485486291978072693 ) ) ;
#13066=CARTESIAN_POINT ( 'NONE',  ( 50.02271294988505446, 48.50051614449765935, -7.000000000000000888 ) ) ;
#13082=CARTESIAN_POINT ( 'NONE',  ( 43.18075615816989199, 59.19948385550240744, -4.924951120819313743 ) ) ;
#13085=CARTESIAN_POINT ( 'NONE',  ( 51.97223112728254790, 50.39948385550241738, 5.992620115222778487 ) ) ;
#13088=CARTESIAN_POINT ( 'NONE',  ( 41.58830220609386430, 48.00051614449766646, -0.02388180880514929535 ) ) ;
#13089=CARTESIAN_POINT ( 'NONE',  ( 55.08986747509849380, 51.20051614449766220, 3.727524721679155384 ) ) ;
#13100=CARTESIAN_POINT ( 'NONE',  ( 56.65037692655918988, 55.89948385550240317, -2.184720259617163762 ) ) ;
#13112=CARTESIAN_POINT ( 'NONE',  ( 42.63976443033212860, 50.99948385550240459, 0.02388180880522514787 ) ) ;
#13114=CARTESIAN_POINT ( 'NONE',  ( 56.65037692655921120, 51.10051614449766078, 2.184720259617097593 ) ) ;
#13136=CARTESIAN_POINT ( 'NONE',  ( 53.50833635130544508, 49.30051614449766362, 4.867452303228181343 ) ) ;
#13139=CARTESIAN_POINT ( 'NONE',  ( 53.54508667620428497, 52.29948385550240886, 4.840751629271157874 ) ) ;
#13141=CARTESIAN_POINT ( 'NONE',  ( 43.33558569842703179, 49.09948385550240602, -2.141517661632099223 ) ) ;
#13143=CARTESIAN_POINT ( 'NONE',  ( 45.31609314410960820, 48.30051614449765651, -6.485486291978072693 ) ) ;
#13159=CARTESIAN_POINT ( 'NONE',  ( 44.03140696652192787, 53.19948385550238612, -4.306917132069425058 ) ) ;
#13162=CARTESIAN_POINT ( 'NONE',  ( 43.20883090819745576, 48.79948385550240175, 4.963592699179006473 ) ) ;
#13164=CARTESIAN_POINT ( 'NONE',  ( 43.33558569842706021, 47.90051614449765793, 2.141517661632167169 ) ) ;
#13181=CARTESIAN_POINT ( 'NONE',  ( 57.61547081786812896, 60.09948385550240602, 2.450534656007040901 ) ) ;
#13184=CARTESIAN_POINT ( 'NONE',  ( 44.91013252490152752, 52.79948385550240175, 3.727524721679198461 ) ) ;
#13189=CARTESIAN_POINT ( 'NONE',  ( 45.27934281921082516, 49.70051614449766220, 6.458785618021089192 ) ) ;
#13190=CARTESIAN_POINT ( 'NONE',  ( 53.50833635130544508, 51.30051614449765651, 4.867452303228181343 ) ) ;
#13197=CARTESIAN_POINT ( 'NONE',  ( 47.70284917648453415, 63.39948385550240317, -6.992620115222774047 ) ) ;
#13202=CARTESIAN_POINT ( 'NONE',  ( 52.25172492374522903, 45.59948385550240602, -7.007379884777227730 ) ) ;
#13208=CARTESIAN_POINT ( 'NONE',  ( 54.13287192849676188, 54.29948385550240886, 5.649768623646098220 ) ) ;
#13210=CARTESIAN_POINT ( 'NONE',  ( 52.29715082351538769, 48.60051614449766788, -6.992620115222796251 ) ) ;
#13230=CARTESIAN_POINT ( 'NONE',  ( 55.11794222512599362, 46.80051614449766362, -3.688883143319583446 ) ) ;
#13235=CARTESIAN_POINT ( 'NONE',  ( 50.02271294988511841, 52.49948385550241170, 6.000000000000000888 ) ) ;
#13237=CARTESIAN_POINT ( 'NONE',  ( 49.97728705011488159, 49.49948385550240459, -7.000000000000000888 ) ) ;
#13238=CARTESIAN_POINT ( 'NONE',  ( 57.60143344285435774, 49.10051614449766788, 2.493737253992045044 ) ) ;
#13254=CARTESIAN_POINT ( 'NONE',  ( 54.13287192849676188, 52.29948385550240886, 5.649768623646098220 ) ) ;
#13256=CARTESIAN_POINT ( 'NONE',  ( 41.58830220609386430, 52.99948385550241170, 0.02388180880523263147 ) ) ;
#13259=CARTESIAN_POINT ( 'NONE',  ( 44.05948171654945611, 48.20051614449764799, -4.345558710429044069 ) ) ;
#13274=CARTESIAN_POINT ( 'NONE',  ( 56.79116909180255135, 59.79948385550240175, -4.963592699179005585 ) ) ;
#13277=CARTESIAN_POINT ( 'NONE',  ( 48.07319477248768180, 54.59948385550240602, 6.007379884777225953 ) ) ;
#13281=CARTESIAN_POINT ( 'NONE',  ( 45.31609314410960820, 52.30051614449766362, -6.485486291978072693 ) ) ;
#13283=CARTESIAN_POINT ( 'NONE',  ( 48.07319477248762496, 52.40051614449767214, -6.007379884777208190 ) ) ;
#13291=FACE_OUTER_BOUND ( 'NONE', #4880, .T. ) ;
#13295=CARTESIAN_POINT ( 'NONE',  ( 56.66441430157296821, 48.09948385550240602, 2.141517661632100111 ) ) ;
#13301=CARTESIAN_POINT ( 'NONE',  ( 56.65037692655918988, 57.89948385550240317, -2.184720259617163762 ) ) ;
#13303=CARTESIAN_POINT ( 'NONE',  ( 45.90387839640208512, 50.30051614449766362, -5.676469297603124353 ) ) ;
#13314=CARTESIAN_POINT ( 'NONE',  ( 57.36023556966787851, 45.99948385550238328, -0.02388180880522424582 ) ) ;
#13322=CARTESIAN_POINT ( 'NONE',  ( 51.97223112728249816, 48.60051614449766788, -5.992620115222793586 ) ) ;
#13325=CARTESIAN_POINT ( 'NONE',  ( 56.30877334542961421, 57.99948385550241170, -0.02388180880520959434 ) ) ;
#13327=CARTESIAN_POINT ( 'NONE',  ( 57.36023556966787851, 53.99948385550239038, -0.02388180880522424582 ) ) ;
#13328=CARTESIAN_POINT ( 'NONE',  ( 45.27934281921082516, 55.70051614449766220, 6.458785618021089192 ) ) ;
#13349=CARTESIAN_POINT ( 'NONE',  ( 55.94051828345050836, 57.79948385550238754, -4.345558710429104465 ) ) ;
#13352=CARTESIAN_POINT ( 'NONE',  ( 41.58830220609386430, 54.99948385550239749, 0.02388180880523263147 ) ) ;
#13354=CARTESIAN_POINT ( 'NONE',  ( 57.36023556966787851, 51.00051614449763804, 0.02388180880515038476 ) ) ;
#13373=CARTESIAN_POINT ( 'NONE',  ( 46.45491332379572924, 55.29948385550240175, -4.840751629271157874 ) ) ;
#13376=CARTESIAN_POINT ( 'NONE',  ( 56.79116909180259398, 51.20051614449766220, 4.963592699178938972 ) ) ;
#13377=CARTESIAN_POINT ( 'NONE',  ( 44.91013252490150620, 52.20051614449766220, -3.727524721679154940 ) ) ;
#13387=CARTESIAN_POINT ( 'NONE',  ( 45.90387839640214196, 64.69948385550240744, 5.676469297603166098 ) ) ;
#13393=CARTESIAN_POINT ( 'NONE',  ( 50.02271294988512551, 46.49948385550240459, 7.000000000000000888 ) ) ;
#13399=CARTESIAN_POINT ( 'NONE',  ( 56.79116909180255135, 45.79948385550240886, -4.963592699179005585 ) ) ;
#13401=CARTESIAN_POINT ( 'NONE',  ( 57.36023556966787851, 59.99948385550240459, -0.02388180880522424582 ) ) ;
#13403=CARTESIAN_POINT ( 'NONE',  ( 47.74827507625469281, 52.40051614449763662, -7.007379884777203749 ) ) ;
#13416=CARTESIAN_POINT ( 'NONE',  ( 54.72065718078924590, 64.29948385550240175, 6.458785618021043895 ) ) ;
#13421=CARTESIAN_POINT ( 'NONE',  ( 47.70284917648459810, 61.60051614449765367, 6.992620115222797139 ) ) ;
#13429=CARTESIAN_POINT ( 'NONE',  ( 51.92680522751238925, 55.40051614449767214, 6.007379884777208190 ) ) ;
#13432=CARTESIAN_POINT ( 'NONE',  ( 48.02776887271745210, 59.39948385550240317, -5.992620115222778487 ) ) ;
#13434=CARTESIAN_POINT ( 'NONE',  ( 43.33558569842703179, 51.09948385550240602, -2.141517661632099223 ) ) ;
#13435=CARTESIAN_POINT ( 'NONE',  ( 54.68390685589039890, 53.30051614449767072, 6.485486291978072693 ) ) ;
#13446=CARTESIAN_POINT ( 'NONE',  ( 45.90387839640214196, 62.69948385550240744, 5.676469297603166098 ) ) ;
#13451=CARTESIAN_POINT ( 'NONE',  ( 47.70284917648453415, 57.39948385550241028, -6.992620115222774047 ) ) ;
#13453=CARTESIAN_POINT ( 'NONE',  ( 57.61547081786812896, 56.09948385550240602, 2.450534656007040901 ) ) ;
#13456=CARTESIAN_POINT ( 'NONE',  ( 47.70284917648459100, 53.60051614449765367, 6.992620115222796251 ) ) ;
#13476=CARTESIAN_POINT ( 'NONE',  ( 43.69122665457040000, 58.99948385550239749, 0.02388180880521036456 ) ) ;
#13478=CARTESIAN_POINT ( 'NONE',  ( 43.20883090819742023, 54.20051614449766220, -4.963592699178938972 ) ) ;
#13481=CARTESIAN_POINT ( 'NONE',  ( 51.97223112728249816, 58.60051614449766788, -5.992620115222793586 ) ) ;
#13492=CARTESIAN_POINT ( 'NONE',  ( 50.02271294988512551, 64.49948385550240459, 7.000000000000000888 ) ) ;
#13502=CARTESIAN_POINT ( 'NONE',  ( 52.57664461997811856, 45.59948385550240602, -8.007379884777229506 ) ) ;
#13504=CARTESIAN_POINT ( 'NONE',  ( 54.23491683972284960, 45.00000000000001421, -4.999999999999999112 ) ) ;
#13505=CARTESIAN_POINT ( 'NONE',  ( 45.86712807150323812, 55.29948385550240175, -5.649768623646098220 ) ) ;
#13508=CARTESIAN_POINT ( 'NONE',  ( 43.33558569842706021, 51.90051614449765793, 2.141517661632167169 ) ) ;
#13514=EDGE_LOOP ( 'NONE', ( #14344, #17654, #16749, #15812 ) ) ;
#13518=CARTESIAN_POINT ( 'NONE',  ( 54.13287192849676188, 46.29948385550240886, 5.649768623646098220 ) ) ;
#13524=CARTESIAN_POINT ( 'NONE',  ( 43.33558569842706021, 61.90051614449766504, 2.141517661632167169 ) ) ;
#13529=CARTESIAN_POINT ( 'NONE',  ( 48.02776887271750184, 55.60051614449765367, 5.992620115222795363 ) ) ;
#13534=CARTESIAN_POINT ( 'NONE',  ( 43.69122665457040000, 56.99948385550241170, 0.02388180880521036456 ) ) ;
#13536=CARTESIAN_POINT ( 'NONE',  ( 42.38452918213190657, 53.90051614449765793, 2.450534656007115508 ) ) ;
#13546=CARTESIAN_POINT ( 'NONE',  ( 45.86712807150323812, 65.29948385550241596, -5.649768623646098220 ) ) ;
#13550=CARTESIAN_POINT ( 'NONE',  ( 44.05948171654949874, 60.79948385550240886, 4.345558710429105354 ) ) ;
#13552=CARTESIAN_POINT ( 'NONE',  ( 43.20883090819745576, 50.79948385550240175, 4.963592699179006473 ) ) ;
#13554=CARTESIAN_POINT ( 'NONE',  ( 45.86712807150329496, 51.70051614449766220, 5.649768623646139964 ) ) ;
#13569=CARTESIAN_POINT ( 'NONE',  ( 55.08986747509847248, 57.79948385550240175, -3.727524721679197572 ) ) ;
#13571=CARTESIAN_POINT ( 'NONE',  ( 52.62207051974829852, 52.60051614449765367, -7.992620115222797139 ) ) ;
#13572=CARTESIAN_POINT ( 'NONE',  ( 44.88205777487401349, 53.80051614449766362, 3.688883143319584779 ) ) ;
#13578=CARTESIAN_POINT ( 'NONE',  ( 54.23491683972284960, 45.00000000000001421, -4.999999999999999112 ) ) ;
#13580=CARTESIAN_POINT ( 'NONE',  ( 42.63976443033212860, 62.99948385550241170, 0.02388180880522514787 ) ) ;
#13590=CARTESIAN_POINT ( 'NONE',  ( 41.58830220609386430, 64.00051614449765225, -0.02388180880514929535 ) ) ;
#13593=CARTESIAN_POINT ( 'NONE',  ( 54.13287192849676188, 56.29948385550240175, 5.649768623646098220 ) ) ;
#13596=CARTESIAN_POINT ( 'NONE',  ( 54.09612160359792199, 51.30051614449766362, 5.676469297603124353 ) ) ;
#13606=CARTESIAN_POINT ( 'NONE',  ( 42.38452918213188525, 63.09948385550240602, -2.450534656007040013 ) ) ;
#13612=CARTESIAN_POINT ( 'NONE',  ( 44.03140696652198471, 59.80051614449766362, 4.306917132069485454 ) ) ;
#13619=CARTESIAN_POINT ( 'NONE',  ( 44.88205777487401349, 53.80051614449766362, 3.688883143319584779 ) ) ;
#13622=CARTESIAN_POINT ( 'NONE',  ( 51.92680522751233951, 59.59948385550240602, -6.007379884777223289 ) ) ;
#13625=CARTESIAN_POINT ( 'NONE',  ( 54.72065718078918906, 52.70051614449766220, -6.458785618021089192 ) ) ;
#13637=CARTESIAN_POINT ( 'NONE',  ( 43.33558569842703179, 61.09948385550240602, -2.141517661632099223 ) ) ;
#13642=CARTESIAN_POINT ( 'NONE',  ( 50.02271294988512551, 58.49948385550241170, 7.000000000000000888 ) ) ;
#13644=CARTESIAN_POINT ( 'NONE',  ( 43.18075615816989199, 55.19948385550240744, -4.924951120819313743 ) ) ;
#13646=CARTESIAN_POINT ( 'NONE',  ( 57.36023556966787851, 53.00051614449765225, 0.02388180880515038476 ) ) ;
#13655=CARTESIAN_POINT ( 'NONE',  ( 56.66441430157294690, 48.90051614449766504, -2.141517661632166281 ) ) ;
#13656=CARTESIAN_POINT ( 'NONE',  ( 50.02271294988512551, 64.49948385550240459, 7.000000000000000888 ) ) ;
#13661=CARTESIAN_POINT ( 'NONE',  ( 55.71335778527780747, 58.09948385550241312, 1.832500667257165983 ) ) ;
#13664=CARTESIAN_POINT ( 'NONE',  ( 41.58830220609386430, 54.00051614449765935, -0.02388180880514929535 ) ) ;
#13665=CARTESIAN_POINT ( 'NONE',  ( 44.91013252490150620, 56.20051614449766220, -3.727524721679154940 ) ) ;
#13676=CARTESIAN_POINT ( 'NONE',  ( 49.97728705011488159, 51.49948385550240459, -7.000000000000000888 ) ) ;
#13681=CARTESIAN_POINT ( 'NONE',  ( 54.68390685589033495, 45.69948385550240033, -6.485486291978119766 ) ) ;
#13684=CARTESIAN_POINT ( 'NONE',  ( 47.70284917648453415, 59.39948385550241028, -6.992620115222774047 ) ) ;
#13688=CARTESIAN_POINT ( 'NONE',  ( 55.94051828345053679, 55.20051614449766930, 4.345558710429044069 ) ) ;
#13700=CARTESIAN_POINT ( 'NONE',  ( 47.42335538002188144, 62.59948385550238470, 8.007379884777233059 ) ) ;
#13708=CARTESIAN_POINT ( 'NONE',  ( 55.94051828345054389, 57.20051614449766220, 4.345558710429044957 ) ) ;
#13713=CARTESIAN_POINT ( 'NONE',  ( 53.54508667620424234, 56.70051614449766930, -4.840751629271188961 ) ) ;
#13717=CARTESIAN_POINT ( 'NONE',  ( 46.45491332379572924, 65.29948385550241596, -4.840751629271157874 ) ) ;
#13720=CARTESIAN_POINT ( 'NONE',  ( 54.68390685589039890, 55.30051614449765651, 6.485486291978072693 ) ) ;
#13731=CARTESIAN_POINT ( 'NONE',  ( 56.65037692655918988, 61.89948385550241028, -2.184720259617163762 ) ) ;
#13735=CARTESIAN_POINT ( 'NONE',  ( 45.86712807150323812, 55.29948385550240175, -5.649768623646098220 ) ) ;
#13737=CARTESIAN_POINT ( 'NONE',  ( 49.97728705011486738, 59.49948385550240459, -8.000000000000001776 ) ) ;
#13739=CARTESIAN_POINT ( 'NONE',  ( 42.63976443033212860, 52.00051614449766646, -0.02388180880514948964 ) ) ;
#13747=CARTESIAN_POINT ( 'NONE',  ( 45.86712807150329496, 49.70051614449766220, 5.649768623646139964 ) ) ;
#13756=CARTESIAN_POINT ( 'NONE',  ( 44.28664221472220675, 65.09948385550239891, -1.832500667257165317 ) ) ;
#13759=CARTESIAN_POINT ( 'NONE',  ( 42.39856655714564226, 58.10051614449765367, -2.493737253992044156 ) ) ;
#13761=CARTESIAN_POINT ( 'NONE',  ( 55.71335778527780036, 56.90051614449767214, -1.832500667257213056 ) ) ;
#13773=CARTESIAN_POINT ( 'NONE',  ( 56.66441430157296821, 54.09948385550240602, 2.141517661632100111 ) ) ;
#13776=ORIENTED_EDGE ( 'NONE', *, *, #11053, .T. ) ;
#13777=CARTESIAN_POINT ( 'NONE',  ( 52.62207051974839089, 46.39948385550240317, 7.992620115222770494 ) ) ;
#13780=CARTESIAN_POINT ( 'NONE',  ( 55.96859303347804371, 62.19948385550240744, 4.306917132069425946 ) ) ;
#13785=CARTESIAN_POINT ( 'NONE',  ( 49.97728705011495265, 55.50051614449766646, 7.000000000000000888 ) ) ;
#13788=CARTESIAN_POINT ( 'NONE',  ( 44.05948171654949874, 52.79948385550240175, 4.345558710429105354 ) ) ;
#13795=CARTESIAN_POINT ( 'NONE',  ( 54.13287192849676188, 54.29948385550240886, 5.649768623646098220 ) ) ;
#13803=CARTESIAN_POINT ( 'NONE',  ( 56.65037692655921120, 59.10051614449766078, 2.184720259617097593 ) ) ;
#13809=CARTESIAN_POINT ( 'NONE',  ( 44.30067958973594955, 58.10051614449765367, -1.875703265242155693 ) ) ;
#13811=CARTESIAN_POINT ( 'NONE',  ( 44.88205777487401349, 45.80051614449766362, 3.688883143319584779 ) ) ;
#13815=CARTESIAN_POINT ( 'NONE',  ( 43.20883090819742023, 62.20051614449766220, -4.963592699178938972 ) ) ;
#13827=CARTESIAN_POINT ( 'NONE',  ( 42.63976443033212149, 62.99948385550241170, 0.02388180880522514787 ) ) ;
#13832=CARTESIAN_POINT ( 'NONE',  ( 55.69932041026404335, 47.89948385550240317, -1.875703265242203432 ) ) ;
#13834=CARTESIAN_POINT ( 'NONE',  ( 49.97728705011486738, 61.49948385550241170, -8.000000000000001776 ) ) ;
#13835=CARTESIAN_POINT ( 'NONE',  ( 42.63976443033212860, 54.00051614449766646, -0.02388180880514948964 ) ) ;
#13843=CARTESIAN_POINT ( 'NONE',  ( 56.65037692655921120, 45.10051614449766078, 2.184720259617097593 ) ) ;
#13844=CARTESIAN_POINT ( 'NONE',  ( 56.65037692655918988, 63.89948385550239607, -2.184720259617163762 ) ) ;
#13850=CARTESIAN_POINT ( 'NONE',  ( 55.69932041026404335, 63.89948385550240317, -1.875703265242203432 ) ) ;
#13853=CARTESIAN_POINT ( 'NONE',  ( 45.31609314410960820, 58.30051614449765651, -6.485486291978072693 ) ) ;
#13854=CARTESIAN_POINT ( 'NONE',  ( 55.11794222512599362, 56.80051614449764941, -3.688883143319583446 ) ) ;
#13866=CARTESIAN_POINT ( 'NONE',  ( 52.29715082351547295, 52.39948385550240317, 6.992620115222774047 ) ) ;
#13870=CARTESIAN_POINT ( 'NONE',  ( 56.79116909180255135, 55.79948385550239465, -4.963592699179005585 ) ) ;
#13872=CARTESIAN_POINT ( 'NONE',  ( 49.97728705011488870, 47.49948385550240459, -6.000000000000000888 ) ) ;
#13875=CARTESIAN_POINT ( 'NONE',  ( 52.25172492374527877, 63.40051614449765793, 7.007379884777203749 ) ) ;
#13877=CARTESIAN_POINT ( 'NONE',  ( 55.96859303347804371, 58.19948385550241454, 4.306917132069425946 ) ) ;
#13882=CARTESIAN_POINT ( 'NONE',  ( 45.86712807150323812, 51.29948385550240175, -5.649768623646098220 ) ) ;
#13893=CARTESIAN_POINT ( 'NONE',  ( 55.69932041026405045, 61.10051614449766788, 1.875703265242156359 ) ) ;
#13899=CARTESIAN_POINT ( 'NONE',  ( 52.57664461997821093, 59.40051614449765793, 8.007379884777206414 ) ) ;
#13914=CARTESIAN_POINT ( 'NONE',  ( 52.29715082351547295, 62.39948385550239607, 6.992620115222774047 ) ) ;
#13916=CARTESIAN_POINT ( 'NONE',  ( 41.58830220609386430, 62.99948385550241170, 0.02388180880523263147 ) ) ;
#13917=CARTESIAN_POINT ( 'NONE',  ( 54.09612160359792199, 61.30051614449766362, 5.676469297603124353 ) ) ;
#13928=CARTESIAN_POINT ( 'NONE',  ( 50.02271294988505446, 48.50051614449765935, -7.000000000000000888 ) ) ;
#13931=CARTESIAN_POINT ( 'NONE',  ( 57.36023556966787851, 61.99948385550241170, -0.02388180880522424582 ) ) ;
#13936=CARTESIAN_POINT ( 'NONE',  ( 53.54508667620428497, 62.29948385550241596, 4.840751629271157874 ) ) ;
#13938=CARTESIAN_POINT ( 'NONE',  ( 47.70284917648453415, 47.39948385550238896, -6.992620115222774047 ) ) ;
#13940=CARTESIAN_POINT ( 'NONE',  ( 45.27934281921082516, 59.70051614449766220, 6.458785618021089192 ) ) ;
#13942=CARTESIAN_POINT ( 'NONE',  ( 57.36023556966787851, 45.00051614449763804, 0.02388180880515038476 ) ) ;
#13955=CARTESIAN_POINT ( 'NONE',  ( 55.96859303347805081, 50.19948385550240744, 4.306917132069425058 ) ) ;
#13959=CARTESIAN_POINT ( 'NONE',  ( 54.68390685589033495, 55.69948385550240744, -6.485486291978119766 ) ) ;
#13961=CARTESIAN_POINT ( 'NONE',  ( 50.02271294988511841, 46.49948385550240459, 6.000000000000000888 ) ) ;
#13964=CARTESIAN_POINT ( 'NONE',  ( 42.63976443033212860, 60.00051614449764514, -0.02388180880514948964 ) ) ;
#13966=CARTESIAN_POINT ( 'NONE',  ( 43.33558569842703179, 61.09948385550240602, -2.141517661632099223 ) ) ;
#13974=CARTESIAN_POINT ( 'NONE',  ( 47.70284917648453415, 51.39948385550238896, -6.992620115222774047 ) ) ;
#13983=CARTESIAN_POINT ( 'NONE',  ( 52.29715082351547295, 46.39948385550240317, 6.992620115222774047 ) ) ;
#13986=CARTESIAN_POINT ( 'NONE',  ( 43.69122665457040000, 64.00051614449765225, -0.02388180880515696977 ) ) ;
#13992=CARTESIAN_POINT ( 'NONE',  ( 52.62207051974829852, 60.60051614449765367, -7.992620115222797139 ) ) ;
#14011=CARTESIAN_POINT ( 'NONE',  ( 49.97728705011488870, 45.49948385550240459, -6.000000000000000888 ) ) ;
#14014=CARTESIAN_POINT ( 'NONE',  ( 57.61547081786812896, 58.09948385550241312, 2.450534656007040901 ) ) ;
#14015=CARTESIAN_POINT ( 'NONE',  ( 44.03140696652198471, 61.80051614449767072, 4.306917132069485454 ) ) ;
#14024=CARTESIAN_POINT ( 'NONE',  ( 54.09612160359792199, 47.30051614449765651, 5.676469297603124353 ) ) ;
#14032=CARTESIAN_POINT ( 'NONE',  ( 51.97223112728254790, 64.39948385550239607, 5.992620115222778487 ) ) ;
#14036=CARTESIAN_POINT ( 'NONE',  ( 52.57664461997821093, 59.40051614449765793, 8.007379884777206414 ) ) ;
#14037=CARTESIAN_POINT ( 'NONE',  ( 55.71335778527780036, 58.90051614449766504, -1.832500667257213056 ) ) ;
#14053=CARTESIAN_POINT ( 'NONE',  ( 56.65037692655918988, 49.89948385550240317, -2.184720259617163762 ) ) ;
#14058=CARTESIAN_POINT ( 'NONE',  ( 49.97728705011486738, 51.49948385550240459, -8.000000000000001776 ) ) ;
#14061=CARTESIAN_POINT ( 'NONE',  ( 49.97728705011488870, 45.49948385550240459, -6.000000000000000888 ) ) ;
#14065=CARTESIAN_POINT ( 'NONE',  ( 44.03140696652198471, 57.80051614449766362, 4.306917132069485454 ) ) ;
#14067=CARTESIAN_POINT ( 'NONE',  ( 43.33558569842703179, 57.09948385550240602, -2.141517661632099223 ) ) ;
#14076=CARTESIAN_POINT ( 'NONE',  ( 56.66441430157296821, 50.09948385550240602, 2.141517661632100111 ) ) ;
#14083=CARTESIAN_POINT ( 'NONE',  ( 44.05948171654945611, 64.20051614449766930, -4.345558710429044069 ) ) ;
#14088=CARTESIAN_POINT ( 'NONE',  ( 53.54508667620424234, 60.70051614449766930, -4.840751629271188961 ) ) ;
#14092=CARTESIAN_POINT ( 'NONE',  ( 45.27934281921082516, 61.70051614449766220, 6.458785618021089192 ) ) ;
#14100=VECTOR ( 'NONE', #1894, 1000.000000000000000 ) ;
#14114=CARTESIAN_POINT ( 'NONE',  ( 44.05948171654949874, 62.79948385550241596, 4.345558710429105354 ) ) ;
#14116=CARTESIAN_POINT ( 'NONE',  ( 57.61547081786812896, 60.09948385550240602, 2.450534656007040901 ) ) ;
#14117=CARTESIAN_POINT ( 'NONE',  ( 47.70284917648459100, 63.60051614449766078, 6.992620115222796251 ) ) ;
#14127=CARTESIAN_POINT ( 'NONE',  ( 55.94051828345054389, 51.20051614449765509, 4.345558710429044957 ) ) ;
#14134=CARTESIAN_POINT ( 'NONE',  ( 45.90387839640214196, 46.69948385550240744, 5.676469297603166098 ) ) ;
#14136=CARTESIAN_POINT ( 'NONE',  ( 56.81924384183006538, 60.80051614449766362, -4.924951120819380357 ) ) ;
#14137=CARTESIAN_POINT ( 'NONE',  ( 50.02271294988506156, 60.50051614449766646, -6.000000000000000888 ) ) ;
#14151=CARTESIAN_POINT ( 'NONE',  ( 44.05948171654949874, 60.79948385550240886, 4.345558710429104465 ) ) ;
#14155=CARTESIAN_POINT ( 'NONE',  ( 50.02271294988513972, 54.49948385550240459, 8.000000000000001776 ) ) ;
#14157=CARTESIAN_POINT ( 'NONE',  ( 54.09612160359786515, 63.69948385550240744, -5.676469297603166098 ) ) ;
#14160=CARTESIAN_POINT ( 'NONE',  ( 57.36023556966787851, 61.00051614449766646, 0.02388180880515038476 ) ) ;
#14161=CARTESIAN_POINT ( 'NONE',  ( 43.69122665457040000, 46.00051614449764514, -0.02388180880515696977 ) ) ;
#14163=CARTESIAN_POINT ( 'NONE',  ( 45.90387839640214196, 58.69948385550240033, 5.676469297603166098 ) ) ;
#14171=CARTESIAN_POINT ( 'NONE',  ( 42.63976443033212860, 50.99948385550240459, 0.02388180880522514787 ) ) ;
#14180=DIRECTION ( 'NONE',  ( 0.9989677110047502362, 0.04542589977017699732, -6.931730960091013400E-15 ) ) ;
#14185=CARTESIAN_POINT ( 'NONE',  ( 43.69122665457040000, 62.00051614449766646, -0.02388180880515696977 ) ) ;
#14208=CARTESIAN_POINT ( 'NONE',  ( 45.86712807150323812, 65.29948385550241596, -5.649768623646098220 ) ) ;
#14210=CARTESIAN_POINT ( 'NONE',  ( 52.25172492374522903, 47.59948385550239891, -7.007379884777225953 ) ) ;
#14211=CARTESIAN_POINT ( 'NONE',  ( 57.36023556966787851, 59.00051614449765935, 0.02388180880515038476 ) ) ;
#14221=CARTESIAN_POINT ( 'NONE',  ( 52.29715082351539479, 54.60051614449766788, -6.992620115222796251 ) ) ;
#14229=CARTESIAN_POINT ( 'NONE',  ( 49.97728705011488159, 45.49948385550240459, -7.000000000000000888 ) ) ;
#14232=CARTESIAN_POINT ( 'NONE',  ( 52.62207051974839089, 48.39948385550240317, 7.992620115222770494 ) ) ;
#14234=CARTESIAN_POINT ( 'NONE',  ( 44.28664221472221385, 63.90051614449765793, 1.832500667257213722 ) ) ;
#14248=CARTESIAN_POINT ( 'NONE',  ( 55.94051828345050836, 57.79948385550240175, -4.345558710429103577 ) ) ;
#14252=CARTESIAN_POINT ( 'NONE',  ( 43.18075615816989199, 55.19948385550240744, -4.924951120819313743 ) ) ;
#14255=CARTESIAN_POINT ( 'NONE',  ( 44.30067958973596376, 50.89948385550240317, 1.875703265242204099 ) ) ;
#14258=CARTESIAN_POINT ( 'NONE',  ( 45.90387839640208512, 62.30051614449766362, -5.676469297603124353 ) ) ;
#14259=CARTESIAN_POINT ( 'NONE',  ( 44.30067958973596376, 60.89948385550241028, 1.875703265242204099 ) ) ;
#14261=CARTESIAN_POINT ( 'NONE',  ( 56.65037692655918988, 59.89948385550241028, -2.184720259617163762 ) ) ;
#14268=CARTESIAN_POINT ( 'NONE',  ( 57.36023556966787851, 59.99948385550240459, -0.02388180880522424582 ) ) ;
#14276=CARTESIAN_POINT ( 'NONE',  ( 45.86712807150329496, 63.70051614449766220, 5.649768623646139964 ) ) ;
#14281=CARTESIAN_POINT ( 'NONE',  ( 48.02776887271750184, 63.60051614449764656, 5.992620115222795363 ) ) ;
#14283=EDGE_CURVE ( 'NONE', #17307, #9631, #2168, .T. ) ;
#14310=CARTESIAN_POINT ( 'NONE',  ( 46.49166364869460466, 50.69948385550240744, 4.867452303228209765 ) ) ;
#14312=CARTESIAN_POINT ( 'NONE',  ( 47.42335538002188144, 64.59948385550241312, 8.007379884777233059 ) ) ;
#14313=CARTESIAN_POINT ( 'NONE',  ( 43.18075615816994173, 47.80051614449764941, 4.924951120819380357 ) ) ;
#14322=CARTESIAN_POINT ( 'NONE',  ( 54.09612160359792199, 51.30051614449766362, 5.676469297603124353 ) ) ;
#14323=CARTESIAN_POINT ( 'NONE',  ( 53.49409602498213445, 45.00000000000000711, -6.629536405711814240 ) ) ;
#14329=CARTESIAN_POINT ( 'NONE',  ( 43.33558569842703179, 49.09948385550240602, -2.141517661632099223 ) ) ;
#14331=CARTESIAN_POINT ( 'NONE',  ( 52.57664461997811856, 49.59948385550241312, -8.007379884777229506 ) ) ;
#14334=CARTESIAN_POINT ( 'NONE',  ( 50.02271294988505446, 44.50051614449765935, -7.000000000000000888 ) ) ;
#14344=ORIENTED_EDGE ( 'NONE', *, *, #17915, .T. ) ;
#14347=CARTESIAN_POINT ( 'NONE',  ( 55.96859303347805081, 56.19948385550240744, 4.306917132069425058 ) ) ;
#14352=VERTEX_POINT ( 'NONE', #6991 ) ;
#14353=CARTESIAN_POINT ( 'NONE',  ( 52.57664461997811856, 59.59948385550240602, -8.007379884777229506 ) ) ;
#14356=CARTESIAN_POINT ( 'NONE',  ( 55.11794222512601493, 48.19948385550240744, 3.688883143319541702 ) ) ;
#14360=CARTESIAN_POINT ( 'NONE',  ( 56.81924384183006538, 46.80051614449766362, -4.924951120819380357 ) ) ;
#14361=CARTESIAN_POINT ( 'NONE',  ( 50.02271294988506156, 44.50051614449765935, -6.000000000000000888 ) ) ;
#14370=CARTESIAN_POINT ( 'NONE',  ( 47.70284917648453415, 59.39948385550241028, -6.992620115222774047 ) ) ;
#14381=CARTESIAN_POINT ( 'NONE',  ( 57.36023556966787851, 53.99948385550239038, -0.02388180880522424582 ) ) ;
#14383=CARTESIAN_POINT ( 'NONE',  ( 42.63976443033212860, 48.00051614449766646, -0.02388180880514948964 ) ) ;
#14403=CARTESIAN_POINT ( 'NONE',  ( 43.69122665457040000, 62.99948385550241170, 0.02388180880521036456 ) ) ;
#14407=CARTESIAN_POINT ( 'NONE',  ( 53.50833635130540955, 51.69948385550241454, -4.867452303228209765 ) ) ;
#14411=CARTESIAN_POINT ( 'NONE',  ( 54.09612160359786515, 45.69948385550240744, -5.676469297603166098 ) ) ;
#14412=CARTESIAN_POINT ( 'NONE',  ( 52.62207051974829852, 44.60051614449766078, -7.992620115222797139 ) ) ;
#14428=CARTESIAN_POINT ( 'NONE',  ( 42.63976443033212149, 56.00051614449765225, -0.02388180880514948964 ) ) ;
#14436=CARTESIAN_POINT ( 'NONE',  ( 52.25172492374522903, 51.59948385550240602, -7.007379884777225953 ) ) ;
#14439=CARTESIAN_POINT ( 'NONE',  ( 57.60143344285433642, 45.89948385550240317, -2.493737253992118319 ) ) ;
#14441=CARTESIAN_POINT ( 'NONE',  ( 49.97728705011495265, 51.50051614449765935, 7.000000000000000888 ) ) ;
#14454=CARTESIAN_POINT ( 'NONE',  ( 47.70284917648453415, 59.39948385550241028, -6.992620115222774047 ) ) ;
#14458=CARTESIAN_POINT ( 'NONE',  ( 42.38452918213188525, 59.09948385550240602, -2.450534656007040013 ) ) ;
#14461=CARTESIAN_POINT ( 'NONE',  ( 48.07319477248768180, 50.59948385550240602, 6.007379884777225953 ) ) ;
#14465=CARTESIAN_POINT ( 'NONE',  ( 57.60143344285435774, 49.10051614449766788, 2.493737253992045044 ) ) ;
#14466=CARTESIAN_POINT ( 'NONE',  ( 44.91013252490150620, 48.20051614449766930, -3.727524721679154940 ) ) ;
#14475=CARTESIAN_POINT ( 'NONE',  ( 54.09612160359786515, 59.69948385550240033, -5.676469297603166098 ) ) ;
#14483=CARTESIAN_POINT ( 'NONE',  ( 43.33558569842703179, 49.09948385550240602, -2.141517661632099223 ) ) ;
#14485=CARTESIAN_POINT ( 'NONE',  ( 52.29715082351538769, 50.60051614449766788, -6.992620115222796251 ) ) ;
#14495=EDGE_LOOP ( 'NONE', ( #7536, #18494, #3961 ) ) ;
#14501=CARTESIAN_POINT ( 'NONE',  ( 44.28664221472221385, 47.90051614449765793, 1.832500667257213722 ) ) ;
#14504=CARTESIAN_POINT ( 'NONE',  ( 44.28664221472220675, 53.09948385550240602, -1.832500667257165317 ) ) ;
#14506=CARTESIAN_POINT ( 'NONE',  ( 47.70284917648453415, 47.39948385550238896, -6.992620115222774047 ) ) ;
#14507=CARTESIAN_POINT ( 'NONE',  ( 52.62207051974829852, 48.60051614449766788, -7.992620115222797139 ) ) ;
#14516=CARTESIAN_POINT ( 'NONE',  ( 55.96859303347802239, 50.80051614449766362, -4.306917132069484566 ) ) ;
#14522=CARTESIAN_POINT ( 'NONE',  ( 55.96859303347804371, 50.19948385550240744, 4.306917132069425946 ) ) ;
#14524=CARTESIAN_POINT ( 'NONE',  ( 52.57664461997811856, 47.59948385550239891, -8.007379884777229506 ) ) ;
#14526=CARTESIAN_POINT ( 'NONE',  ( 44.03140696652198471, 47.80051614449764230, 4.306917132069485454 ) ) ;
#14543=CARTESIAN_POINT ( 'NONE',  ( 47.42335538002188144, 56.59948385550239891, 8.007379884777233059 ) ) ;
#14546=CARTESIAN_POINT ( 'NONE',  ( 48.02776887271745210, 53.39948385550241028, -5.992620115222778487 ) ) ;
#14549=CARTESIAN_POINT ( 'NONE',  ( 42.38452918213190657, 47.90051614449765793, 2.450534656007115508 ) ) ;
#14552=CARTESIAN_POINT ( 'NONE',  ( 44.91013252490150620, 50.20051614449766220, -3.727524721679154940 ) ) ;
#14555=DIRECTION ( 'NONE',  ( -0.9989677110047502362, -0.04542589977017699732, 6.931730960091013400E-15 ) ) ;
#14557=( BOUNDED_SURFACE ( )  B_SPLINE_SURFACE ( 3, 2, ( 
 ( #14229, #15521, #17012, #17300, #9439, #17199, #9817, #12379, #2098, #2004, #9623, #12578, #14134, #7966, #3856, #6492, #11006, #8057, #3756, #13938, #15720, #15618, #618, #18586, #18388, #11094, #12772, #2197, #10904, #2300, #8254, #815, #18773, #11292, #11773, #7079, #14329, #913, #14722, #1309, #8555, #16113, #2398, #9915, #2692, #1018, #19070, #14522, #6980, #12960, #8351, #16206, #5809, #11386, #1205, #5716, #8646, #6881, #18968, #5612, #19175, #14436, #17394, #1108, #19270, #15914, #5509, #11482, #13254, #17491, #3954, #18874, #11585, #13062, #4053, #10015, #2501, #13159, #5413, #8745, #16018, #2603, #17778, #8455, #11683, #4337, #12872, #17597, #4151, #2783, #10116, #17686, #7278, #10305, #14619, #7180, #4239, #10202, #13735, #18269, #321, #4539, #4824, #19369, #11977, #16311, #2885, #3173, #10406, #12170, #8845, #29, #6197, #18178, #14821, #9032, #6296, #18074, #1497, #13451, #17981, #1401, #7377, #13349, #216, #10498, #12271, #15019, #7661, #7470, #13642, #9134, #16502, #17881, #6015, #4736, #15118, #5904, #11873, #14921, #6103, #3076, #15212, #9222, #10697, #4638, #1694, #1598, #1789, #7568, #4446, #16406, #2973, #13550, #16601, #7760, #8938, #123, #16697, #12073, #10597, #3261, #16890, #3638, #12653, #3547, #413, #1982, #7946, #13914, #3734, #2280, #9597, #14114, #18660, #6571, #12452, #15496, #5008, #15405, #6671, #18565, #8233, #501, #4914, #6377, #3453, #18462, #796, #10985, #6472, #16992, #9506, #11166, #2074, #10884, #5197, #6767, #14208, #8035, #12357 ),
 ( #14011, #2175, #15595, #596, #18367, #12558, #17174, #5107, #9418, #11077, #17082, #8137, #700, #12750, #9700, #15701, #18746, #10787, #16790, #3356, #9318, #15307, #1888, #7859, #13832, #4217, #6857, #3838, #1187, #8330, #11265, #18854, #10184, #14698, #9993, #17278, #9799, #17662, #16184, #11460, #19047, #5293, #12844, #5590, #3935, #2581, #17471, #9893, #15893, #15795, #19149, #8724, #14310, #4128, #8626, #11560, #5395, #888, #11367, #6962, #1287, #12941, #14407, #18950, #2478, #5695, #4030, #17374, #13139, #7261, #13235, #5490, #8430, #995, #11661, #1089, #14504, #2376, #2765, #7059, #8534, #15990, #13040, #17574, #10095, #16090, #14599, #2673, #7160, #16388, #1378, #10387, #2953, #2862, #7739, #17962, #16483, #1473, #14996, #19245, #106, #5993, #4615, #1577, #12055, #1768, #12149, #8918, #17860, #19345, #7549, #18054, #200, #4422, #4520, #13534, #3052, #10479, #5886, #6177, #5787, #10574, #9011, #9115, #11959, #13325, #16578, #7352, #18153, #6084, #3149, #15102, #11751, #7451, #11853, #14899, #1679, #17758, #16680, #13432, #7642, #13622, #4712, #10675, #3246, #9205, #15191, #7, #4317, #10286, #16289, #8826, #14799, #6718, #14259, #12902, #2533, #17228, #17329, #296, #11124, #3793, #394, #6818, #15843, #12701, #3336, #5151, #17130, #3689, #6916, #5442, #12804, #3887, #2428, #9757, #15650, #18704, #8193, #18611, #9843, #2328, #11419, #9653, #12247, #8380, #16771, #6268, #7833, #18904, #3980, #5250, #18252, #4808, #17421, #9944, #744, #8281, #13717, #1867, #842 ),
 ( #14361, #15943, #9297, #18804, #945, #5354, #10771, #12602, #15750, #11326, #6362, #15287, #11221, #13811, #2235, #14161, #17625, #19400, #4175, #4082, #5536, #11706, #14647, #19098, #5639, #16047, #19299, #11511, #14852, #10141, #16144, #17910, #10049, #5836, #10430, #1046, #2629, #14466, #8870, #17713, #4367, #1430, #7403, #2909, #7012, #11615, #12991, #5938, #16434, #11900, #2721, #8490, #17521, #8676, #18998, #8583, #14750, #14552, #10331, #1136, #1233, #17811, #16337, #7107, #7206, #4469, #10235, #13089, #13190, #19203, #5742, #4269, #16236, #11806, #2810, #8772, #1334, #13377, #7308, #13283, #15233, #18103, #4566, #7592, #10810, #4664, #10525, #18205, #1717, #3282, #16529, #18390, #1631, #13572, #6127, #7783, #3102, #16814, #4762, #146, #15139, #4936, #10623, #1915, #9058, #7685, #9245, #7881, #10907, #6222, #6321, #8962, #12097, #12195, #15049, #1813, #4849, #13665, #12001, #16630, #3199, #9161, #15334, #13854, #13761, #12294, #3377, #10722, #240, #16721, #346, #18294, #9340, #434, #6404, #12383, #3003, #18006, #14945, #1525, #7499, #13481, #57, #6037, #14037, #17304, #15622, #17017, #5323, #6888, #917, #5128, #12475, #622, #11298, #12678, #6693, #2007, #3861, #18679, #14137, #3479, #18488, #12581, #5222, #9821, #820, #9627, #8062, #6599, #5037, #18590, #11099, #523, #5417, #2202, #723, #17106, #11196, #16915, #17202, #3664, #2304, #3760, #9727, #18879, #15822, #8164, #15525, #3567, #15723, #8257, #2403, #2101, #14234, #6790, #12776, #18777, #9533, #8356, #9443 ),
 ( #14334, #15428, #12876, #7970, #6496, #13942, #11009, #5721, #11390, #10020, #14622, #8749, #4057, #6985, #4156, #8850, #18973, #8561, #1112, #2890, #7083, #12964, #8460, #1209, #17600, #2608, #10120, #11686, #10309, #19374, #7184, #14727, #17400, #14526, #13164, #17495, #4244, #13259, #16117, #1022, #13066, #19074, #5616, #4341, #14826, #10207, #1312, #19274, #19180, #11590, #2697, #8650, #16021, #7283, #17690, #1405, #16210, #5513, #11486, #2788, #5813, #7381, #11779, #17783, #16315, #13354, #3958, #9920, #15920, #2505, #14441, #9321, #13554, #1501, #9036, #13739, #1698, #15122, #10411, #324, #7665, #3178, #11877, #7475, #1604, #13646, #6300, #9225, #18079, #16507, #3080, #13456, #15024, #7572, #8942, #13835, #4642, #9139, #127, #221, #5910, #6201, #12077, #10702, #12175, #18182, #7862, #18273, #6107, #4543, #6019, #4741, #16701, #12274, #10502, #10603, #3264, #15215, #16605, #11981, #4828, #17886, #1794, #7763, #10790, #16793, #34, #3359, #17985, #15310, #1891, #4450, #16410, #2977, #14926, #505, #12455, #12656, #12361, #17281, #18466, #9601, #6575, #18750, #12753, #14211, #8142, #5200, #5011, #5297, #2077, #3841, #9422, #18370, #15408, #12561, #9802, #7949, #16995, #9509, #11271, #15499, #1985, #16894, #3641, #18568, #10988, #3550, #13917, #11170, #3456, #6770, #8040, #14015, #15798, #6476, #17178, #2379, #4918, #600, #6381, #799, #15599, #15704, #8333, #416, #10887, #5110, #11080, #17085, #2179, #14117, #703, #6674, #18663, #3739, #9704, #2283, #8237, #1191, #8434 ),
 ( #13043, #14412, #2769, #4321, #17761, #2584, #9896, #17475, #8727, #10098, #4131, #18857, #14702, #16093, #11564, #891, #15897, #9997, #2676, #1292, #17665, #7062, #5493, #11463, #2481, #4034, #15995, #17377, #2866, #19051, #17579, #8537, #8629, #14313, #14602, #1092, #19155, #7163, #13143, #16293, #7265, #14507, #12944, #998, #5698, #11664, #13238, #18953, #5594, #4220, #10187, #16187, #6965, #19248, #6861, #5790, #11754, #10289, #12849, #5398, #11370, #3938, #7741, #1580, #6180, #3152, #8829, #10482, #8921, #1476, #1681, #1382, #6271, #7454, #16774, #7553, #6087, #16485, #4617, #14803, #9118, #14999, #13625, #10576, #7645, #10773, #1770, #5999, #13435, #14902, #16580, #202, #9208, #11, #13536, #15104, #12057, #108, #11962, #15193, #7356, #12151, #18057, #18156, #4714, #2958, #10679, #10390, #13720, #16682, #3248, #299, #13328, #3054, #17965, #4524, #12251, #19348, #18254, #9013, #4810, #5890, #11856, #17864, #4427, #16391, #5090, #9394, #6654, #483, #5176, #396, #15289, #4988, #6551, #12632, #9680, #15475, #3616, #9299, #1964, #2057, #16870, #12536, #15576, #10964, #6364, #15385, #7926, #13899, #682, #18636, #18549, #17064, #2155, #8018, #6453, #16973, #12434, #18442, #8117, #13992, #11147, #3525, #4900, #12341, #10863, #9488, #17155, #578, #11056, #9581, #14092, #3717, #3338, #1870, #7835, #13815, #18351, #3435, #16450, #4583, #9262, #16650, #10643, #5957, #15250, #3217, #18122, #7422, #3019, #16548, #9180, #1831, #4777, #13590, #12018, #18022, #8981, #10540, #3121 ),
 ( #1544, #13502, #13681, #13399, #18313, #77, #15159, #7612, #366, #13777, #7799, #1738, #6239, #6055, #6337, #9077, #4869, #10446, #18587, #165, #7702, #12309, #9357, #4685, #10739, #11923, #15070, #259, #7517, #12212, #3304, #6142, #14965, #1650, #12113, #18225, #10830, #16834, #16740, #3396, #1446, #17931, #4489, #641, #9549, #545, #11215, #3681, #12797, #6516, #9460, #10926, #2026, #17031, #5345, #3587, #5054, #15541, #12494, #15741, #14058, #15445, #3783, #11317, #18797, #2119, #16931, #18506, #9746, #11116, #5144, #451, #2320, #17123, #12596, #1934, #3496, #11025, #9647, #8273, #18697, #8082, #6618, #18605, #7986, #15642, #2224, #18410, #3878, #8183, #14155, #738, #6711, #15350, #12694, #5242, #17221, #14252, #836, #17321, #6809, #7898, #13959, #13870, #6423, #12403, #4953, #8479, #8576, #4168, #7097, #14543, #9937, #10226, #15837, #14638, #19091, #19195, #2622, #3973, #7199, #11409, #8764, #15937, #14742, #19290, #1127, #2421, #8373, #2803, #1328, #16038, #10133, #9836, #17414, #16135, #14458, #13082, #5632, #1040, #7003, #14353, #4261, #13274, #18897, #8666, #13181, #2714, #937, #12981, #11606, #5735, #2524, #5432, #17616, #7300, #18989, #5528, #11504, #5829, #17514, #4074, #6906, #1225, #11698, #10039, #17706, #16227, #11797, #12895, #17802, #13700, #9191, #8997, #4597, #10558, #13606, #4506, #1364, #2939, #8901, #14882, #4700, #3231, #16563, #15086, #185, #7533, #13416, #16467, #5974, #16373, #7627, #92, #15175, #1458, #5873, #7337, #17844, #3540, #1753 ),
 ( #11839, #6158, #7719, #276, #11943, #13314, #7437, #12131, #13518, #1563, #16271, #18138, #6072, #14980, #17744, #19331, #17947, #12039, #10660, #1664, #10463, #3034, #18037, #4404, #3137, #9098, #14785, #11739, #16667, #4303, #10268, #2846, #8812, #10373, #12417, #11039, #8003, #18526, #8202, #18620, #3414, #4884, #6349, #1848, #1948, #2041, #14076, #9566, #18427, #16853, #9374, #7815, #15366, #7910, #9279, #14171, #4969, #3510, #13882, #13974, #6253, #6532, #10944, #17045, #561, #5069, #12231, #5160, #466, #10847, #12325, #12516, #3601, #6634, #6438, #16951, #15558, #9473, #15459, #18331, #12613, #18239, #2138, #8098, #663, #11132, #381, #17140, #13795, #3701, #9662, #15659, #2248, #4794, #10757, #16754, #3321, #15269, #12711, #17634, #18815, #9953, #6927, #19109, #13100, #14561, #8500, #5546, #5361, #5649, #2438, #4183, #9769, #18714, #12909, #1053, #11622, #8686, #3990, #4090, #2730, #10150, #17431, #13004, #19009, #2639, #18913, #15762, #11334, #17342, #3897, #16151, #754, #11522, #10057, #8591, #15954, #8390, #5453, #14370, #9856, #16056, #14475, #6727, #15855, #14268, #2340, #6826, #954, #5261, #11428, #2541, #7022, #17530, #1146, #7119, #852, #11231, #17237, #3802, #8292, #12812, #17821, #3112, #10437, #4478, #19211, #9066, #16441, #11913, #1243, #15060, #3010, #69, #19307, #13580, #16345, #12104, #4278, #13197, #7412, #14955, #155, #3209, #17920, #18013, #16640, #18112, #8972, #7508, #13492, #16537, #13387, #10244, #5846, #11815, #4379, #7603, #6133, #6045, #4574 ) ),
 .UNSPECIFIED., .T., .F., .T. ) 
 B_SPLINE_SURFACE_WITH_KNOTS ( ( 4, 3, 4 ),
 ( 3, 2, 2, 2, 2, 2, 2, 2, 2, 2, 2, 2, 2, 2, 2, 2, 2, 2, 2, 2, 2, 2, 2, 2, 2, 2, 2, 2, 2, 2, 2, 2, 2, 2, 2, 2, 2, 2, 2, 2, 2, 2, 2, 2, 2, 2, 2, 2, 2, 2, 2, 2, 2, 2, 2, 2, 2, 2, 2, 2, 2, 2, 2, 2, 2, 2, 2, 2, 2, 2, 2, 2, 2, 2, 2, 2, 2, 2, 2, 2, 2, 2, 2, 2, 2, 2, 2, 2, 2, 2, 2, 2, 2, 2, 2, 2, 2, 2, 2, 2, 3 ),
 ( 0.000000000000000000, 0.5000000000000000000, 1.000000000000000000 ),
 ( 0.000000000000000000, 0.01000000000000000021, 0.02000000000000000042, 0.02999999999999999889, 0.04000000000000000083, 0.05000000000000000278, 0.05999999999999999778, 0.07000000000000000666, 0.08000000000000000167, 0.08999999999999999667, 0.1000000000000000056, 0.1100000000000000006, 0.1199999999999999956, 0.1300000000000000044, 0.1400000000000000133, 0.1499999999999999944, 0.1600000000000000033, 0.1700000000000000122, 0.1799999999999999933, 0.1900000000000000022, 0.2000000000000000111, 0.2099999999999999922, 0.2200000000000000011, 0.2300000000000000100, 0.2399999999999999911, 0.2500000000000000000, 0.2600000000000000089, 0.2700000000000000178, 0.2800000000000000266, 0.2899999999999999800, 0.2999999999999999889, 0.3099999999999999978, 0.3200000000000000067, 0.3300000000000000155, 0.3400000000000000244, 0.3499999999999999778, 0.3599999999999999867, 0.3699999999999999956, 0.3800000000000000044, 0.3900000000000000133, 0.4000000000000000222, 0.4099999999999999756, 0.4199999999999999845, 0.4299999999999999933, 0.4400000000000000022, 0.4500000000000000111, 0.4600000000000000200, 0.4699999999999999734, 0.4799999999999999822, 0.4899999999999999911, 0.5000000000000000000, 0.5100000000000000089, 0.5200000000000000178, 0.5300000000000000266, 0.5400000000000000355, 0.5500000000000000444, 0.5600000000000000533, 0.5699999999999999512, 0.5799999999999999600, 0.5899999999999999689, 0.5999999999999999778, 0.6099999999999999867, 0.6199999999999999956, 0.6300000000000000044, 0.6400000000000000133, 0.6500000000000000222, 0.6600000000000000311, 0.6700000000000000400, 0.6800000000000000488, 0.6899999999999999467, 0.6999999999999999556, 0.7099999999999999645, 0.7199999999999999734, 0.7299999999999999822, 0.7399999999999999911, 0.7500000000000000000, 0.7600000000000000089, 0.7700000000000000178, 0.7800000000000000266, 0.7900000000000000355, 0.8000000000000000444, 0.8100000000000000533, 0.8199999999999999512, 0.8299999999999999600, 0.8399999999999999689, 0.8499999999999999778, 0.8599999999999999867, 0.8699999999999999956, 0.8800000000000000044, 0.8900000000000000133, 0.9000000000000000222, 0.9100000000000000311, 0.9200000000000000400, 0.9300000000000000488, 0.9399999999999999467, 0.9499999999999999556, 0.9599999999999999645, 0.9699999999999999734, 0.9799999999999999822, 0.9899999999999999911, 1.000000000000000000 ),
 .UNSPECIFIED. ) 
 GEOMETRIC_REPRESENTATION_ITEM ( )  RATIONAL_B_SPLINE_SURFACE ( (
 ( 1.000000000000000000, 0.9510565162951535312, 1.000000000000000000, 0.9510565162951535312, 1.000000000000000000, 0.9510565162951535312, 1.000000000000000000, 0.9510565162951535312, 1.000000000000000000, 0.9510565162951535312, 1.000000000000000000, 0.9510565162951535312, 1.000000000000000000, 0.9510565162951535312, 1.000000000000000000, 0.9510565162951535312, 1.000000000000000000, 0.9510565162951535312, 1.000000000000000000, 0.9510565162951535312, 1.000000000000000000, 0.9510565162951535312, 1.000000000000000000, 0.9510565162951535312, 1.000000000000000000, 0.9510565162951535312, 1.000000000000000000, 0.9510565162951535312, 1.000000000000000000, 0.9510565162951535312, 1.000000000000000000, 0.9510565162951535312, 1.000000000000000000, 0.9510565162951535312, 1.000000000000000000, 0.9510565162951535312, 1.000000000000000000, 0.9510565162951535312, 1.000000000000000000, 0.9510565162951535312, 1.000000000000000000, 0.9510565162951535312, 1.000000000000000000, 0.9510565162951535312, 1.000000000000000000, 0.9510565162951535312, 1.000000000000000000, 0.9510565162951535312, 1.000000000000000000, 0.9510565162951535312, 1.000000000000000000, 0.9510565162951535312, 1.000000000000000000, 0.9510565162951535312, 1.000000000000000000, 0.9510565162951535312, 1.000000000000000000, 0.9510565162951535312, 1.000000000000000000, 0.9510565162951535312, 1.000000000000000000, 0.9510565162951535312, 1.000000000000000000, 0.9510565162951535312, 1.000000000000000000, 0.9510565162951535312, 1.000000000000000000, 0.9510565162951535312, 1.000000000000000000, 0.9510565162951535312, 1.000000000000000000, 0.9510565162951535312, 1.000000000000000000, 0.9510565162951535312, 1.000000000000000000, 0.9510565162951535312, 1.000000000000000000, 0.9510565162951535312, 1.000000000000000000, 0.9510565162951535312, 1.000000000000000000, 0.9510565162951535312, 1.000000000000000000, 0.9510565162951535312, 1.000000000000000000, 0.9510565162951535312, 1.000000000000000000, 0.9510565162951535312, 1.000000000000000000, 0.9510565162951535312, 1.000000000000000000, 0.9510565162951535312, 1.000000000000000000, 0.9510565162951535312, 1.000000000000000000, 0.9510565162951535312, 1.000000000000000000, 0.9510565162951535312, 1.000000000000000000, 0.9510565162951535312, 1.000000000000000000, 0.9510565162951535312, 1.000000000000000000, 0.9510565162951535312, 1.000000000000000000, 0.9510565162951535312, 1.000000000000000000, 0.9510565162951535312, 1.000000000000000000, 0.9510565162951535312, 1.000000000000000000, 0.9510565162951535312, 1.000000000000000000, 0.9510565162951535312, 1.000000000000000000, 0.9510565162951535312, 1.000000000000000000, 0.9510565162951535312, 1.000000000000000000, 0.9510565162951535312, 1.000000000000000000, 0.9510565162951535312, 1.000000000000000000, 0.9510565162951535312, 1.000000000000000000, 0.9510565162951535312, 1.000000000000000000, 0.9510565162951535312, 1.000000000000000000, 0.9510565162951535312, 1.000000000000000000, 0.9510565162951535312, 1.000000000000000000, 0.9510565162951535312, 1.000000000000000000, 0.9510565162951535312, 1.000000000000000000, 0.9510565162951535312, 1.000000000000000000, 0.9510565162951535312, 1.000000000000000000, 0.9510565162951535312, 1.000000000000000000, 0.9510565162951535312, 1.000000000000000000, 0.9510565162951535312, 1.000000000000000000, 0.9510565162951535312, 1.000000000000000000, 0.9510565162951535312, 1.000000000000000000, 0.9510565162951535312, 1.000000000000000000, 0.9510565162951535312, 1.000000000000000000, 0.9510565162951535312, 1.000000000000000000, 0.9510565162951535312, 1.000000000000000000, 0.9510565162951535312, 1.000000000000000000, 0.9510565162951535312, 1.000000000000000000, 0.9510565162951535312, 1.000000000000000000, 0.9510565162951535312, 1.000000000000000000, 0.9510565162951535312, 1.000000000000000000, 0.9510565162951535312, 1.000000000000000000, 0.9510565162951535312, 1.000000000000000000, 0.9510565162951535312, 1.000000000000000000, 0.9510565162951535312, 1.000000000000000000, 0.9510565162951535312, 1.000000000000000000, 0.9510565162951535312, 1.000000000000000000, 0.9510565162951535312, 1.000000000000000000, 0.9510565162951535312, 1.000000000000000000, 0.9510565162951535312, 1.000000000000000000, 0.9510565162951535312, 1.000000000000000000, 0.9510565162951535312, 1.000000000000000000, 0.9510565162951535312, 1.000000000000000000, 0.9510565162951535312, 1.000000000000000000, 0.9510565162951535312, 1.000000000000000000, 0.9510565162951535312, 1.000000000000000000, 0.9510565162951535312, 1.000000000000000000),
 ( 0.3333333333333333703, 0.3170188387650512141, 0.3333333333333333703, 0.3170188387650512141, 0.3333333333333333703, 0.3170188387650512141, 0.3333333333333333703, 0.3170188387650512141, 0.3333333333333333703, 0.3170188387650512141, 0.3333333333333333703, 0.3170188387650512141, 0.3333333333333333703, 0.3170188387650512141, 0.3333333333333333703, 0.3170188387650512141, 0.3333333333333333703, 0.3170188387650512141, 0.3333333333333333703, 0.3170188387650512141, 0.3333333333333333703, 0.3170188387650512141, 0.3333333333333333703, 0.3170188387650512141, 0.3333333333333333703, 0.3170188387650512141, 0.3333333333333333703, 0.3170188387650512141, 0.3333333333333333703, 0.3170188387650512141, 0.3333333333333333703, 0.3170188387650512141, 0.3333333333333333703, 0.3170188387650512141, 0.3333333333333333703, 0.3170188387650512141, 0.3333333333333333703, 0.3170188387650512141, 0.3333333333333333703, 0.3170188387650512141, 0.3333333333333333703, 0.3170188387650512141, 0.3333333333333333703, 0.3170188387650512141, 0.3333333333333333703, 0.3170188387650512141, 0.3333333333333333703, 0.3170188387650512141, 0.3333333333333333703, 0.3170188387650512141, 0.3333333333333333703, 0.3170188387650512141, 0.3333333333333333703, 0.3170188387650512141, 0.3333333333333333703, 0.3170188387650512141, 0.3333333333333333703, 0.3170188387650512141, 0.3333333333333333703, 0.3170188387650512141, 0.3333333333333333703, 0.3170188387650512141, 0.3333333333333333703, 0.3170188387650512141, 0.3333333333333333703, 0.3170188387650512141, 0.3333333333333333703, 0.3170188387650512141, 0.3333333333333333703, 0.3170188387650512141, 0.3333333333333333703, 0.3170188387650512141, 0.3333333333333333703, 0.3170188387650512141, 0.3333333333333333703, 0.3170188387650512141, 0.3333333333333333703, 0.3170188387650512141, 0.3333333333333333703, 0.3170188387650512141, 0.3333333333333333703, 0.3170188387650512141, 0.3333333333333333703, 0.3170188387650512141, 0.3333333333333333703, 0.3170188387650512141, 0.3333333333333333703, 0.3170188387650512141, 0.3333333333333333703, 0.3170188387650512141, 0.3333333333333333703, 0.3170188387650512141, 0.3333333333333333703, 0.3170188387650512141, 0.3333333333333333703, 0.3170188387650512141, 0.3333333333333333703, 0.3170188387650512141, 0.3333333333333333703, 0.3170188387650512141, 0.3333333333333333703, 0.3170188387650512141, 0.3333333333333333703, 0.3170188387650512141, 0.3333333333333333703, 0.3170188387650512141, 0.3333333333333333703, 0.3170188387650512141, 0.3333333333333333703, 0.3170188387650512141, 0.3333333333333333703, 0.3170188387650512141, 0.3333333333333333703, 0.3170188387650512141, 0.3333333333333333703, 0.3170188387650512141, 0.3333333333333333703, 0.3170188387650512141, 0.3333333333333333703, 0.3170188387650512141, 0.3333333333333333703, 0.3170188387650512141, 0.3333333333333333703, 0.3170188387650512141, 0.3333333333333333703, 0.3170188387650512141, 0.3333333333333333703, 0.3170188387650512141, 0.3333333333333333703, 0.3170188387650512141, 0.3333333333333333703, 0.3170188387650512141, 0.3333333333333333703, 0.3170188387650512141, 0.3333333333333333703, 0.3170188387650512141, 0.3333333333333333703, 0.3170188387650512141, 0.3333333333333333703, 0.3170188387650512141, 0.3333333333333333703, 0.3170188387650512141, 0.3333333333333333703, 0.3170188387650512141, 0.3333333333333333703, 0.3170188387650512141, 0.3333333333333333703, 0.3170188387650512141, 0.3333333333333333703, 0.3170188387650512141, 0.3333333333333333703, 0.3170188387650512141, 0.3333333333333333703, 0.3170188387650512141, 0.3333333333333333703, 0.3170188387650512141, 0.3333333333333333703, 0.3170188387650512141, 0.3333333333333333703, 0.3170188387650512141, 0.3333333333333333703, 0.3170188387650512141, 0.3333333333333333703, 0.3170188387650512141, 0.3333333333333333703, 0.3170188387650512141, 0.3333333333333333703, 0.3170188387650512141, 0.3333333333333333703, 0.3170188387650512141, 0.3333333333333333703, 0.3170188387650512141, 0.3333333333333333703, 0.3170188387650512141, 0.3333333333333333703, 0.3170188387650512141, 0.3333333333333333703, 0.3170188387650512141, 0.3333333333333333703, 0.3170188387650512141, 0.3333333333333333703, 0.3170188387650512141, 0.3333333333333333703, 0.3170188387650512141, 0.3333333333333333703, 0.3170188387650512141, 0.3333333333333333703, 0.3170188387650512141, 0.3333333333333333703, 0.3170188387650512141, 0.3333333333333333703, 0.3170188387650512141, 0.3333333333333333703, 0.3170188387650512141, 0.3333333333333333703, 0.3170188387650512141, 0.3333333333333333703, 0.3170188387650512141, 0.3333333333333333703, 0.3170188387650512141, 0.3333333333333333703),
 ( 0.3333333333333333703, 0.3170188387650512141, 0.3333333333333333703, 0.3170188387650512141, 0.3333333333333333703, 0.3170188387650512141, 0.3333333333333333703, 0.3170188387650512141, 0.3333333333333333703, 0.3170188387650512141, 0.3333333333333333703, 0.3170188387650512141, 0.3333333333333333703, 0.3170188387650512141, 0.3333333333333333703, 0.3170188387650512141, 0.3333333333333333703, 0.3170188387650512141, 0.3333333333333333703, 0.3170188387650512141, 0.3333333333333333703, 0.3170188387650512141, 0.3333333333333333703, 0.3170188387650512141, 0.3333333333333333703, 0.3170188387650512141, 0.3333333333333333703, 0.3170188387650512141, 0.3333333333333333703, 0.3170188387650512141, 0.3333333333333333703, 0.3170188387650512141, 0.3333333333333333703, 0.3170188387650512141, 0.3333333333333333703, 0.3170188387650512141, 0.3333333333333333703, 0.3170188387650512141, 0.3333333333333333703, 0.3170188387650512141, 0.3333333333333333703, 0.3170188387650512141, 0.3333333333333333703, 0.3170188387650512141, 0.3333333333333333703, 0.3170188387650512141, 0.3333333333333333703, 0.3170188387650512141, 0.3333333333333333703, 0.3170188387650512141, 0.3333333333333333703, 0.3170188387650512141, 0.3333333333333333703, 0.3170188387650512141, 0.3333333333333333703, 0.3170188387650512141, 0.3333333333333333703, 0.3170188387650512141, 0.3333333333333333703, 0.3170188387650512141, 0.3333333333333333703, 0.3170188387650512141, 0.3333333333333333703, 0.3170188387650512141, 0.3333333333333333703, 0.3170188387650512141, 0.3333333333333333703, 0.3170188387650512141, 0.3333333333333333703, 0.3170188387650512141, 0.3333333333333333703, 0.3170188387650512141, 0.3333333333333333703, 0.3170188387650512141, 0.3333333333333333703, 0.3170188387650512141, 0.3333333333333333703, 0.3170188387650512141, 0.3333333333333333703, 0.3170188387650512141, 0.3333333333333333703, 0.3170188387650512141, 0.3333333333333333703, 0.3170188387650512141, 0.3333333333333333703, 0.3170188387650512141, 0.3333333333333333703, 0.3170188387650512141, 0.3333333333333333703, 0.3170188387650512141, 0.3333333333333333703, 0.3170188387650512141, 0.3333333333333333703, 0.3170188387650512141, 0.3333333333333333703, 0.3170188387650512141, 0.3333333333333333703, 0.3170188387650512141, 0.3333333333333333703, 0.3170188387650512141, 0.3333333333333333703, 0.3170188387650512141, 0.3333333333333333703, 0.3170188387650512141, 0.3333333333333333703, 0.3170188387650512141, 0.3333333333333333703, 0.3170188387650512141, 0.3333333333333333703, 0.3170188387650512141, 0.3333333333333333703, 0.3170188387650512141, 0.3333333333333333703, 0.3170188387650512141, 0.3333333333333333703, 0.3170188387650512141, 0.3333333333333333703, 0.3170188387650512141, 0.3333333333333333703, 0.3170188387650512141, 0.3333333333333333703, 0.3170188387650512141, 0.3333333333333333703, 0.3170188387650512141, 0.3333333333333333703, 0.3170188387650512141, 0.3333333333333333703, 0.3170188387650512141, 0.3333333333333333703, 0.3170188387650512141, 0.3333333333333333703, 0.3170188387650512141, 0.3333333333333333703, 0.3170188387650512141, 0.3333333333333333703, 0.3170188387650512141, 0.3333333333333333703, 0.3170188387650512141, 0.3333333333333333703, 0.3170188387650512141, 0.3333333333333333703, 0.3170188387650512141, 0.3333333333333333703, 0.3170188387650512141, 0.3333333333333333703, 0.3170188387650512141, 0.3333333333333333703, 0.3170188387650512141, 0.3333333333333333703, 0.3170188387650512141, 0.3333333333333333703, 0.3170188387650512141, 0.3333333333333333703, 0.3170188387650512141, 0.3333333333333333703, 0.3170188387650512141, 0.3333333333333333703, 0.3170188387650512141, 0.3333333333333333703, 0.3170188387650512141, 0.3333333333333333703, 0.3170188387650512141, 0.3333333333333333703, 0.3170188387650512141, 0.3333333333333333703, 0.3170188387650512141, 0.3333333333333333703, 0.3170188387650512141, 0.3333333333333333703, 0.3170188387650512141, 0.3333333333333333703, 0.3170188387650512141, 0.3333333333333333703, 0.3170188387650512141, 0.3333333333333333703, 0.3170188387650512141, 0.3333333333333333703, 0.3170188387650512141, 0.3333333333333333703, 0.3170188387650512141, 0.3333333333333333703, 0.3170188387650512141, 0.3333333333333333703, 0.3170188387650512141, 0.3333333333333333703, 0.3170188387650512141, 0.3333333333333333703, 0.3170188387650512141, 0.3333333333333333703, 0.3170188387650512141, 0.3333333333333333703, 0.3170188387650512141, 0.3333333333333333703, 0.3170188387650512141, 0.3333333333333333703, 0.3170188387650512141, 0.3333333333333333703, 0.3170188387650512141, 0.3333333333333333703, 0.3170188387650512141, 0.3333333333333333703),
 ( 1.000000000000000000, 0.9510565162951535312, 1.000000000000000000, 0.9510565162951535312, 1.000000000000000000, 0.9510565162951535312, 1.000000000000000000, 0.9510565162951535312, 1.000000000000000000, 0.9510565162951535312, 1.000000000000000000, 0.9510565162951535312, 1.000000000000000000, 0.9510565162951535312, 1.000000000000000000, 0.9510565162951535312, 1.000000000000000000, 0.9510565162951535312, 1.000000000000000000, 0.9510565162951535312, 1.000000000000000000, 0.9510565162951535312, 1.000000000000000000, 0.9510565162951535312, 1.000000000000000000, 0.9510565162951535312, 1.000000000000000000, 0.9510565162951535312, 1.000000000000000000, 0.9510565162951535312, 1.000000000000000000, 0.9510565162951535312, 1.000000000000000000, 0.9510565162951535312, 1.000000000000000000, 0.9510565162951535312, 1.000000000000000000, 0.9510565162951535312, 1.000000000000000000, 0.9510565162951535312, 1.000000000000000000, 0.9510565162951535312, 1.000000000000000000, 0.9510565162951535312, 1.000000000000000000, 0.9510565162951535312, 1.000000000000000000, 0.9510565162951535312, 1.000000000000000000, 0.9510565162951535312, 1.000000000000000000, 0.9510565162951535312, 1.000000000000000000, 0.9510565162951535312, 1.000000000000000000, 0.9510565162951535312, 1.000000000000000000, 0.9510565162951535312, 1.000000000000000000, 0.9510565162951535312, 1.000000000000000000, 0.9510565162951535312, 1.000000000000000000, 0.9510565162951535312, 1.000000000000000000, 0.9510565162951535312, 1.000000000000000000, 0.9510565162951535312, 1.000000000000000000, 0.9510565162951535312, 1.000000000000000000, 0.9510565162951535312, 1.000000000000000000, 0.9510565162951535312, 1.000000000000000000, 0.9510565162951535312, 1.000000000000000000, 0.9510565162951535312, 1.000000000000000000, 0.9510565162951535312, 1.000000000000000000, 0.9510565162951535312, 1.000000000000000000, 0.9510565162951535312, 1.000000000000000000, 0.9510565162951535312, 1.000000000000000000, 0.9510565162951535312, 1.000000000000000000, 0.9510565162951535312, 1.000000000000000000, 0.9510565162951535312, 1.000000000000000000, 0.9510565162951535312, 1.000000000000000000, 0.9510565162951535312, 1.000000000000000000, 0.9510565162951535312, 1.000000000000000000, 0.9510565162951535312, 1.000000000000000000, 0.9510565162951535312, 1.000000000000000000, 0.9510565162951535312, 1.000000000000000000, 0.9510565162951535312, 1.000000000000000000, 0.9510565162951535312, 1.000000000000000000, 0.9510565162951535312, 1.000000000000000000, 0.9510565162951535312, 1.000000000000000000, 0.9510565162951535312, 1.000000000000000000, 0.9510565162951535312, 1.000000000000000000, 0.9510565162951535312, 1.000000000000000000, 0.9510565162951535312, 1.000000000000000000, 0.9510565162951535312, 1.000000000000000000, 0.9510565162951535312, 1.000000000000000000, 0.9510565162951535312, 1.000000000000000000, 0.9510565162951535312, 1.000000000000000000, 0.9510565162951535312, 1.000000000000000000, 0.9510565162951535312, 1.000000000000000000, 0.9510565162951535312, 1.000000000000000000, 0.9510565162951535312, 1.000000000000000000, 0.9510565162951535312, 1.000000000000000000, 0.9510565162951535312, 1.000000000000000000, 0.9510565162951535312, 1.000000000000000000, 0.9510565162951535312, 1.000000000000000000, 0.9510565162951535312, 1.000000000000000000, 0.9510565162951535312, 1.000000000000000000, 0.9510565162951535312, 1.000000000000000000, 0.9510565162951535312, 1.000000000000000000, 0.9510565162951535312, 1.000000000000000000, 0.9510565162951535312, 1.000000000000000000, 0.9510565162951535312, 1.000000000000000000, 0.9510565162951535312, 1.000000000000000000, 0.9510565162951535312, 1.000000000000000000, 0.9510565162951535312, 1.000000000000000000, 0.9510565162951535312, 1.000000000000000000, 0.9510565162951535312, 1.000000000000000000, 0.9510565162951535312, 1.000000000000000000, 0.9510565162951535312, 1.000000000000000000, 0.9510565162951535312, 1.000000000000000000, 0.9510565162951535312, 1.000000000000000000, 0.9510565162951535312, 1.000000000000000000, 0.9510565162951535312, 1.000000000000000000, 0.9510565162951535312, 1.000000000000000000, 0.9510565162951535312, 1.000000000000000000, 0.9510565162951535312, 1.000000000000000000, 0.9510565162951535312, 1.000000000000000000, 0.9510565162951535312, 1.000000000000000000, 0.9510565162951535312, 1.000000000000000000, 0.9510565162951535312, 1.000000000000000000, 0.9510565162951535312, 1.000000000000000000, 0.9510565162951535312, 1.000000000000000000, 0.9510565162951535312, 1.000000000000000000),
 ( 0.3333333333333333703, 0.3170188387650512141, 0.3333333333333333703, 0.3170188387650512141, 0.3333333333333333703, 0.3170188387650512141, 0.3333333333333333703, 0.3170188387650512141, 0.3333333333333333703, 0.3170188387650512141, 0.3333333333333333703, 0.3170188387650512141, 0.3333333333333333703, 0.3170188387650512141, 0.3333333333333333703, 0.3170188387650512141, 0.3333333333333333703, 0.3170188387650512141, 0.3333333333333333703, 0.3170188387650512141, 0.3333333333333333703, 0.3170188387650512141, 0.3333333333333333703, 0.3170188387650512141, 0.3333333333333333703, 0.3170188387650512141, 0.3333333333333333703, 0.3170188387650512141, 0.3333333333333333703, 0.3170188387650512141, 0.3333333333333333703, 0.3170188387650512141, 0.3333333333333333703, 0.3170188387650512141, 0.3333333333333333703, 0.3170188387650512141, 0.3333333333333333703, 0.3170188387650512141, 0.3333333333333333703, 0.3170188387650512141, 0.3333333333333333703, 0.3170188387650512141, 0.3333333333333333703, 0.3170188387650512141, 0.3333333333333333703, 0.3170188387650512141, 0.3333333333333333703, 0.3170188387650512141, 0.3333333333333333703, 0.3170188387650512141, 0.3333333333333333703, 0.3170188387650512141, 0.3333333333333333703, 0.3170188387650512141, 0.3333333333333333703, 0.3170188387650512141, 0.3333333333333333703, 0.3170188387650512141, 0.3333333333333333703, 0.3170188387650512141, 0.3333333333333333703, 0.3170188387650512141, 0.3333333333333333703, 0.3170188387650512141, 0.3333333333333333703, 0.3170188387650512141, 0.3333333333333333703, 0.3170188387650512141, 0.3333333333333333703, 0.3170188387650512141, 0.3333333333333333703, 0.3170188387650512141, 0.3333333333333333703, 0.3170188387650512141, 0.3333333333333333703, 0.3170188387650512141, 0.3333333333333333703, 0.3170188387650512141, 0.3333333333333333703, 0.3170188387650512141, 0.3333333333333333703, 0.3170188387650512141, 0.3333333333333333703, 0.3170188387650512141, 0.3333333333333333703, 0.3170188387650512141, 0.3333333333333333703, 0.3170188387650512141, 0.3333333333333333703, 0.3170188387650512141, 0.3333333333333333703, 0.3170188387650512141, 0.3333333333333333703, 0.3170188387650512141, 0.3333333333333333703, 0.3170188387650512141, 0.3333333333333333703, 0.3170188387650512141, 0.3333333333333333703, 0.3170188387650512141, 0.3333333333333333703, 0.3170188387650512141, 0.3333333333333333703, 0.3170188387650512141, 0.3333333333333333703, 0.3170188387650512141, 0.3333333333333333703, 0.3170188387650512141, 0.3333333333333333703, 0.3170188387650512141, 0.3333333333333333703, 0.3170188387650512141, 0.3333333333333333703, 0.3170188387650512141, 0.3333333333333333703, 0.3170188387650512141, 0.3333333333333333703, 0.3170188387650512141, 0.3333333333333333703, 0.3170188387650512141, 0.3333333333333333703, 0.3170188387650512141, 0.3333333333333333703, 0.3170188387650512141, 0.3333333333333333703, 0.3170188387650512141, 0.3333333333333333703, 0.3170188387650512141, 0.3333333333333333703, 0.3170188387650512141, 0.3333333333333333703, 0.3170188387650512141, 0.3333333333333333703, 0.3170188387650512141, 0.3333333333333333703, 0.3170188387650512141, 0.3333333333333333703, 0.3170188387650512141, 0.3333333333333333703, 0.3170188387650512141, 0.3333333333333333703, 0.3170188387650512141, 0.3333333333333333703, 0.3170188387650512141, 0.3333333333333333703, 0.3170188387650512141, 0.3333333333333333703, 0.3170188387650512141, 0.3333333333333333703, 0.3170188387650512141, 0.3333333333333333703, 0.3170188387650512141, 0.3333333333333333703, 0.3170188387650512141, 0.3333333333333333703, 0.3170188387650512141, 0.3333333333333333703, 0.3170188387650512141, 0.3333333333333333703, 0.3170188387650512141, 0.3333333333333333703, 0.3170188387650512141, 0.3333333333333333703, 0.3170188387650512141, 0.3333333333333333703, 0.3170188387650512141, 0.3333333333333333703, 0.3170188387650512141, 0.3333333333333333703, 0.3170188387650512141, 0.3333333333333333703, 0.3170188387650512141, 0.3333333333333333703, 0.3170188387650512141, 0.3333333333333333703, 0.3170188387650512141, 0.3333333333333333703, 0.3170188387650512141, 0.3333333333333333703, 0.3170188387650512141, 0.3333333333333333703, 0.3170188387650512141, 0.3333333333333333703, 0.3170188387650512141, 0.3333333333333333703, 0.3170188387650512141, 0.3333333333333333703, 0.3170188387650512141, 0.3333333333333333703, 0.3170188387650512141, 0.3333333333333333703, 0.3170188387650512141, 0.3333333333333333703, 0.3170188387650512141, 0.3333333333333333703, 0.3170188387650512141, 0.3333333333333333703, 0.3170188387650512141, 0.3333333333333333703, 0.3170188387650512141, 0.3333333333333333703),
 ( 0.3333333333333333703, 0.3170188387650512141, 0.3333333333333333703, 0.3170188387650512141, 0.3333333333333333703, 0.3170188387650512141, 0.3333333333333333703, 0.3170188387650512141, 0.3333333333333333703, 0.3170188387650512141, 0.3333333333333333703, 0.3170188387650512141, 0.3333333333333333703, 0.3170188387650512141, 0.3333333333333333703, 0.3170188387650512141, 0.3333333333333333703, 0.3170188387650512141, 0.3333333333333333703, 0.3170188387650512141, 0.3333333333333333703, 0.3170188387650512141, 0.3333333333333333703, 0.3170188387650512141, 0.3333333333333333703, 0.3170188387650512141, 0.3333333333333333703, 0.3170188387650512141, 0.3333333333333333703, 0.3170188387650512141, 0.3333333333333333703, 0.3170188387650512141, 0.3333333333333333703, 0.3170188387650512141, 0.3333333333333333703, 0.3170188387650512141, 0.3333333333333333703, 0.3170188387650512141, 0.3333333333333333703, 0.3170188387650512141, 0.3333333333333333703, 0.3170188387650512141, 0.3333333333333333703, 0.3170188387650512141, 0.3333333333333333703, 0.3170188387650512141, 0.3333333333333333703, 0.3170188387650512141, 0.3333333333333333703, 0.3170188387650512141, 0.3333333333333333703, 0.3170188387650512141, 0.3333333333333333703, 0.3170188387650512141, 0.3333333333333333703, 0.3170188387650512141, 0.3333333333333333703, 0.3170188387650512141, 0.3333333333333333703, 0.3170188387650512141, 0.3333333333333333703, 0.3170188387650512141, 0.3333333333333333703, 0.3170188387650512141, 0.3333333333333333703, 0.3170188387650512141, 0.3333333333333333703, 0.3170188387650512141, 0.3333333333333333703, 0.3170188387650512141, 0.3333333333333333703, 0.3170188387650512141, 0.3333333333333333703, 0.3170188387650512141, 0.3333333333333333703, 0.3170188387650512141, 0.3333333333333333703, 0.3170188387650512141, 0.3333333333333333703, 0.3170188387650512141, 0.3333333333333333703, 0.3170188387650512141, 0.3333333333333333703, 0.3170188387650512141, 0.3333333333333333703, 0.3170188387650512141, 0.3333333333333333703, 0.3170188387650512141, 0.3333333333333333703, 0.3170188387650512141, 0.3333333333333333703, 0.3170188387650512141, 0.3333333333333333703, 0.3170188387650512141, 0.3333333333333333703, 0.3170188387650512141, 0.3333333333333333703, 0.3170188387650512141, 0.3333333333333333703, 0.3170188387650512141, 0.3333333333333333703, 0.3170188387650512141, 0.3333333333333333703, 0.3170188387650512141, 0.3333333333333333703, 0.3170188387650512141, 0.3333333333333333703, 0.3170188387650512141, 0.3333333333333333703, 0.3170188387650512141, 0.3333333333333333703, 0.3170188387650512141, 0.3333333333333333703, 0.3170188387650512141, 0.3333333333333333703, 0.3170188387650512141, 0.3333333333333333703, 0.3170188387650512141, 0.3333333333333333703, 0.3170188387650512141, 0.3333333333333333703, 0.3170188387650512141, 0.3333333333333333703, 0.3170188387650512141, 0.3333333333333333703, 0.3170188387650512141, 0.3333333333333333703, 0.3170188387650512141, 0.3333333333333333703, 0.3170188387650512141, 0.3333333333333333703, 0.3170188387650512141, 0.3333333333333333703, 0.3170188387650512141, 0.3333333333333333703, 0.3170188387650512141, 0.3333333333333333703, 0.3170188387650512141, 0.3333333333333333703, 0.3170188387650512141, 0.3333333333333333703, 0.3170188387650512141, 0.3333333333333333703, 0.3170188387650512141, 0.3333333333333333703, 0.3170188387650512141, 0.3333333333333333703, 0.3170188387650512141, 0.3333333333333333703, 0.3170188387650512141, 0.3333333333333333703, 0.3170188387650512141, 0.3333333333333333703, 0.3170188387650512141, 0.3333333333333333703, 0.3170188387650512141, 0.3333333333333333703, 0.3170188387650512141, 0.3333333333333333703, 0.3170188387650512141, 0.3333333333333333703, 0.3170188387650512141, 0.3333333333333333703, 0.3170188387650512141, 0.3333333333333333703, 0.3170188387650512141, 0.3333333333333333703, 0.3170188387650512141, 0.3333333333333333703, 0.3170188387650512141, 0.3333333333333333703, 0.3170188387650512141, 0.3333333333333333703, 0.3170188387650512141, 0.3333333333333333703, 0.3170188387650512141, 0.3333333333333333703, 0.3170188387650512141, 0.3333333333333333703, 0.3170188387650512141, 0.3333333333333333703, 0.3170188387650512141, 0.3333333333333333703, 0.3170188387650512141, 0.3333333333333333703, 0.3170188387650512141, 0.3333333333333333703, 0.3170188387650512141, 0.3333333333333333703, 0.3170188387650512141, 0.3333333333333333703, 0.3170188387650512141, 0.3333333333333333703, 0.3170188387650512141, 0.3333333333333333703, 0.3170188387650512141, 0.3333333333333333703, 0.3170188387650512141, 0.3333333333333333703, 0.3170188387650512141, 0.3333333333333333703),
 ( 1.000000000000000000, 0.9510565162951535312, 1.000000000000000000, 0.9510565162951535312, 1.000000000000000000, 0.9510565162951535312, 1.000000000000000000, 0.9510565162951535312, 1.000000000000000000, 0.9510565162951535312, 1.000000000000000000, 0.9510565162951535312, 1.000000000000000000, 0.9510565162951535312, 1.000000000000000000, 0.9510565162951535312, 1.000000000000000000, 0.9510565162951535312, 1.000000000000000000, 0.9510565162951535312, 1.000000000000000000, 0.9510565162951535312, 1.000000000000000000, 0.9510565162951535312, 1.000000000000000000, 0.9510565162951535312, 1.000000000000000000, 0.9510565162951535312, 1.000000000000000000, 0.9510565162951535312, 1.000000000000000000, 0.9510565162951535312, 1.000000000000000000, 0.9510565162951535312, 1.000000000000000000, 0.9510565162951535312, 1.000000000000000000, 0.9510565162951535312, 1.000000000000000000, 0.9510565162951535312, 1.000000000000000000, 0.9510565162951535312, 1.000000000000000000, 0.9510565162951535312, 1.000000000000000000, 0.9510565162951535312, 1.000000000000000000, 0.9510565162951535312, 1.000000000000000000, 0.9510565162951535312, 1.000000000000000000, 0.9510565162951535312, 1.000000000000000000, 0.9510565162951535312, 1.000000000000000000, 0.9510565162951535312, 1.000000000000000000, 0.9510565162951535312, 1.000000000000000000, 0.9510565162951535312, 1.000000000000000000, 0.9510565162951535312, 1.000000000000000000, 0.9510565162951535312, 1.000000000000000000, 0.9510565162951535312, 1.000000000000000000, 0.9510565162951535312, 1.000000000000000000, 0.9510565162951535312, 1.000000000000000000, 0.9510565162951535312, 1.000000000000000000, 0.9510565162951535312, 1.000000000000000000, 0.9510565162951535312, 1.000000000000000000, 0.9510565162951535312, 1.000000000000000000, 0.9510565162951535312, 1.000000000000000000, 0.9510565162951535312, 1.000000000000000000, 0.9510565162951535312, 1.000000000000000000, 0.9510565162951535312, 1.000000000000000000, 0.9510565162951535312, 1.000000000000000000, 0.9510565162951535312, 1.000000000000000000, 0.9510565162951535312, 1.000000000000000000, 0.9510565162951535312, 1.000000000000000000, 0.9510565162951535312, 1.000000000000000000, 0.9510565162951535312, 1.000000000000000000, 0.9510565162951535312, 1.000000000000000000, 0.9510565162951535312, 1.000000000000000000, 0.9510565162951535312, 1.000000000000000000, 0.9510565162951535312, 1.000000000000000000, 0.9510565162951535312, 1.000000000000000000, 0.9510565162951535312, 1.000000000000000000, 0.9510565162951535312, 1.000000000000000000, 0.9510565162951535312, 1.000000000000000000, 0.9510565162951535312, 1.000000000000000000, 0.9510565162951535312, 1.000000000000000000, 0.9510565162951535312, 1.000000000000000000, 0.9510565162951535312, 1.000000000000000000, 0.9510565162951535312, 1.000000000000000000, 0.9510565162951535312, 1.000000000000000000, 0.9510565162951535312, 1.000000000000000000, 0.9510565162951535312, 1.000000000000000000, 0.9510565162951535312, 1.000000000000000000, 0.9510565162951535312, 1.000000000000000000, 0.9510565162951535312, 1.000000000000000000, 0.9510565162951535312, 1.000000000000000000, 0.9510565162951535312, 1.000000000000000000, 0.9510565162951535312, 1.000000000000000000, 0.9510565162951535312, 1.000000000000000000, 0.9510565162951535312, 1.000000000000000000, 0.9510565162951535312, 1.000000000000000000, 0.9510565162951535312, 1.000000000000000000, 0.9510565162951535312, 1.000000000000000000, 0.9510565162951535312, 1.000000000000000000, 0.9510565162951535312, 1.000000000000000000, 0.9510565162951535312, 1.000000000000000000, 0.9510565162951535312, 1.000000000000000000, 0.9510565162951535312, 1.000000000000000000, 0.9510565162951535312, 1.000000000000000000, 0.9510565162951535312, 1.000000000000000000, 0.9510565162951535312, 1.000000000000000000, 0.9510565162951535312, 1.000000000000000000, 0.9510565162951535312, 1.000000000000000000, 0.9510565162951535312, 1.000000000000000000, 0.9510565162951535312, 1.000000000000000000, 0.9510565162951535312, 1.000000000000000000, 0.9510565162951535312, 1.000000000000000000, 0.9510565162951535312, 1.000000000000000000, 0.9510565162951535312, 1.000000000000000000, 0.9510565162951535312, 1.000000000000000000, 0.9510565162951535312, 1.000000000000000000, 0.9510565162951535312, 1.000000000000000000, 0.9510565162951535312, 1.000000000000000000, 0.9510565162951535312, 1.000000000000000000, 0.9510565162951535312, 1.000000000000000000, 0.9510565162951535312, 1.000000000000000000, 0.9510565162951535312, 1.000000000000000000) ) ) 
 REPRESENTATION_ITEM ( '' )  SURFACE ( )  );
#14561=CARTESIAN_POINT ( 'NONE',  ( 57.36023556966787851, 55.99948385550239038, -0.02388180880522424582 ) ) ;
#14572=CARTESIAN_POINT ( 'NONE',  ( 54.09612160359786515, 51.69948385550240744, -5.676469297603166098 ) ) ;
#14575=CARTESIAN_POINT ( 'NONE',  ( 43.34962307344078880, 50.10051614449766078, -2.184720259617096705 ) ) ;
#14595=CARTESIAN_POINT ( 'NONE',  ( 48.02776887271750184, 49.60051614449766788, 5.992620115222795363 ) ) ;
#14599=CARTESIAN_POINT ( 'NONE',  ( 55.71335778527780747, 54.09948385550241312, 1.832500667257165983 ) ) ;
#14601=CARTESIAN_POINT ( 'NONE',  ( 56.81924384183011512, 64.19948385550240744, 4.924951120819313743 ) ) ;
#14602=CARTESIAN_POINT ( 'NONE',  ( 42.38452918213190657, 47.90051614449765793, 2.450534656007115508 ) ) ;
#14619=CARTESIAN_POINT ( 'NONE',  ( 43.34962307344081012, 54.89948385550240317, 2.184720259617164650 ) ) ;
#14621=CARTESIAN_POINT ( 'NONE',  ( 54.68390685589033495, 49.69948385550240744, -6.485486291978119766 ) ) ;
#14622=CARTESIAN_POINT ( 'NONE',  ( 49.97728705011495265, 45.50051614449765935, 7.000000000000000888 ) ) ;
#14638=CARTESIAN_POINT ( 'NONE',  ( 41.58830220609386430, 56.99948385550241170, 0.02388180880523263147 ) ) ;
#14642=CARTESIAN_POINT ( 'NONE',  ( 55.69932041026404335, 49.89948385550241028, -1.875703265242203432 ) ) ;
#14645=CARTESIAN_POINT ( 'NONE',  ( 47.37792948025170858, 49.60051614449766788, 7.992620115222797139 ) ) ;
#14647=CARTESIAN_POINT ( 'NONE',  ( 53.54508667620424234, 46.70051614449766220, -4.840751629271188961 ) ) ;
#14665=CARTESIAN_POINT ( 'NONE',  ( 47.74827507625477807, 46.59948385550239180, 7.007379884777229506 ) ) ;
#14671=CARTESIAN_POINT ( 'NONE',  ( 55.96859303347804371, 50.19948385550240744, 4.306917132069425946 ) ) ;
#14673=CARTESIAN_POINT ( 'NONE',  ( 49.97728705011495265, 49.50051614449765935, 7.000000000000000888 ) ) ;
#14689=CARTESIAN_POINT ( 'NONE',  ( 54.89903213687075834, 44.74560054925188268, -5.000000000000007105 ) ) ;
#14695=CARTESIAN_POINT ( 'NONE',  ( 43.69122665457040000, 50.00051614449765935, -0.02388180880515696977 ) ) ;
#14698=CARTESIAN_POINT ( 'NONE',  ( 44.91013252490152752, 48.79948385550240175, 3.727524721679198461 ) ) ;
#14700=CARTESIAN_POINT ( 'NONE',  ( 50.02271294988512551, 50.49948385550240459, 7.000000000000000888 ) ) ;
#14702=CARTESIAN_POINT ( 'NONE',  ( 45.27934281921082516, 45.70051614449766220, 6.458785618021089192 ) ) ;
#14721=DIRECTION ( 'NONE',  ( -0.04542589977017699732, 0.9989677110047501252, 0.000000000000000000 ) ) ;
#14722=CARTESIAN_POINT ( 'NONE',  ( 45.86712807150323812, 49.29948385550240175, -5.649768623646098220 ) ) ;
#14725=CARTESIAN_POINT ( 'NONE',  ( 57.60143344285433642, 53.89948385550240317, -2.493737253992118319 ) ) ;
#14727=CARTESIAN_POINT ( 'NONE',  ( 47.70284917648459100, 47.60051614449763946, 6.992620115222796251 ) ) ;
#14742=CARTESIAN_POINT ( 'NONE',  ( 57.60143344285433642, 57.89948385550241028, -2.493737253992118319 ) ) ;
#14744=CARTESIAN_POINT ( 'NONE',  ( 46.49166364869460466, 58.69948385550240033, 4.867452303228209765 ) ) ;
#14749=CARTESIAN_POINT ( 'NONE',  ( 41.58830220609386430, 46.00051614449764514, -0.02388180880514929535 ) ) ;
#14750=CARTESIAN_POINT ( 'NONE',  ( 44.30067958973594955, 50.10051614449766078, -1.875703265242155693 ) ) ;
#14763=CARTESIAN_POINT ( 'NONE',  ( 55.94051828345050836, 47.79948385550240886, -4.345558710429103577 ) ) ;
#14769=CARTESIAN_POINT ( 'NONE',  ( 54.09612160359786515, 53.69948385550240744, -5.676469297603166098 ) ) ;
#14772=CARTESIAN_POINT ( 'NONE',  ( 55.94051828345053679, 49.20051614449766930, 4.345558710429044069 ) ) ;
#14785=CARTESIAN_POINT ( 'NONE',  ( 56.66441430157296821, 48.09948385550240602, 2.141517661632100111 ) ) ;
#14796=CARTESIAN_POINT ( 'NONE',  ( 53.54508667620424234, 48.70051614449766930, -4.840751629271188961 ) ) ;
#14799=CARTESIAN_POINT ( 'NONE',  ( 46.49166364869460466, 60.69948385550240033, 4.867452303228209765 ) ) ;
#14801=CARTESIAN_POINT ( 'NONE',  ( 52.25172492374522903, 55.59948385550241312, -7.007379884777225953 ) ) ;
#14803=CARTESIAN_POINT ( 'NONE',  ( 47.42335538002180328, 52.40051614449767214, -8.007379884777206414 ) ) ;
#14811=PRODUCT_DEFINITION_FORMATION_WITH_SPECIFIED_SOURCE ( 'ANY', '', #3649, .NOT_KNOWN. ) ;
#14821=CARTESIAN_POINT ( 'NONE',  ( 43.34962307344081012, 56.89948385550240317, 2.184720259617164650 ) ) ;
#14823=CARTESIAN_POINT ( 'NONE',  ( 58.41169779390614281, 55.99948385550241170, -0.02388180880523160798 ) ) ;
#14826=CARTESIAN_POINT ( 'NONE',  ( 56.66441430157294690, 48.90051614449766504, -2.141517661632166281 ) ) ;
#14845=CARTESIAN_POINT ( 'NONE',  ( 56.30877334542961421, 53.99948385550241170, -0.02388180880520959434 ) ) ;
#14849=CARTESIAN_POINT ( 'NONE',  ( 54.68390685589039890, 53.30051614449767072, 6.485486291978072693 ) ) ;
#14852=CARTESIAN_POINT ( 'NONE',  ( 53.50833635130544508, 47.30051614449766362, 4.867452303228181343 ) ) ;
#14863=CARTESIAN_POINT ( 'NONE',  ( 45.86712807150323812, 47.29948385550240886, -5.649768623646098220 ) ) ;
#14869=CARTESIAN_POINT ( 'NONE',  ( 55.94051828345050836, 59.79948385550238754, -4.345558710429104465 ) ) ;
#14871=CARTESIAN_POINT ( 'NONE',  ( 44.05948171654945611, 54.20051614449764799, -4.345558710429044069 ) ) ;
#14882=CARTESIAN_POINT ( 'NONE',  ( 52.57664461997811856, 63.59948385550239891, -8.007379884777229506 ) ) ;
#14887=CARTESIAN_POINT ( 'NONE',  ( 56.65037692655921120, 61.10051614449766078, 2.184720259617097593 ) ) ;
#14894=CARTESIAN_POINT ( 'NONE',  ( 44.91013252490150620, 46.20051614449766220, -3.727524721679154940 ) ) ;
#14899=CARTESIAN_POINT ( 'NONE',  ( 43.69122665457040000, 58.99948385550239749, 0.02388180880521036456 ) ) ;
#14901=CARTESIAN_POINT ( 'NONE',  ( 42.63976443033212860, 50.99948385550240459, 0.02388180880522514787 ) ) ;
#14902=CARTESIAN_POINT ( 'NONE',  ( 52.57664461997821093, 53.40051614449765793, 8.007379884777206414 ) ) ;
#14916=CARTESIAN_POINT ( 'NONE',  ( 43.34962307344081012, 62.89948385550241028, 2.184720259617164650 ) ) ;
#14921=CARTESIAN_POINT ( 'NONE',  ( 47.70284917648453415, 59.39948385550241028, -6.992620115222774047 ) ) ;
#14924=CARTESIAN_POINT ( 'NONE',  ( 54.72065718078924590, 52.29948385550240886, 6.458785618021043895 ) ) ;
#14926=CARTESIAN_POINT ( 'NONE',  ( 43.33558569842706021, 57.90051614449766504, 2.141517661632167169 ) ) ;
#14941=CARTESIAN_POINT ( 'NONE',  ( 48.07319477248768180, 56.59948385550239891, 6.007379884777225953 ) ) ;
#14944=CARTESIAN_POINT ( 'NONE',  ( 43.20883090819742023, 56.20051614449766220, -4.963592699178938972 ) ) ;
#14945=CARTESIAN_POINT ( 'NONE',  ( 46.49166364869456913, 58.30051614449765651, -4.867452303228181343 ) ) ;
#14955=CARTESIAN_POINT ( 'NONE',  ( 52.25172492374522903, 63.59948385550237759, -7.007379884777225953 ) ) ;
#14961=CARTESIAN_POINT ( 'NONE',  ( 49.97728705011488159, 47.49948385550240459, -7.000000000000000888 ) ) ;
#14965=CARTESIAN_POINT ( 'NONE',  ( 45.31609314410967926, 48.69948385550241454, 6.485486291978119766 ) ) ;
#14967=CARTESIAN_POINT ( 'NONE',  ( 47.74827507625478518, 58.59948385550238470, 7.007379884777227730 ) ) ;
#14969=CARTESIAN_POINT ( 'NONE',  ( 44.03140696652198471, 51.80051614449766362, 4.306917132069485454 ) ) ;
#14980=CARTESIAN_POINT ( 'NONE',  ( 44.05948171654949874, 46.79948385550238754, 4.345558710429105354 ) ) ;
#14986=CARTESIAN_POINT ( 'NONE',  ( 43.34962307344078880, 58.10051614449766078, -2.184720259617096705 ) ) ;
#14993=CARTESIAN_POINT ( 'NONE',  ( 55.08986747509849380, 55.20051614449766220, 3.727524721679155384 ) ) ;
#14996=CARTESIAN_POINT ( 'NONE',  ( 46.45491332379572924, 55.29948385550240175, -4.840751629271157874 ) ) ;
#14999=CARTESIAN_POINT ( 'NONE',  ( 52.62207051974829852, 52.60051614449765367, -7.992620115222797139 ) ) ;
#15019=CARTESIAN_POINT ( 'NONE',  ( 55.96859303347804371, 58.19948385550241454, 4.306917132069425946 ) ) ;
#15022=CARTESIAN_POINT ( 'NONE',  ( 42.38452918213188525, 53.09948385550240602, -2.450534656007040013 ) ) ;
#15024=CARTESIAN_POINT ( 'NONE',  ( 45.86712807150329496, 53.70051614449766220, 5.649768623646139964 ) ) ;
#15037=CARTESIAN_POINT ( 'NONE',  ( 55.94051828345050836, 61.79948385550239465, -4.345558710429104465 ) ) ;
#15039=DIRECTION ( 'NONE',  ( -0.9989677110047504582, -0.04542589977017007230, 1.386346192018204258E-14 ) ) ;
#15043=CARTESIAN_POINT ( 'NONE',  ( 44.88205777487398507, 57.19948385550241454, -3.688883143319540814 ) ) ;
#15047=CARTESIAN_POINT ( 'NONE',  ( 56.81924384183006538, 52.80051614449766362, -4.924951120819380357 ) ) ;
#15049=CARTESIAN_POINT ( 'NONE',  ( 44.28664221472221385, 55.90051614449766504, 1.832500667257213722 ) ) ;
#15060=CARTESIAN_POINT ( 'NONE',  ( 47.74827507625478518, 62.59948385550240602, 7.007379884777227730 ) ) ;
#15065=CARTESIAN_POINT ( 'NONE',  ( 43.33558569842703179, 49.09948385550240602, -2.141517661632099223 ) ) ;
#15069=ORIENTED_EDGE ( 'NONE', *, *, #17915, .F. ) ;
#15070=CARTESIAN_POINT ( 'NONE',  ( 57.61547081786812896, 48.09948385550240602, 2.450534656007040901 ) ) ;
#15073=CARTESIAN_POINT ( 'NONE',  ( 54.09612160359786515, 55.69948385550240744, -5.676469297603166098 ) ) ;
#15076=CARTESIAN_POINT ( 'NONE',  ( 54.13287192849671214, 54.70051614449766220, -5.649768623646139964 ) ) ;
#15086=CARTESIAN_POINT ( 'NONE',  ( 58.41169779390614281, 63.99948385550241170, -0.02388180880523160798 ) ) ;
#15093=CARTESIAN_POINT ( 'NONE',  ( 52.29715082351539479, 60.60051614449764656, -6.992620115222796251 ) ) ;
#15098=CARTESIAN_POINT ( 'NONE',  ( 49.97728705011494554, 55.50051614449766646, 6.000000000000000888 ) ) ;
#15102=CARTESIAN_POINT ( 'NONE',  ( 48.07319477248768180, 58.59948385550239891, 6.007379884777225953 ) ) ;
#15104=CARTESIAN_POINT ( 'NONE',  ( 41.58830220609386430, 54.00051614449765935, -0.02388180880514929535 ) ) ;
#15118=CARTESIAN_POINT ( 'NONE',  ( 43.33558569842703179, 59.09948385550240602, -2.141517661632099223 ) ) ;
#15120=CARTESIAN_POINT ( 'NONE',  ( 47.37792948025162332, 51.39948385550241028, -7.992620115222770494 ) ) ;
#15122=CARTESIAN_POINT ( 'NONE',  ( 44.05948171654945611, 52.20051614449764799, -4.345558710429044069 ) ) ;
#15129=CARTESIAN_POINT ( 'NONE',  ( 44.03140696652192787, 65.19948385550240744, -4.306917132069425058 ) ) ;
#15135=CARTESIAN_POINT ( 'NONE',  ( 44.30067958973596376, 54.89948385550240317, 1.875703265242204099 ) ) ;
#15138=CARTESIAN_POINT ( 'NONE',  ( 52.62207051974829852, 54.60051614449766788, -7.992620115222797139 ) ) ;
#15139=CARTESIAN_POINT ( 'NONE',  ( 50.02271294988506156, 54.50051614449765935, -6.000000000000000888 ) ) ;
#15154=CARTESIAN_POINT ( 'NONE',  ( 52.29715082351547295, 50.39948385550241028, 6.992620115222774047 ) ) ;
#15159=CARTESIAN_POINT ( 'NONE',  ( 57.61547081786812896, 46.09948385550240602, 2.450534656007040901 ) ) ;
#15163=CARTESIAN_POINT ( 'NONE',  ( 47.70284917648453415, 57.39948385550241028, -6.992620115222774047 ) ) ;
#15167=CARTESIAN_POINT ( 'NONE',  ( 52.29715082351538769, 56.60051614449766788, -6.992620115222796251 ) ) ;
#15175=CARTESIAN_POINT ( 'NONE',  ( 42.39856655714566358, 64.89948385550239607, 2.493737253992119207 ) ) ;
#15180=CARTESIAN_POINT ( 'NONE',  ( 45.90387839640208512, 60.30051614449766362, -5.676469297603124353 ) ) ;
#15187=CARTESIAN_POINT ( 'NONE',  ( 53.50833635130544508, 57.30051614449767072, 4.867452303228181343 ) ) ;
#15191=CARTESIAN_POINT ( 'NONE',  ( 55.71335778527780747, 60.09948385550240602, 1.832500667257165983 ) ) ;
#15193=CARTESIAN_POINT ( 'NONE',  ( 47.42335538002180328, 54.40051614449765793, -8.007379884777206414 ) ) ;
#15207=CARTESIAN_POINT ( 'NONE',  ( 45.90387839640214196, 64.69948385550240744, 5.676469297603166098 ) ) ;
#15212=CARTESIAN_POINT ( 'NONE',  ( 54.09612160359786515, 59.69948385550240033, -5.676469297603166098 ) ) ;
#15214=CARTESIAN_POINT ( 'NONE',  ( 43.20883090819745576, 60.79948385550241596, 4.963592699179006473 ) ) ;
#15215=CARTESIAN_POINT ( 'NONE',  ( 44.05948171654945611, 56.20051614449764799, -4.345558710429044069 ) ) ;
#15217=CARTESIAN_POINT ( 'NONE',  ( 49.99999999999997158, 45.00000000000001421, -7.000000000000000888 ) ) ;
#15222=CARTESIAN_POINT ( 'NONE',  ( 54.09612160359792199, 45.30051614449766362, 5.676469297603124353 ) ) ;
#15229=CARTESIAN_POINT ( 'NONE',  ( 44.88205777487398507, 65.19948385550240744, -3.688883143319540814 ) ) ;
#15232=CARTESIAN_POINT ( 'NONE',  ( 42.39856655714564226, 52.10051614449766788, -2.493737253992044156 ) ) ;
#15233=CARTESIAN_POINT ( 'NONE',  ( 50.02271294988506156, 52.50051614449766646, -6.000000000000000888 ) ) ;
#15246=CARTESIAN_POINT ( 'NONE',  ( 54.09612160359786515, 53.69948385550240744, -5.676469297603166098 ) ) ;
#15250=CARTESIAN_POINT ( 'NONE',  ( 57.60143344285435774, 63.10051614449766078, 2.493737253992045044 ) ) ;
#15253=CARTESIAN_POINT ( 'NONE',  ( 48.07319477248768180, 46.59948385550239891, 6.007379884777225953 ) ) ;
#15257=CARTESIAN_POINT ( 'NONE',  ( 43.34962307344078880, 52.10051614449766078, -2.184720259617096705 ) ) ;
#15261=CARTESIAN_POINT ( 'NONE',  ( 44.03140696652192787, 53.19948385550238612, -4.306917132069425058 ) ) ;
#15269=CARTESIAN_POINT ( 'NONE',  ( 44.03140696652192787, 55.19948385550238612, -4.306917132069425058 ) ) ;
#15276=CARTESIAN_POINT ( 'NONE',  ( 47.74827507625470702, 58.40051614449766504, -7.007379884777204637 ) ) ;
#15283=CARTESIAN_POINT ( 'NONE',  ( 53.54508667620424234, 52.70051614449766220, -4.840751629271188961 ) ) ;
#15287=CARTESIAN_POINT ( 'NONE',  ( 48.02776887271750184, 45.60051614449765367, 5.992620115222795363 ) ) ;
#15289=CARTESIAN_POINT ( 'NONE',  ( 45.27934281921082516, 57.70051614449766930, 6.458785618021089192 ) ) ;
#15290=STYLED_ITEM ( 'NONE', ( #12732 ), #780 ) ;
#15303=CARTESIAN_POINT ( 'NONE',  ( 47.74827507625477807, 62.59948385550239891, 7.007379884777229506 ) ) ;
#15307=CARTESIAN_POINT ( 'NONE',  ( 51.92680522751233951, 47.59948385550239891, -6.007379884777223289 ) ) ;
#15309=CARTESIAN_POINT ( 'NONE',  ( 58.41169779390614281, 61.99948385550241170, -0.02388180880523160798 ) ) ;
#15310=CARTESIAN_POINT ( 'NONE',  ( 52.25172492374527877, 57.40051614449765083, 7.007379884777203749 ) ) ;
#15313=( BOUNDED_CURVE ( )  B_SPLINE_CURVE ( 2, ( #15511, #3555, #6391, #6483, #13843, #1995, #15222, #17093, #6310, #9232, #3269, #425, #7870, #9522, #16903, #12282, #12369, #1901, #18378, #6586, #18474, #18282, #4835, #1803, #3467, #5024, #14024, #10798, #4925, #9430, #15321, #15414, #16801, #609, #7674, #12570, #7958, #18578, #13928, #7772, #5116, #9330, #13655, #229, #6208, #10710, #12180, #18193, #4751, #16707, #13747, #18867, #12952, #8246, #11183, #8341, #13054, #3747, #12763, #5308, #7071, #14516, #17292, #19064, #5208, #14127, #14322, #15906, #1100, #4411, #15608, #18961, #9809, #5605, #902, #6974, #6779, #5502, #8445, #12665, #16010, #11575, #6872, #11475, #2188, #17485, #18668, #18763, #11283, #17188, #8152, #712, #17591, #17385, #4044, #6683, #2491, #2390, #1009, #14221, #9714, #10007, #15713, #2596, #2293, #806, #3849, #15808, #12862, #5405, #11378, #3946, #9906, #14428, #8546, #4705, #10378, #17952, #10667, #9003, #7632, #7726, #11949, #9287, #3142, #13708, #16672, #16380, #12045, #10469, #3039, #3236, #2945, #7822, #14986, #190, #16568, #15276, #3327, #4799, #18143, #1570, #1856, #18045, #13803, #1, #8907, #9106, #9195, #387, #18338, #13612, #283, #12331, #6354, #6166, #15180, #1760, #12239, #15093, #5982, #10762, #12138, #6259, #14887, #1463, #16759, #7443, #7539, #13421, #4512, #16473, #13524, #97, #6077, #4603, #10564, #18245, #1668, #7915, #15374, #12525, #9668, #3707, #18535, #2048, #5268, #3608, #4977, #12718, #14276, #8298, #5078, #472, #672, #14083, #9382, #18721, #6642 ),
 .UNSPECIFIED., .F., .F. ) 
 B_SPLINE_CURVE_WITH_KNOTS ( ( 3, 2, 2, 2, 2, 2, 2, 2, 2, 2, 2, 2, 2, 2, 2, 2, 2, 2, 2, 2, 2, 2, 2, 2, 2, 2, 2, 2, 2, 2, 2, 2, 2, 2, 2, 2, 2, 2, 2, 2, 2, 2, 2, 2, 2, 2, 2, 2, 2, 2, 2, 2, 2, 2, 2, 2, 2, 2, 2, 2, 2, 2, 2, 2, 2, 2, 2, 2, 2, 2, 2, 2, 2, 2, 2, 2, 2, 2, 2, 2, 2, 2, 2, 2, 2, 2, 2, 2, 2, 2, 2, 2, 2, 2, 2, 2, 2, 2, 2, 3 ),
 ( 0.01230184727895902198, 0.02000000000000000042, 0.02999999999999999889, 0.04000000000000000083, 0.05000000000000000278, 0.05999999999999999778, 0.07000000000000000666, 0.08000000000000000167, 0.08999999999999999667, 0.1000000000000000056, 0.1100000000000000006, 0.1199999999999999956, 0.1300000000000000044, 0.1400000000000000133, 0.1499999999999999944, 0.1600000000000000033, 0.1700000000000000122, 0.1799999999999999933, 0.1900000000000000022, 0.2000000000000000111, 0.2099999999999999922, 0.2200000000000000011, 0.2300000000000000100, 0.2399999999999999911, 0.2500000000000000000, 0.2600000000000000089, 0.2700000000000000178, 0.2800000000000000266, 0.2899999999999999800, 0.2999999999999999889, 0.3099999999999999978, 0.3200000000000000067, 0.3300000000000000155, 0.3400000000000000244, 0.3499999999999999778, 0.3599999999999999867, 0.3699999999999999956, 0.3800000000000000044, 0.3900000000000000133, 0.4000000000000000222, 0.4099999999999999756, 0.4199999999999999845, 0.4299999999999999933, 0.4400000000000000022, 0.4500000000000000111, 0.4600000000000000200, 0.4699999999999999734, 0.4799999999999999822, 0.4899999999999999911, 0.5000000000000000000, 0.5100000000000000089, 0.5200000000000000178, 0.5300000000000000266, 0.5400000000000000355, 0.5500000000000000444, 0.5600000000000000533, 0.5699999999999999512, 0.5799999999999999600, 0.5899999999999999689, 0.5999999999999999778, 0.6099999999999999867, 0.6199999999999999956, 0.6300000000000000044, 0.6400000000000000133, 0.6500000000000000222, 0.6600000000000000311, 0.6700000000000000400, 0.6800000000000000488, 0.6899999999999999467, 0.6999999999999999556, 0.7099999999999999645, 0.7199999999999999734, 0.7299999999999999822, 0.7399999999999999911, 0.7500000000000000000, 0.7600000000000000089, 0.7700000000000000178, 0.7800000000000000266, 0.7900000000000000355, 0.8000000000000000444, 0.8100000000000000533, 0.8199999999999999512, 0.8299999999999999600, 0.8399999999999999689, 0.8499999999999999778, 0.8599999999999999867, 0.8699999999999999956, 0.8800000000000000044, 0.8900000000000000133, 0.9000000000000000222, 0.9100000000000000311, 0.9200000000000000400, 0.9300000000000000488, 0.9399999999999999467, 0.9499999999999999556, 0.9599999999999999645, 0.9699999999999999734, 0.9799999999999999822, 0.9899999999999999911, 1.000000000000000000 ),
 .UNSPECIFIED. ) 
 CURVE ( )  GEOMETRIC_REPRESENTATION_ITEM ( )  RATIONAL_B_SPLINE_CURVE ( ( 0.9826544568871729002, 0.9623225587740311671, 1.000000000000000000, 0.9510565162951535312, 1.000000000000000000, 0.9510565162951535312, 1.000000000000000000, 0.9510565162951535312, 1.000000000000000000, 0.9510565162951535312, 1.000000000000000000, 0.9510565162951535312, 1.000000000000000000, 0.9510565162951535312, 1.000000000000000000, 0.9510565162951535312, 1.000000000000000000, 0.9510565162951535312, 1.000000000000000000, 0.9510565162951535312, 1.000000000000000000, 0.9510565162951535312, 1.000000000000000000, 0.9510565162951535312, 1.000000000000000000, 0.9510565162951535312, 1.000000000000000000, 0.9510565162951535312, 1.000000000000000000, 0.9510565162951535312, 1.000000000000000000, 0.9510565162951535312, 1.000000000000000000, 0.9510565162951535312, 1.000000000000000000, 0.9510565162951535312, 1.000000000000000000, 0.9510565162951535312, 1.000000000000000000, 0.9510565162951535312, 1.000000000000000000, 0.9510565162951535312, 1.000000000000000000, 0.9510565162951535312, 1.000000000000000000, 0.9510565162951535312, 1.000000000000000000, 0.9510565162951535312, 1.000000000000000000, 0.9510565162951535312, 1.000000000000000000, 0.9510565162951535312, 1.000000000000000000, 0.9510565162951535312, 1.000000000000000000, 0.9510565162951535312, 1.000000000000000000, 0.9510565162951535312, 1.000000000000000000, 0.9510565162951535312, 1.000000000000000000, 0.9510565162951535312, 1.000000000000000000, 0.9510565162951535312, 1.000000000000000000, 0.9510565162951535312, 1.000000000000000000, 0.9510565162951535312, 1.000000000000000000, 0.9510565162951535312, 1.000000000000000000, 0.9510565162951535312, 1.000000000000000000, 0.9510565162951535312, 1.000000000000000000, 0.9510565162951535312, 1.000000000000000000, 0.9510565162951535312, 1.000000000000000000, 0.9510565162951535312, 1.000000000000000000, 0.9510565162951535312, 1.000000000000000000, 0.9510565162951535312, 1.000000000000000000, 0.9510565162951535312, 1.000000000000000000, 0.9510565162951535312, 1.000000000000000000, 0.9510565162951535312, 1.000000000000000000, 0.9510565162951535312, 1.000000000000000000, 0.9510565162951535312, 1.000000000000000000, 0.9510565162951535312, 1.000000000000000000, 0.9510565162951535312, 1.000000000000000000, 0.9510565162951535312, 1.000000000000000000, 0.9510565162951535312, 1.000000000000000000, 0.9510565162951535312, 1.000000000000000000, 0.9510565162951535312, 1.000000000000000000, 0.9510565162951535312, 1.000000000000000000, 0.9510565162951535312, 1.000000000000000000, 0.9510565162951535312, 1.000000000000000000, 0.9510565162951535312, 1.000000000000000000, 0.9510565162951535312, 1.000000000000000000, 0.9510565162951535312, 1.000000000000000000, 0.9510565162951535312, 1.000000000000000000, 0.9510565162951535312, 1.000000000000000000, 0.9510565162951535312, 1.000000000000000000, 0.9510565162951535312, 1.000000000000000000, 0.9510565162951535312, 1.000000000000000000, 0.9510565162951535312, 1.000000000000000000, 0.9510565162951535312, 1.000000000000000000, 0.9510565162951535312, 1.000000000000000000, 0.9510565162951535312, 1.000000000000000000, 0.9510565162951535312, 1.000000000000000000, 0.9510565162951535312, 1.000000000000000000, 0.9510565162951535312, 1.000000000000000000, 0.9510565162951535312, 1.000000000000000000, 0.9510565162951535312, 1.000000000000000000, 0.9510565162951535312, 1.000000000000000000, 0.9510565162951535312, 1.000000000000000000, 0.9510565162951535312, 1.000000000000000000, 0.9510565162951535312, 1.000000000000000000, 0.9510565162951535312, 1.000000000000000000, 0.9510565162951535312, 1.000000000000000000, 0.9510565162951535312, 1.000000000000000000, 0.9510565162951535312, 1.000000000000000000, 0.9510565162951535312, 1.000000000000000000, 0.9510565162951535312, 1.000000000000000000, 0.9510565162951535312, 1.000000000000000000, 0.9510565162951535312, 1.000000000000000000, 0.9510565162951535312, 1.000000000000000000, 0.9510565162951535312, 1.000000000000000000, 0.9510565162951535312, 1.000000000000000000, 0.9510565162951535312, 1.000000000000000000, 0.9510565162951535312, 1.000000000000000000, 0.9510565162951535312, 1.000000000000000000, 0.9510565162951535312, 1.000000000000000000, 0.9510565162951535312, 1.000000000000000000, 0.9510565162951535312, 1.000000000000000000, 0.9510565162951535312, 1.000000000000000000, 0.9510565162951535312, 1.000000000000000000, 0.9510565162951535312, 1.000000000000000000, 0.9510565162951535312, 1.000000000000000000, 0.9510565162951535312, 1.000000000000000000 ) ) 
 REPRESENTATION_ITEM ( '' )  );
#15315=LINE ( 'NONE', #15217, #14100 ) ;
#15321=CARTESIAN_POINT ( 'NONE',  ( 45.86712807150329496, 47.70051614449766220, 5.649768623646139964 ) ) ;
#15324=CARTESIAN_POINT ( 'NONE',  ( 47.74827507625478518, 64.59948385550239891, 7.007379884777227730 ) ) ;
#15329=CARTESIAN_POINT ( 'NONE',  ( 44.88205777487398507, 61.19948385550241454, -3.688883143319540814 ) ) ;
#15333=CARTESIAN_POINT ( 'NONE',  ( 42.38452918213190657, 57.90051614449765793, 2.450534656007115508 ) ) ;
#15334=CARTESIAN_POINT ( 'NONE',  ( 53.54508667620424234, 56.70051614449766930, -4.840751629271188961 ) ) ;
#15346=CARTESIAN_POINT ( 'NONE',  ( 45.86712807150323812, 49.29948385550240175, -5.649768623646098220 ) ) ;
#15350=CARTESIAN_POINT ( 'NONE',  ( 43.20883090819745576, 54.79948385550240175, 4.963592699179006473 ) ) ;
#15353=CARTESIAN_POINT ( 'NONE',  ( 55.11794222512601493, 46.19948385550240744, 3.688883143319541702 ) ) ;
#15358=CARTESIAN_POINT ( 'NONE',  ( 55.94051828345053679, 63.20051614449765509, 4.345558710429044069 ) ) ;
#15361=CARTESIAN_POINT ( 'NONE',  ( 43.34962307344081012, 52.89948385550240317, 2.184720259617164650 ) ) ;
#15366=CARTESIAN_POINT ( 'NONE',  ( 45.90387839640214196, 50.69948385550240744, 5.676469297603166098 ) ) ;
#15371=AXIS2_PLACEMENT_3D ( 'NONE', #9922, #18780, #11300 ) ;
#15374=CARTESIAN_POINT ( 'NONE',  ( 54.13287192849671214, 62.70051614449766220, -5.649768623646139964 ) ) ;
#15379=CARTESIAN_POINT ( 'NONE',  ( 46.49166364869456913, 56.30051614449766362, -4.867452303228181343 ) ) ;
#15385=CARTESIAN_POINT ( 'NONE',  ( 56.79116909180259398, 59.20051614449766220, 4.963592699178938972 ) ) ;
#15405=CARTESIAN_POINT ( 'NONE',  ( 47.70284917648453415, 63.39948385550240317, -6.992620115222774047 ) ) ;
#15407=CARTESIAN_POINT ( 'NONE',  ( 45.27934281921075410, 59.29948385550240886, -6.458785618021043895 ) ) ;
#15408=CARTESIAN_POINT ( 'NONE',  ( 43.33558569842706021, 59.90051614449766504, 2.141517661632167169 ) ) ;
#15414=CARTESIAN_POINT ( 'NONE',  ( 44.03140696652198471, 47.80051614449764941, 4.306917132069485454 ) ) ;
#15415=CARTESIAN_POINT ( 'NONE',  ( 43.34962307344081012, 64.89948385550239607, 2.184720259617164650 ) ) ;
#15421=CARTESIAN_POINT ( 'NONE',  ( 48.07319477248768180, 60.59948385550240602, 6.007379884777225953 ) ) ;
#15427=CARTESIAN_POINT ( 'NONE',  ( 43.20883090819742023, 58.20051614449766220, -4.963592699178938972 ) ) ;
#15428=CARTESIAN_POINT ( 'NONE',  ( 52.29715082351538769, 44.60051614449766788, -6.992620115222796251 ) ) ;
#15440=CARTESIAN_POINT ( 'NONE',  ( 47.70284917648453415, 53.39948385550239607, -6.992620115222774047 ) ) ;
#15445=CARTESIAN_POINT ( 'NONE',  ( 52.57664461997811856, 51.59948385550240602, -8.007379884777229506 ) ) ;
#15448=CARTESIAN_POINT ( 'NONE',  ( 56.65037692655918988, 61.89948385550241028, -2.184720259617163762 ) ) ;
#15451=CARTESIAN_POINT ( 'NONE',  ( 47.74827507625469281, 62.40051614449766504, -7.007379884777203749 ) ) ;
#15453=CARTESIAN_POINT ( 'NONE',  ( 57.36023556966787851, 59.99948385550240459, -0.02388180880522424582 ) ) ;
#15459=CARTESIAN_POINT ( 'NONE',  ( 45.86712807150323812, 53.29948385550240886, -5.649768623646098220 ) ) ;
#15469=CARTESIAN_POINT ( 'NONE',  ( 55.08986747509849380, 63.20051614449766220, 3.727524721679155384 ) ) ;
#15475=CARTESIAN_POINT ( 'NONE',  ( 43.20883090819742023, 58.20051614449766220, -4.963592699178938972 ) ) ;
#15479=( NAMED_UNIT ( * ) PLANE_ANGLE_UNIT ( ) SI_UNIT ( $, .RADIAN. ) );
#15496=CARTESIAN_POINT ( 'NONE',  ( 44.03140696652192787, 63.19948385550240744, -4.306917132069425058 ) ) ;
#15498=CARTESIAN_POINT ( 'NONE',  ( 56.79116909180255135, 57.79948385550240175, -4.963592699179005585 ) ) ;
#15499=CARTESIAN_POINT ( 'NONE',  ( 52.29715082351538769, 60.60051614449764656, -6.992620115222796251 ) ) ;
#15509=ADVANCED_FACE ( 'NONE', ( #13291 ), #10343, .F. ) ;
#15511=CARTESIAN_POINT ( 'NONE',  ( 54.89903213687075834, 44.74560054925188268, -5.000000000000007105 ) ) ;
#15519=CARTESIAN_POINT ( 'NONE',  ( 44.91013252490152752, 60.79948385550241596, 3.727524721679198461 ) ) ;
#15521=CARTESIAN_POINT ( 'NONE',  ( 52.25172492374522903, 45.59948385550240602, -7.007379884777225953 ) ) ;
#15523=CARTESIAN_POINT ( 'NONE',  ( 41.58830220609386430, 60.00051614449765935, -0.02388180880514929535 ) ) ;
#15525=CARTESIAN_POINT ( 'NONE',  ( 53.50833635130544508, 63.30051614449767072, 4.867452303228181343 ) ) ;
#15537=CARTESIAN_POINT ( 'NONE',  ( 42.63976443033212149, 50.99948385550240459, 0.02388180880522514787 ) ) ;
#15541=CARTESIAN_POINT ( 'NONE',  ( 43.18075615816989199, 51.19948385550240744, -4.924951120819313743 ) ) ;
#15543=CARTESIAN_POINT ( 'NONE',  ( 57.36023556966787851, 61.99948385550241170, -0.02388180880522424582 ) ) ;
#15546=CARTESIAN_POINT ( 'NONE',  ( 54.13287192849671214, 58.70051614449765509, -5.649768623646139964 ) ) ;
#15547=CARTESIAN_POINT ( 'NONE',  ( 45.86712807150323812, 57.29948385550240175, -5.649768623646098220 ) ) ;
#15558=CARTESIAN_POINT ( 'NONE',  ( 43.33558569842703179, 53.09948385550240602, -2.141517661632099223 ) ) ;
#15569=CARTESIAN_POINT ( 'NONE',  ( 50.02271294988512551, 46.49948385550240459, 7.000000000000000888 ) ) ;
#15571=CARTESIAN_POINT ( 'NONE',  ( 46.49166364869456913, 60.30051614449767072, -4.867452303228181343 ) ) ;
#15576=CARTESIAN_POINT ( 'NONE',  ( 57.61547081786810764, 58.90051614449766504, -2.450534656007114176 ) ) ;
#15581=SURFACE_STYLE_FILL_AREA ( #6845 ) ;
#15595=CARTESIAN_POINT ( 'NONE',  ( 53.50833635130540955, 45.69948385550240033, -4.867452303228209765 ) ) ;
#15597=CARTESIAN_POINT ( 'NONE',  ( 57.61547081786812896, 62.09948385550240602, 2.450534656007040901 ) ) ;
#15599=CARTESIAN_POINT ( 'NONE',  ( 54.13287192849671214, 62.70051614449766220, -5.649768623646139964 ) ) ;
#15608=CARTESIAN_POINT ( 'NONE',  ( 45.86712807150329496, 51.70051614449766220, 5.649768623646139964 ) ) ;
#15618=CARTESIAN_POINT ( 'NONE',  ( 52.25172492374522903, 47.59948385550239891, -7.007379884777225953 ) ) ;
#15620=CARTESIAN_POINT ( 'NONE',  ( 42.38452918213190657, 59.90051614449767214, 2.450534656007115508 ) ) ;
#15622=CARTESIAN_POINT ( 'NONE',  ( 55.69932041026405045, 59.10051614449766078, 1.875703265242156359 ) ) ;
#15638=CARTESIAN_POINT ( 'NONE',  ( 50.02271294988512551, 60.49948385550240459, 7.000000000000000888 ) ) ;
#15642=CARTESIAN_POINT ( 'NONE',  ( 58.41169779390614281, 53.99948385550241170, -0.02388180880523160798 ) ) ;
#15644=CARTESIAN_POINT ( 'NONE',  ( 54.09612160359786515, 61.69948385550240744, -5.676469297603166098 ) ) ;
#15647=CARTESIAN_POINT ( 'NONE',  ( 44.05948171654945611, 58.20051614449764799, -4.345558710429044069 ) ) ;
#15650=CARTESIAN_POINT ( 'NONE',  ( 44.28664221472220675, 63.09948385550240602, -1.832500667257165317 ) ) ;
#15652=CARTESIAN_POINT ( 'NONE',  ( 54.13287192849676188, 58.29948385550240175, 5.649768623646098220 ) ) ;
#15659=CARTESIAN_POINT ( 'NONE',  ( 47.74827507625478518, 54.59948385550239180, 7.007379884777227730 ) ) ;
#15671=CARTESIAN_POINT ( 'NONE',  ( 42.63976443033212860, 46.99948385550240459, 0.02388180880522514787 ) ) ;
#15673=CARTESIAN_POINT ( 'NONE',  ( 44.91013252490150620, 64.20051614449766930, -3.727524721679154940 ) ) ;
#15701=CARTESIAN_POINT ( 'NONE',  ( 43.69122665457040000, 46.99948385550239749, 0.02388180880521036456 ) ) ;
#15703=CARTESIAN_POINT ( 'NONE',  ( 54.13287192849676188, 48.29948385550240175, 5.649768623646098220 ) ) ;
#15704=CARTESIAN_POINT ( 'NONE',  ( 55.96859303347802239, 62.80051614449766362, -4.306917132069484566 ) ) ;
#15713=CARTESIAN_POINT ( 'NONE',  ( 56.66441430157294690, 54.90051614449765793, -2.141517661632166281 ) ) ;
#15714=CARTESIAN_POINT ( 'NONE',  ( 55.31939397794342028, 44.99999999999998579, -5.196074157289758411 ) ) ;
#15720=CARTESIAN_POINT ( 'NONE',  ( 49.97728705011488159, 47.49948385550240459, -7.000000000000000888 ) ) ;
#15722=CARTESIAN_POINT ( 'NONE',  ( 58.41169779390614281, 59.00051614449766646, 0.02388180880515032231 ) ) ;
#15723=CARTESIAN_POINT ( 'NONE',  ( 49.97728705011494554, 63.50051614449765935, 6.000000000000000888 ) ) ;
#15737=CARTESIAN_POINT ( 'NONE',  ( 44.05948171654949874, 58.79948385550240175, 4.345558710429104465 ) ) ;
#15741=CARTESIAN_POINT ( 'NONE',  ( 47.37792948025162332, 51.39948385550241028, -7.992620115222770494 ) ) ;
#15745=CARTESIAN_POINT ( 'NONE',  ( 48.02776887271745210, 49.39948385550241028, -5.992620115222778487 ) ) ;
#15748=CARTESIAN_POINT ( 'NONE',  ( 43.33558569842706021, 61.90051614449766504, 2.141517661632167169 ) ) ;
#15750=CARTESIAN_POINT ( 'NONE',  ( 53.50833635130544508, 45.30051614449766362, 4.867452303228181343 ) ) ;
#15752=CARTESIAN_POINT ( 'NONE',  ( 56.65037692655918988, 57.89948385550240317, -2.184720259617163762 ) ) ;
#15762=CARTESIAN_POINT ( 'NONE',  ( 55.96859303347804371, 58.19948385550241454, 4.306917132069425946 ) ) ;
#15772=CARTESIAN_POINT ( 'NONE',  ( 54.13287192849676188, 48.29948385550240175, 5.649768623646098220 ) ) ;
#15774=CARTESIAN_POINT ( 'NONE',  ( 44.88205777487401349, 63.80051614449766362, 3.688883143319584779 ) ) ;
#15795=CARTESIAN_POINT ( 'NONE',  ( 51.97223112728254790, 50.39948385550241738, 5.992620115222778487 ) ) ;
#15797=CARTESIAN_POINT ( 'NONE',  ( 47.37792948025162332, 65.39948385550239607, -7.992620115222770494 ) ) ;
#15798=CARTESIAN_POINT ( 'NONE',  ( 43.33558569842706021, 61.90051614449766504, 2.141517661632167169 ) ) ;
#15808=CARTESIAN_POINT ( 'NONE',  ( 52.25172492374528588, 55.40051614449765083, 7.007379884777204637 ) ) ;
#15812=ORIENTED_EDGE ( 'NONE', *, *, #19249, .T. ) ;
#15816=FACE_OUTER_BOUND ( 'NONE', #830, .T. ) ;
#15819=CARTESIAN_POINT ( 'NONE',  ( 47.37792948025170858, 63.60051614449764656, 7.992620115222797139 ) ) ;
#15822=CARTESIAN_POINT ( 'NONE',  ( 55.69932041026405045, 63.10051614449766078, 1.875703265242156359 ) ) ;
#15833=CARTESIAN_POINT ( 'NONE',  ( 47.74827507625477807, 58.59948385550239180, 7.007379884777229506 ) ) ;
#15837=CARTESIAN_POINT ( 'NONE',  ( 42.39856655714566358, 56.89948385550240317, 2.493737253992119207 ) ) ;
#15839=CARTESIAN_POINT ( 'NONE',  ( 46.49166364869460466, 50.69948385550240744, 4.867452303228209765 ) ) ;
#15842=CARTESIAN_POINT ( 'NONE',  ( 42.63976443033212860, 64.00051614449765225, -0.02388180880514948964 ) ) ;
#15843=CARTESIAN_POINT ( 'NONE',  ( 55.69932041026404335, 61.89948385550241738, -1.875703265242203432 ) ) ;
#15855=CARTESIAN_POINT ( 'NONE',  ( 56.65037692655918988, 59.89948385550241028, -2.184720259617163762 ) ) ;
#15864=CARTESIAN_POINT ( 'NONE',  ( 55.94051828345050836, 53.79948385550238754, -4.345558710429104465 ) ) ;
#15868=CARTESIAN_POINT ( 'NONE',  ( 44.03140696652198471, 45.80051614449764230, 4.306917132069485454 ) ) ;
#15889=CARTESIAN_POINT ( 'NONE',  ( 50.02271294988511841, 62.49948385550240459, 6.000000000000000888 ) ) ;
#15893=CARTESIAN_POINT ( 'NONE',  ( 53.54508667620428497, 50.29948385550240886, 4.840751629271157874 ) ) ;
#15896=CARTESIAN_POINT ( 'NONE',  ( 43.34962307344081012, 48.89948385550240317, 2.184720259617164650 ) ) ;
#15897=CARTESIAN_POINT ( 'NONE',  ( 42.39856655714564226, 46.10051614449766078, -2.493737253992044156 ) ) ;
#15906=CARTESIAN_POINT ( 'NONE',  ( 52.25172492374528588, 51.40051614449767214, 7.007379884777204637 ) ) ;
#15914=CARTESIAN_POINT ( 'NONE',  ( 57.36023556966787851, 51.99948385550238328, -0.02388180880522424582 ) ) ;
#15916=CARTESIAN_POINT ( 'NONE',  ( 42.38452918213190657, 63.90051614449765793, 2.450534656007115508 ) ) ;
#15920=CARTESIAN_POINT ( 'NONE',  ( 54.09612160359792199, 51.30051614449766362, 5.676469297603124353 ) ) ;
#15932=CARTESIAN_POINT ( 'NONE',  ( 50.02271294988512551, 56.49948385550240459, 7.000000000000000888 ) ) ;
#15937=CARTESIAN_POINT ( 'NONE',  ( 56.79116909180255135, 57.79948385550240175, -4.963592699179005585 ) ) ;
#15939=CARTESIAN_POINT ( 'NONE',  ( 55.71335778527780747, 50.09948385550240602, 1.832500667257165983 ) ) ;
#15942=CARTESIAN_POINT ( 'NONE',  ( 45.31609314410960820, 48.30051614449765651, -6.485486291978072693 ) ) ;
#15943=CARTESIAN_POINT ( 'NONE',  ( 51.97223112728249816, 44.60051614449766078, -5.992620115222793586 ) ) ;
#15954=CARTESIAN_POINT ( 'NONE',  ( 43.33558569842703179, 59.09948385550240602, -2.141517661632099223 ) ) ;
#15965=CARTESIAN_POINT ( 'NONE',  ( 44.05948171654949874, 52.79948385550240175, 4.345558710429105354 ) ) ;
#15967=CARTESIAN_POINT ( 'NONE',  ( 56.65037692655921120, 49.10051614449766078, 2.184720259617097593 ) ) ;
#15985=CARTESIAN_POINT ( 'NONE',  ( 53.50833635130544508, 51.30051614449765651, 4.867452303228181343 ) ) ;
#15990=CARTESIAN_POINT ( 'NONE',  ( 51.92680522751233951, 53.59948385550240602, -6.007379884777223289 ) ) ;
#15994=CARTESIAN_POINT ( 'NONE',  ( 42.38452918213188525, 65.09948385550239891, -2.450534656007040013 ) ) ;
#15995=CARTESIAN_POINT ( 'NONE',  ( 57.60143344285435774, 47.10051614449766078, 2.493737253992045044 ) ) ;
#16010=CARTESIAN_POINT ( 'NONE',  ( 54.13287192849671214, 52.70051614449766220, -5.649768623646139964 ) ) ;
#16018=CARTESIAN_POINT ( 'NONE',  ( 49.97728705011488159, 53.49948385550240459, -7.000000000000000888 ) ) ;
#16020=CARTESIAN_POINT ( 'NONE',  ( 41.58830220609386430, 64.00051614449765225, -0.02388180880514929535 ) ) ;
#16021=CARTESIAN_POINT ( 'NONE',  ( 45.86712807150329496, 49.70051614449766220, 5.649768623646139964 ) ) ;
#16038=CARTESIAN_POINT ( 'NONE',  ( 47.42335538002188144, 58.59948385550239891, 8.007379884777233059 ) ) ;
#16041=CARTESIAN_POINT ( 'NONE',  ( 44.88205777487398507, 49.19948385550240744, -3.688883143319540814 ) ) ;
#16046=CARTESIAN_POINT ( 'NONE',  ( 43.18075615816994173, 45.80051614449766362, 4.924951120819380357 ) ) ;
#16047=CARTESIAN_POINT ( 'NONE',  ( 56.30877334542961421, 47.00051614449766646, 0.02388180880515774693 ) ) ;
#16056=CARTESIAN_POINT ( 'NONE',  ( 52.25172492374522903, 59.59948385550240602, -7.007379884777225953 ) ) ;
#16067=CARTESIAN_POINT ( 'NONE',  ( 52.25172492374522903, 51.59948385550240602, -7.007379884777225953 ) ) ;
#16069=CARTESIAN_POINT ( 'NONE',  ( 45.86712807150329496, 47.70051614449766220, 5.649768623646139964 ) ) ;
#16087=CARTESIAN_POINT ( 'NONE',  ( 46.45491332379576477, 47.70051614449766220, 4.840751629271188961 ) ) ;
#16090=CARTESIAN_POINT ( 'NONE',  ( 56.30877334542961421, 53.99948385550241170, -0.02388180880520959434 ) ) ;
#16092=CARTESIAN_POINT ( 'NONE',  ( 45.31609314410967926, 64.69948385550240744, 6.485486291978119766 ) ) ;
#16093=CARTESIAN_POINT ( 'NONE',  ( 43.18075615816994173, 45.80051614449766362, 4.924951120819380357 ) ) ;
#16113=CARTESIAN_POINT ( 'NONE',  ( 52.25172492374522903, 49.59948385550240602, -7.007379884777225953 ) ) ;
#16116=CARTESIAN_POINT ( 'NONE',  ( 58.41169779390614281, 49.99948385550240459, -0.02388180880523160798 ) ) ;
#16117=CARTESIAN_POINT ( 'NONE',  ( 45.90387839640208512, 48.30051614449765651, -5.676469297603124353 ) ) ;
#16135=CARTESIAN_POINT ( 'NONE',  ( 41.58830220609386430, 58.99948385550239749, 0.02388180880523263147 ) ) ;
#16138=CARTESIAN_POINT ( 'NONE',  ( 53.50833635130540955, 53.69948385550240744, -4.867452303228209765 ) ) ;
#16142=CARTESIAN_POINT ( 'NONE',  ( 54.72065718078918906, 44.70051614449765509, -6.458785618021089192 ) ) ;
#16144=CARTESIAN_POINT ( 'NONE',  ( 49.97728705011494554, 47.50051614449765935, 6.000000000000000888 ) ) ;
#16151=CARTESIAN_POINT ( 'NONE',  ( 47.74827507625478518, 58.59948385550238470, 7.007379884777227730 ) ) ;
#16162=CARTESIAN_POINT ( 'NONE',  ( 42.63976443033212860, 48.99948385550240459, 0.02388180880522514787 ) ) ;
#16164=CARTESIAN_POINT ( 'NONE',  ( 44.03140696652198471, 47.80051614449764230, 4.306917132069485454 ) ) ;
#16181=CARTESIAN_POINT ( 'NONE',  ( 48.02776887271750184, 47.60051614449766078, 5.992620115222795363 ) ) ;
#16184=CARTESIAN_POINT ( 'NONE',  ( 46.45491332379572924, 49.29948385550240886, -4.840751629271157874 ) ) ;
#16186=CARTESIAN_POINT ( 'NONE',  ( 54.13287192849676188, 54.29948385550240886, 5.649768623646098220 ) ) ;
#16187=CARTESIAN_POINT ( 'NONE',  ( 47.37792948025170858, 49.60051614449766788, 7.992620115222797139 ) ) ;
#16191=DIRECTION ( 'NONE',  ( 1.000000000000000000, 0.000000000000000000, 0.000000000000000000 ) ) ;
#16195=CLOSED_SHELL ( 'NONE', ( #8905, #12022, #15509, #17720, #7239, #7057 ) ) ;
#16206=CARTESIAN_POINT ( 'NONE',  ( 47.74827507625478518, 50.59948385550238470, 7.007379884777227730 ) ) ;
#16208=CARTESIAN_POINT ( 'NONE',  ( 57.61547081786812896, 54.09948385550241312, 2.450534656007040901 ) ) ;
#16210=CARTESIAN_POINT ( 'NONE',  ( 43.34962307344078880, 50.10051614449766078, -2.184720259617096705 ) ) ;
#16227=CARTESIAN_POINT ( 'NONE',  ( 56.81924384183011512, 62.19948385550240744, 4.924951120819313743 ) ) ;
#16231=CARTESIAN_POINT ( 'NONE',  ( 48.02776887271745210, 55.39948385550240317, -5.992620115222778487 ) ) ;
#16235=CARTESIAN_POINT ( 'NONE',  ( 54.68390685589039890, 47.30051614449766362, 6.485486291978072693 ) ) ;
#16236=CARTESIAN_POINT ( 'NONE',  ( 46.45491332379576477, 51.70051614449765509, 4.840751629271188961 ) ) ;
#16250=CARTESIAN_POINT ( 'NONE',  ( 57.36023556966787851, 45.99948385550239749, -0.02388180880522424582 ) ) ;
#16257=CARTESIAN_POINT ( 'NONE',  ( 52.29715082351547295, 54.39948385550239607, 6.992620115222774047 ) ) ;
#16260=CARTESIAN_POINT ( 'NONE',  ( 49.97728705011495265, 47.50051614449766646, 7.000000000000000888 ) ) ;
#16271=CARTESIAN_POINT ( 'NONE',  ( 50.02271294988512551, 46.49948385550240459, 7.000000000000000888 ) ) ;
#16285=CARTESIAN_POINT ( 'NONE',  ( 49.97728705011494554, 49.50051614449766646, 6.000000000000000888 ) ) ;
#16289=CARTESIAN_POINT ( 'NONE',  ( 50.02271294988511841, 60.49948385550240459, 6.000000000000000888 ) ) ;
#16291=CARTESIAN_POINT ( 'NONE',  ( 47.70284917648453415, 51.39948385550238896, -6.992620115222774047 ) ) ;
#16293=CARTESIAN_POINT ( 'NONE',  ( 47.42335538002180328, 48.40051614449766504, -8.007379884777206414 ) ) ;
#16311=CARTESIAN_POINT ( 'NONE',  ( 57.36023556966787851, 55.99948385550239038, -0.02388180880522424582 ) ) ;
#16314=CARTESIAN_POINT ( 'NONE',  ( 42.39856655714566358, 54.89948385550240317, 2.493737253992119207 ) ) ;
#16315=CARTESIAN_POINT ( 'NONE',  ( 56.66441430157294690, 50.90051614449766504, -2.141517661632166281 ) ) ;
#16331=CARTESIAN_POINT ( 'NONE',  ( 55.11794222512601493, 60.19948385550240744, 3.688883143319541702 ) ) ;
#16336=CARTESIAN_POINT ( 'NONE',  ( 58.41169779390614281, 51.00051614449765935, 0.02388180880515032231 ) ) ;
#16337=CARTESIAN_POINT ( 'NONE',  ( 53.54508667620424234, 50.70051614449766220, -4.840751629271188961 ) ) ;
#16345=CARTESIAN_POINT ( 'NONE',  ( 43.33558569842703179, 63.09948385550240602, -2.141517661632099223 ) ) ;
#16351=CARTESIAN_POINT ( 'NONE',  ( 42.63976443033212149, 46.99948385550240459, 0.02388180880522514787 ) ) ;
#16360=CARTESIAN_POINT ( 'NONE',  ( 47.74827507625478518, 56.59948385550238470, 7.007379884777227730 ) ) ;
#16362=CARTESIAN_POINT ( 'NONE',  ( 57.36023556966787851, 53.00051614449765225, 0.02388180880515038476 ) ) ;
#16373=CARTESIAN_POINT ( 'NONE',  ( 47.42335538002188144, 64.59948385550241312, 8.007379884777233059 ) ) ;
#16380=CARTESIAN_POINT ( 'NONE',  ( 52.25172492374528588, 57.40051614449765793, 7.007379884777204637 ) ) ;
#16385=CARTESIAN_POINT ( 'NONE',  ( 51.97223112728249816, 50.60051614449765367, -5.992620115222793586 ) ) ;
#16388=CARTESIAN_POINT ( 'NONE',  ( 51.97223112728254790, 54.39948385550241028, 5.992620115222778487 ) ) ;
#16390=CARTESIAN_POINT ( 'NONE',  ( 42.63976443033212860, 54.99948385550241170, 0.02388180880522514787 ) ) ;
#16391=CARTESIAN_POINT ( 'NONE',  ( 58.41169779390614281, 57.00051614449766646, 0.02388180880515032231 ) ) ;
#16406=CARTESIAN_POINT ( 'NONE',  ( 47.74827507625478518, 60.59948385550239891, 7.007379884777227730 ) ) ;
#16408=CARTESIAN_POINT ( 'NONE',  ( 45.31609314410967926, 56.69948385550240744, 6.485486291978119766 ) ) ;
#16410=CARTESIAN_POINT ( 'NONE',  ( 45.86712807150329496, 57.70051614449765509, 5.649768623646139964 ) ) ;
#16428=CARTESIAN_POINT ( 'NONE',  ( 50.02271294988511841, 54.49948385550240459, 6.000000000000000888 ) ) ;
#16432=CARTESIAN_POINT ( 'NONE',  ( 58.41169779390614281, 53.00051614449765935, 0.02388180880515032231 ) ) ;
#16434=CARTESIAN_POINT ( 'NONE',  ( 53.50833635130544508, 49.30051614449766362, 4.867452303228181343 ) ) ;
#16441=CARTESIAN_POINT ( 'NONE',  ( 54.13287192849676188, 62.29948385550240886, 5.649768623646098220 ) ) ;
#16450=CARTESIAN_POINT ( 'NONE',  ( 50.02271294988505446, 62.50051614449767357, -8.000000000000001776 ) ) ;
#16453=CARTESIAN_POINT ( 'NONE',  ( 45.90387839640214196, 60.69948385550240033, 5.676469297603166098 ) ) ;
#16456=CARTESIAN_POINT ( 'NONE',  ( 55.94051828345053679, 53.20051614449766220, 4.345558710429044069 ) ) ;
#16467=CARTESIAN_POINT ( 'NONE',  ( 52.62207051974839089, 64.39948385550239607, 7.992620115222770494 ) ) ;
#16473=CARTESIAN_POINT ( 'NONE',  ( 44.03140696652198471, 61.80051614449766362, 4.306917132069485454 ) ) ;
#16477=CARTESIAN_POINT ( 'NONE',  ( 56.30877334542961421, 53.00051614449765935, 0.02388180880515774693 ) ) ;
#16483=CARTESIAN_POINT ( 'NONE',  ( 44.28664221472220675, 55.09948385550241312, -1.832500667257165317 ) ) ;
#16485=CARTESIAN_POINT ( 'NONE',  ( 43.20883090819742023, 52.20051614449766220, -4.963592699178938972 ) ) ;
#16498=CARTESIAN_POINT ( 'NONE',  ( 52.29715082351547295, 64.39948385550239607, 6.992620115222774047 ) ) ;
#16502=CARTESIAN_POINT ( 'NONE',  ( 45.90387839640214196, 58.69948385550240033, 5.676469297603166098 ) ) ;
#16505=CARTESIAN_POINT ( 'NONE',  ( 56.79116909180255135, 51.79948385550240175, -4.963592699179005585 ) ) ;
#16507=CARTESIAN_POINT ( 'NONE',  ( 52.25172492374527877, 53.40051614449765793, 7.007379884777203749 ) ) ;
#16518=CARTESIAN_POINT ( 'NONE',  ( 52.25172492374522903, 63.59948385550237759, -7.007379884777225953 ) ) ;
#16524=CARTESIAN_POINT ( 'NONE',  ( 53.54508667620428497, 54.29948385550241596, 4.840751629271157874 ) ) ;
#16528=CARTESIAN_POINT ( 'NONE',  ( 43.18075615816994173, 53.80051614449766362, 4.924951120819380357 ) ) ;
#16529=CARTESIAN_POINT ( 'NONE',  ( 49.97728705011494554, 53.50051614449767357, 6.000000000000000888 ) ) ;
#16537=CARTESIAN_POINT ( 'NONE',  ( 47.74827507625478518, 64.59948385550239891, 7.007379884777227730 ) ) ;
#16548=CARTESIAN_POINT ( 'NONE',  ( 47.37792948025170858, 63.60051614449764656, 7.992620115222797139 ) ) ;
#16549=CARTESIAN_POINT ( 'NONE',  ( 50.38494826773854385, 45.00000000000002842, -6.500000000000005329 ) ) ;
#16550=CARTESIAN_POINT ( 'NONE',  ( 52.25172492374522903, 55.59948385550241312, -7.007379884777225953 ) ) ;
#16553=CARTESIAN_POINT ( 'NONE',  ( 52.25172492374527877, 51.40051614449767214, 7.007379884777203749 ) ) ;
#16563=CARTESIAN_POINT ( 'NONE',  ( 57.60143344285433642, 63.89948385550240317, -2.493737253992118319 ) ) ;
#16568=CARTESIAN_POINT ( 'NONE',  ( 45.90387839640208512, 58.30051614449766362, -5.676469297603124353 ) ) ;
#16575=CARTESIAN_POINT ( 'NONE',  ( 44.91013252490150620, 54.20051614449766220, -3.727524721679154940 ) ) ;
#16578=CARTESIAN_POINT ( 'NONE',  ( 55.71335778527780747, 58.09948385550241312, 1.832500667257165983 ) ) ;
#16580=CARTESIAN_POINT ( 'NONE',  ( 49.97728705011495265, 53.50051614449767357, 8.000000000000001776 ) ) ;
#16594=CARTESIAN_POINT ( 'NONE',  ( 56.66441430157296821, 62.09948385550239891, 2.141517661632100111 ) ) ;
#16601=CARTESIAN_POINT ( 'NONE',  ( 43.34962307344081012, 60.89948385550241028, 2.184720259617164650 ) ) ;
#16603=CARTESIAN_POINT ( 'NONE',  ( 56.79116909180255135, 53.79948385550241596, -4.963592699179005585 ) ) ;
#16605=CARTESIAN_POINT ( 'NONE',  ( 45.90387839640208512, 56.30051614449765651, -5.676469297603124353 ) ) ;
#16619=CARTESIAN_POINT ( 'NONE',  ( 45.86712807150323812, 65.29948385550241596, -5.649768623646098220 ) ) ;
#16625=CARTESIAN_POINT ( 'NONE',  ( 48.07319477248768180, 58.59948385550239891, 6.007379884777225953 ) ) ;
#16628=CARTESIAN_POINT ( 'NONE',  ( 57.60143344285435774, 55.10051614449765367, 2.493737253992045044 ) ) ;
#16630=CARTESIAN_POINT ( 'NONE',  ( 48.07319477248762496, 56.40051614449765793, -6.007379884777208190 ) ) ;
#16640=CARTESIAN_POINT ( 'NONE',  ( 56.66441430157296821, 64.09948385550239891, 2.141517661632100111 ) ) ;
#16650=CARTESIAN_POINT ( 'NONE',  ( 56.81924384183006538, 62.80051614449766362, -4.924951120819380357 ) ) ;
#16653=CARTESIAN_POINT ( 'NONE',  ( 55.96859303347804371, 58.19948385550241454, 4.306917132069425946 ) ) ;
#16656=CARTESIAN_POINT ( 'NONE',  ( 45.90387839640208512, 54.30051614449765651, -5.676469297603124353 ) ) ;
#16667=CARTESIAN_POINT ( 'NONE',  ( 54.13287192849676188, 48.29948385550240175, 5.649768623646098220 ) ) ;
#16672=CARTESIAN_POINT ( 'NONE',  ( 54.09612160359792199, 57.30051614449765651, 5.676469297603124353 ) ) ;
#16676=CARTESIAN_POINT ( 'NONE',  ( 46.45491332379576477, 57.70051614449766930, 4.840751629271188961 ) ) ;
#16680=CARTESIAN_POINT ( 'NONE',  ( 46.45491332379572924, 59.29948385550240886, -4.840751629271157874 ) ) ;
#16682=CARTESIAN_POINT ( 'NONE',  ( 52.57664461997821093, 55.40051614449767214, 8.007379884777206414 ) ) ;
#16693=CARTESIAN_POINT ( 'NONE',  ( 47.74827507625477807, 64.59948385550239891, 7.007379884777229506 ) ) ;
#16697=CARTESIAN_POINT ( 'NONE',  ( 45.86712807150323812, 61.29948385550240886, -5.649768623646098220 ) ) ;
#16699=CARTESIAN_POINT ( 'NONE',  ( 52.57664461997811856, 57.59948385550240602, -8.007379884777229506 ) ) ;
#16701=CARTESIAN_POINT ( 'NONE',  ( 45.86712807150329496, 55.70051614449766220, 5.649768623646139964 ) ) ;
#16707=CARTESIAN_POINT ( 'NONE',  ( 47.70284917648459810, 49.60051614449765367, 6.992620115222797139 ) ) ;
#16709=CARTESIAN_POINT ( 'NONE',  ( 56.66441430157296821, 64.09948385550239891, 2.141517661632100111 ) ) ;
#16715=CARTESIAN_POINT ( 'NONE',  ( 44.91013252490152752, 64.79948385550240175, 3.727524721679198461 ) ) ;
#16719=CARTESIAN_POINT ( 'NONE',  ( 47.37792948025170858, 51.60051614449766788, 7.992620115222797139 ) ) ;
#16721=CARTESIAN_POINT ( 'NONE',  ( 51.92680522751238925, 57.40051614449767214, 6.007379884777208190 ) ) ;
#16728=CARTESIAN_POINT ( 'NONE',  ( 54.42198456365324688, 44.83981687677464834, -4.999999999999773515 ) ) ;
#16735=CARTESIAN_POINT ( 'NONE',  ( 49.97728705011488159, 53.49948385550240459, -7.000000000000000888 ) ) ;
#16740=CARTESIAN_POINT ( 'NONE',  ( 45.27934281921075410, 49.29948385550240886, -6.458785618021043895 ) ) ;
#16742=CARTESIAN_POINT ( 'NONE',  ( 49.97728705011488159, 57.49948385550241170, -7.000000000000000888 ) ) ;
#16745=CARTESIAN_POINT ( 'NONE',  ( 45.86712807150329496, 55.70051614449766220, 5.649768623646139964 ) ) ;
#16747=CARTESIAN_POINT ( 'NONE',  ( 54.09612160359786515, 49.69948385550240744, -5.676469297603166098 ) ) ;
#16749=ORIENTED_EDGE ( 'NONE', *, *, #2942, .T. ) ;
#16754=CARTESIAN_POINT ( 'NONE',  ( 42.63976443033212860, 54.99948385550241170, 0.02388180880522514787 ) ) ;
#16759=CARTESIAN_POINT ( 'NONE',  ( 54.09612160359792199, 61.30051614449766362, 5.676469297603124353 ) ) ;
#16767=CARTESIAN_POINT ( 'NONE',  ( 46.49166364869456913, 58.30051614449765651, -4.867452303228181343 ) ) ;
#16771=CARTESIAN_POINT ( 'NONE',  ( 55.71335778527780747, 64.09948385550239891, 1.832500667257165983 ) ) ;
#16774=CARTESIAN_POINT ( 'NONE',  ( 42.38452918213190657, 51.90051614449765793, 2.450534656007115508 ) ) ;
#16790=CARTESIAN_POINT ( 'NONE',  ( 46.45491332379572924, 47.29948385550241596, -4.840751629271157874 ) ) ;
#16792=CARTESIAN_POINT ( 'NONE',  ( 54.68390685589033495, 61.69948385550240744, -6.485486291978119766 ) ) ;
#16793=CARTESIAN_POINT ( 'NONE',  ( 57.36023556966787851, 57.00051614449766646, 0.02388180880515038476 ) ) ;
#16801=CARTESIAN_POINT ( 'NONE',  ( 43.33558569842706021, 47.90051614449765793, 2.141517661632167169 ) ) ;
#16809=CARTESIAN_POINT ( 'NONE',  ( 48.02776887271750184, 45.60051614449765367, 5.992620115222795363 ) ) ;
#16813=CARTESIAN_POINT ( 'NONE',  ( 56.79116909180259398, 61.20051614449766220, 4.963592699178938972 ) ) ;
#16814=CARTESIAN_POINT ( 'NONE',  ( 44.91013252490150620, 54.20051614449766220, -3.727524721679154940 ) ) ;
#16821=CARTESIAN_POINT ( 'NONE',  ( 54.89903213687075834, 44.74560054925188268, -5.000000000000007105 ) ) ;
#16828=CARTESIAN_POINT ( 'NONE',  ( 54.09612160359786515, 51.69948385550240744, -5.676469297603166098 ) ) ;
#16834=CARTESIAN_POINT ( 'NONE',  ( 43.18075615816989199, 49.19948385550240744, -4.924951120819313743 ) ) ;
#16838=CARTESIAN_POINT ( 'NONE',  ( 55.08986747509847248, 45.79948385550240886, -3.727524721679197572 ) ) ;
#16841=CARTESIAN_POINT ( 'NONE',  ( 56.66441430157294690, 60.90051614449766504, -2.141517661632166281 ) ) ;
#16845=CARTESIAN_POINT ( 'NONE',  ( 52.29715082351547295, 50.39948385550240317, 6.992620115222774047 ) ) ;
#16853=CARTESIAN_POINT ( 'NONE',  ( 52.29715082351547295, 50.39948385550240317, 6.992620115222774047 ) ) ;
#16858=EDGE_CURVE ( 'NONE', #14352, #17307, #493, .T. ) ;
#16865=CARTESIAN_POINT ( 'NONE',  ( 48.07319477248762496, 56.40051614449765793, -6.007379884777208190 ) ) ;
#16870=CARTESIAN_POINT ( 'NONE',  ( 54.72065718078918906, 58.70051614449765509, -6.458785618021089192 ) ) ;
#16886=CARTESIAN_POINT ( 'NONE',  ( 49.97728705011488159, 63.49948385550241170, -7.000000000000000888 ) ) ;
#16890=CARTESIAN_POINT ( 'NONE',  ( 54.09612160359786515, 61.69948385550240744, -5.676469297603166098 ) ) ;
#16892=CARTESIAN_POINT ( 'NONE',  ( 58.41169779390614281, 59.99948385550241170, -0.02388180880523160798 ) ) ;
#16894=CARTESIAN_POINT ( 'NONE',  ( 55.96859303347802239, 60.80051614449764941, -4.306917132069484566 ) ) ;
#16903=CARTESIAN_POINT ( 'NONE',  ( 43.34962307344078880, 46.10051614449766078, -2.184720259617096705 ) ) ;
#16905=CARTESIAN_POINT ( 'NONE',  ( 49.97728705011488159, 61.49948385550240459, -7.000000000000000888 ) ) ;
#16910=CARTESIAN_POINT ( 'NONE',  ( 53.50833635130540955, 61.69948385550240744, -4.867452303228209765 ) ) ;
#16914=CARTESIAN_POINT ( 'NONE',  ( 56.79116909180259398, 59.20051614449766220, 4.963592699178938972 ) ) ;
#16915=CARTESIAN_POINT ( 'NONE',  ( 48.07319477248762496, 62.40051614449765793, -6.007379884777208190 ) ) ;
#16927=CARTESIAN_POINT ( 'NONE',  ( 45.90387839640214196, 52.69948385550240033, 5.676469297603166098 ) ) ;
#16931=CARTESIAN_POINT ( 'NONE',  ( 57.61547081786812896, 52.09948385550241312, 2.450534656007040901 ) ) ;
#16934=CARTESIAN_POINT ( 'NONE',  ( 44.05948171654949874, 64.79948385550240175, 4.345558710429105354 ) ) ;
#16939=CARTESIAN_POINT ( 'NONE',  ( 44.03140696652198471, 63.80051614449765651, 4.306917132069485454 ) ) ;
#16942=CARTESIAN_POINT ( 'NONE',  ( 44.05948171654949874, 60.79948385550240886, 4.345558710429105354 ) ) ;
#16951=CARTESIAN_POINT ( 'NONE',  ( 42.63976443033212860, 52.99948385550240459, 0.02388180880522514787 ) ) ;
#16963=CARTESIAN_POINT ( 'NONE',  ( 54.09612160359786515, 45.69948385550240744, -5.676469297603166098 ) ) ;
#16966=CARTESIAN_POINT ( 'NONE',  ( 51.92680522751238925, 61.40051614449765793, 6.007379884777208190 ) ) ;
#16973=CARTESIAN_POINT ( 'NONE',  ( 43.20883090819742023, 60.20051614449766220, -4.963592699178938972 ) ) ;
#16992=CARTESIAN_POINT ( 'NONE',  ( 47.74827507625478518, 64.59948385550239891, 7.007379884777227730 ) ) ;
#16994=CARTESIAN_POINT ( 'NONE',  ( 50.02271294988513972, 58.49948385550241170, 8.000000000000001776 ) ) ;
#16995=CARTESIAN_POINT ( 'NONE',  ( 45.90387839640208512, 60.30051614449766362, -5.676469297603124353 ) ) ;
#17003=CARTESIAN_POINT ( 'NONE',  ( 51.03999344061968912, 45.00000000000002132, -7.500000000000003553 ) ) ;
#17008=EDGE_CURVE ( 'NONE', #2212, #12707, #5402, .T. ) ;
#17009=CARTESIAN_POINT ( 'NONE',  ( 44.28664221472220675, 61.09948385550241312, -1.832500667257165317 ) ) ;
#17012=CARTESIAN_POINT ( 'NONE',  ( 54.09612160359786515, 45.69948385550240744, -5.676469297603166098 ) ) ;
#17015=CARTESIAN_POINT ( 'NONE',  ( 56.81924384183006538, 62.80051614449766362, -4.924951120819380357 ) ) ;
#17017=CARTESIAN_POINT ( 'NONE',  ( 55.08986747509849380, 59.20051614449766220, 3.727524721679155384 ) ) ;
#17027=CARTESIAN_POINT ( 'NONE',  ( 44.03140696652193498, 51.19948385550240033, -4.306917132069424170 ) ) ;
#17031=CARTESIAN_POINT ( 'NONE',  ( 43.20883090819745576, 50.79948385550240175, 4.963592699179006473 ) ) ;
#17033=CARTESIAN_POINT ( 'NONE',  ( 53.50833635130540955, 45.69948385550240033, -4.867452303228209765 ) ) ;
#17036=CARTESIAN_POINT ( 'NONE',  ( 54.13287192849671214, 60.70051614449766220, -5.649768623646139964 ) ) ;
#17037=CARTESIAN_POINT ( 'NONE',  ( 44.03140696652192787, 59.19948385550238612, -4.306917132069425058 ) ) ;
#17045=CARTESIAN_POINT ( 'NONE',  ( 55.94051828345050836, 51.79948385550240175, -4.345558710429104465 ) ) ;
#17056=CARTESIAN_POINT ( 'NONE',  ( 47.70284917648453415, 47.39948385550238896, -6.992620115222774047 ) ) ;
#17059=CARTESIAN_POINT ( 'NONE',  ( 53.50833635130544508, 61.30051614449766362, 4.867452303228181343 ) ) ;
#17061=( NAMED_UNIT ( * ) PLANE_ANGLE_UNIT ( ) SI_UNIT ( $, .RADIAN. ) );
#17064=CARTESIAN_POINT ( 'NONE',  ( 43.18075615816994173, 59.80051614449766362, 4.924951120819380357 ) ) ;
#17082=CARTESIAN_POINT ( 'NONE',  ( 50.02271294988511841, 46.49948385550240459, 6.000000000000000888 ) ) ;
#17084=CARTESIAN_POINT ( 'NONE',  ( 50.02271294988513972, 60.49948385550240459, 8.000000000000001776 ) ) ;
#17085=CARTESIAN_POINT ( 'NONE',  ( 52.25172492374527877, 63.40051614449765793, 7.007379884777203749 ) ) ;
#17093=CARTESIAN_POINT ( 'NONE',  ( 52.25172492374528588, 45.40051614449766504, 7.007379884777204637 ) ) ;
#17104=CARTESIAN_POINT ( 'NONE',  ( 50.02271294988505446, 62.50051614449767357, -8.000000000000001776 ) ) ;
#17106=CARTESIAN_POINT ( 'NONE',  ( 44.91013252490150620, 62.20051614449766220, -3.727524721679154940 ) ) ;
#17119=CARTESIAN_POINT ( 'NONE',  ( 52.29715082351547295, 60.39948385550240317, 6.992620115222774047 ) ) ;
#17123=CARTESIAN_POINT ( 'NONE',  ( 43.20883090819745576, 52.79948385550240175, 4.963592699179006473 ) ) ;
#17126=CARTESIAN_POINT ( 'NONE',  ( 54.13287192849676188, 62.29948385550240886, 5.649768623646098220 ) ) ;
#17129=CARTESIAN_POINT ( 'NONE',  ( 52.29715082351538769, 60.60051614449764656, -6.992620115222796251 ) ) ;
#17130=CARTESIAN_POINT ( 'NONE',  ( 53.54508667620428497, 62.29948385550241596, 4.840751629271157874 ) ) ;
#17131=CARTESIAN_POINT ( 'NONE',  ( 55.94051828345050836, 57.79948385550238754, -4.345558710429104465 ) ) ;
#17140=CARTESIAN_POINT ( 'NONE',  ( 55.96859303347804371, 54.19948385550240033, 4.306917132069425946 ) ) ;
#17148=CARTESIAN_POINT ( 'NONE',  ( 54.13287192849676188, 46.29948385550240886, 5.649768623646098220 ) ) ;
#17150=CARTESIAN_POINT ( 'NONE',  ( 51.92680522751238925, 63.40051614449765083, 6.007379884777208190 ) ) ;
#17155=CARTESIAN_POINT ( 'NONE',  ( 54.68390685589039890, 61.30051614449766362, 6.485486291978072693 ) ) ;
#17174=CARTESIAN_POINT ( 'NONE',  ( 55.71335778527780747, 46.09948385550240602, 1.832500667257165983 ) ) ;
#17177=CARTESIAN_POINT ( 'NONE',  ( 45.90387839640214196, 48.69948385550240744, 5.676469297603166098 ) ) ;
#17178=CARTESIAN_POINT ( 'NONE',  ( 43.34962307344078880, 62.10051614449766078, -2.184720259617096705 ) ) ;
#17188=CARTESIAN_POINT ( 'NONE',  ( 47.70284917648459810, 53.60051614449766078, 6.992620115222797139 ) ) ;
#17191=CARTESIAN_POINT ( 'NONE',  ( 49.99999999999997158, 45.00000000000001421, -7.499999999999998224 ) ) ;
#17199=CARTESIAN_POINT ( 'NONE',  ( 57.36023556966787851, 45.99948385550238328, -0.02388180880522424582 ) ) ;
#17201=CARTESIAN_POINT ( 'NONE',  ( 49.97728705011495265, 61.50051614449766646, 8.000000000000001776 ) ) ;
#17202=CARTESIAN_POINT ( 'NONE',  ( 50.02271294988506156, 62.50051614449767357, -6.000000000000000888 ) ) ;
#17217=CARTESIAN_POINT ( 'NONE',  ( 45.86712807150323812, 59.29948385550240175, -5.649768623646098220 ) ) ;
#17221=CARTESIAN_POINT ( 'NONE',  ( 42.38452918213188525, 55.09948385550241312, -2.450534656007040013 ) ) ;
#17223=CARTESIAN_POINT ( 'NONE',  ( 52.25172492374522903, 63.59948385550237759, -7.007379884777225953 ) ) ;
#17226=CARTESIAN_POINT ( 'NONE',  ( 43.34962307344078880, 60.10051614449766078, -2.184720259617096705 ) ) ;
#17228=CARTESIAN_POINT ( 'NONE',  ( 44.88205777487398507, 61.19948385550241454, -3.688883143319540814 ) ) ;
#17229=CARTESIAN_POINT ( 'NONE',  ( 52.25172492374522903, 59.59948385550240602, -7.007379884777225953 ) ) ;
#17237=CARTESIAN_POINT ( 'NONE',  ( 45.86712807150323812, 61.29948385550240886, -5.649768623646098220 ) ) ;
#17250=CARTESIAN_POINT ( 'NONE',  ( 55.96859303347804371, 48.19948385550240033, 4.306917132069425946 ) ) ;
#17253=CARTESIAN_POINT ( 'NONE',  ( 50.02271294988506156, 64.50051614449766646, -6.000000000000000888 ) ) ;
#17278=CARTESIAN_POINT ( 'NONE',  ( 43.69122665457040000, 48.99948385550241170, 0.02388180880521036456 ) ) ;
#17280=CARTESIAN_POINT ( 'NONE',  ( 42.63976443033212860, 48.99948385550240459, 0.02388180880522514787 ) ) ;
#17281=CARTESIAN_POINT ( 'NONE',  ( 47.74827507625469281, 58.40051614449766504, -7.007379884777203749 ) ) ;
#17292=CARTESIAN_POINT ( 'NONE',  ( 56.66441430157294690, 50.90051614449766504, -2.141517661632166281 ) ) ;
#17300=CARTESIAN_POINT ( 'NONE',  ( 55.94051828345050836, 45.79948385550240886, -4.345558710429104465 ) ) ;
#17302=CARTESIAN_POINT ( 'NONE',  ( 41.58830220609386430, 48.99948385550241170, 0.02388180880523263147 ) ) ;
#17304=CARTESIAN_POINT ( 'NONE',  ( 56.30877334542961421, 59.00051614449766646, 0.02388180880515774693 ) ) ;
#17307=VERTEX_POINT ( 'NONE', #11361 ) ;
#17317=CARTESIAN_POINT ( 'NONE',  ( 50.02271294988512551, 58.49948385550241170, 7.000000000000000888 ) ) ;
#17321=CARTESIAN_POINT ( 'NONE',  ( 47.37792948025162332, 55.39948385550240317, -7.992620115222770494 ) ) ;
#17324=CARTESIAN_POINT ( 'NONE',  ( 48.07319477248768180, 52.59948385550240602, 6.007379884777225953 ) ) ;
#17328=CARTESIAN_POINT ( 'NONE',  ( 52.57664461997821093, 45.40051614449765793, 8.007379884777206414 ) ) ;
#17329=CARTESIAN_POINT ( 'NONE',  ( 46.45491332379572924, 61.29948385550240886, -4.840751629271157874 ) ) ;
#17335=CARTESIAN_POINT ( 'NONE',  ( 56.66441430157296821, 60.09948385550240602, 2.141517661632100111 ) ) ;
#17342=CARTESIAN_POINT ( 'NONE',  ( 52.29715082351547295, 58.39948385550238896, 6.992620115222774047 ) ) ;
#17349=CARTESIAN_POINT ( 'NONE',  ( 52.25172492374522903, 53.59948385550241312, -7.007379884777225953 ) ) ;
#17351=CARTESIAN_POINT ( 'NONE',  ( 51.97223112728249816, 58.60051614449766788, -5.992620115222793586 ) ) ;
#17371=CARTESIAN_POINT ( 'NONE',  ( 48.02776887271745210, 63.39948385550238896, -5.992620115222778487 ) ) ;
#17374=CARTESIAN_POINT ( 'NONE',  ( 55.11794222512601493, 52.19948385550240744, 3.688883143319541702 ) ) ;
#17376=CARTESIAN_POINT ( 'NONE',  ( 43.34962307344081012, 46.89948385550240317, 2.184720259617164650 ) ) ;
#17377=CARTESIAN_POINT ( 'NONE',  ( 56.79116909180259398, 47.20051614449766220, 4.963592699178938972 ) ) ;
#17385=CARTESIAN_POINT ( 'NONE',  ( 42.63976443033212149, 54.00051614449765935, -0.02388180880514948964 ) ) ;
#17394=CARTESIAN_POINT ( 'NONE',  ( 54.09612160359786515, 51.69948385550240744, -5.676469297603166098 ) ) ;
#17397=CARTESIAN_POINT ( 'NONE',  ( 42.38452918213188525, 49.09948385550241312, -2.450534656007040013 ) ) ;
#17400=CARTESIAN_POINT ( 'NONE',  ( 45.86712807150329496, 47.70051614449766220, 5.649768623646139964 ) ) ;
#17410=CARTESIAN_POINT ( 'NONE',  ( 45.90387839640214196, 56.69948385550240744, 5.676469297603166098 ) ) ;
#17414=CARTESIAN_POINT ( 'NONE',  ( 42.39856655714566358, 58.89948385550241028, 2.493737253992119207 ) ) ;
#17417=CARTESIAN_POINT ( 'NONE',  ( 44.30067958973596376, 52.89948385550241028, 1.875703265242204099 ) ) ;
#17420=CARTESIAN_POINT ( 'NONE',  ( 57.61547081786810764, 48.90051614449766504, -2.450534656007114176 ) ) ;
#17421=CARTESIAN_POINT ( 'NONE',  ( 44.30067958973596376, 64.89948385550239607, 1.875703265242204099 ) ) ;
#17431=CARTESIAN_POINT ( 'NONE',  ( 54.09612160359786515, 57.69948385550240744, -5.676469297603166098 ) ) ;
#17443=CARTESIAN_POINT ( 'NONE',  ( 49.97728705011488159, 49.49948385550240459, -7.000000000000000888 ) ) ;
#17446=CARTESIAN_POINT ( 'NONE',  ( 55.96859303347802239, 46.80051614449767072, -4.306917132069484566 ) ) ;
#17467=CARTESIAN_POINT ( 'NONE',  ( 56.30877334542961421, 51.00051614449765935, 0.02388180880515774693 ) ) ;
#17471=CARTESIAN_POINT ( 'NONE',  ( 55.71335778527780747, 50.09948385550240602, 1.832500667257165983 ) ) ;
#17474=CARTESIAN_POINT ( 'NONE',  ( 52.29715082351547295, 46.39948385550240317, 6.992620115222774047 ) ) ;
#17475=CARTESIAN_POINT ( 'NONE',  ( 56.79116909180259398, 45.20051614449766220, 4.963592699178938972 ) ) ;
#17485=CARTESIAN_POINT ( 'NONE',  ( 55.94051828345054389, 53.20051614449766220, 4.345558710429044957 ) ) ;
#17491=CARTESIAN_POINT ( 'NONE',  ( 52.29715082351547295, 52.39948385550241738, 6.992620115222774047 ) ) ;
#17493=CARTESIAN_POINT ( 'NONE',  ( 49.97728705011486738, 45.49948385550240459, -8.000000000000001776 ) ) ;
#17495=CARTESIAN_POINT ( 'NONE',  ( 42.63976443033212860, 48.00051614449766646, -0.02388180880514948964 ) ) ;
#17509=CARTESIAN_POINT ( 'NONE',  ( 55.96859303347805081, 60.19948385550240033, 4.306917132069425058 ) ) ;
#17514=CARTESIAN_POINT ( 'NONE',  ( 49.97728705011486738, 61.49948385550241170, -8.000000000000001776 ) ) ;
#17516=CARTESIAN_POINT ( 'NONE',  ( 53.50833635130540955, 49.69948385550240744, -4.867452303228209765 ) ) ;
#17520=CARTESIAN_POINT ( 'NONE',  ( 50.02271294988505446, 64.50051614449765225, -7.000000000000000888 ) ) ;
#17521=CARTESIAN_POINT ( 'NONE',  ( 46.45491332379576477, 49.70051614449766220, 4.840751629271188961 ) ) ;
#17530=CARTESIAN_POINT ( 'NONE',  ( 44.05948171654949874, 60.79948385550240886, 4.345558710429105354 ) ) ;
#17541=CARTESIAN_POINT ( 'NONE',  ( 52.29715082351547295, 50.39948385550240317, 6.992620115222774047 ) ) ;
#17543=CARTESIAN_POINT ( 'NONE',  ( 55.96859303347802239, 50.80051614449766362, -4.306917132069484566 ) ) ;
#17568=CARTESIAN_POINT ( 'NONE',  ( 44.28664221472221385, 51.90051614449765793, 1.832500667257213722 ) ) ;
#17574=CARTESIAN_POINT ( 'NONE',  ( 55.08986747509847248, 53.79948385550241596, -3.727524721679197572 ) ) ;
#17578=CARTESIAN_POINT ( 'NONE',  ( 47.74827507625478518, 48.59948385550239180, 7.007379884777227730 ) ) ;
#17579=CARTESIAN_POINT ( 'NONE',  ( 49.97728705011495265, 47.50051614449765935, 8.000000000000001776 ) ) ;
#17591=CARTESIAN_POINT ( 'NONE',  ( 43.33558569842706021, 53.90051614449765793, 2.141517661632167169 ) ) ;
#17597=CARTESIAN_POINT ( 'NONE',  ( 55.96859303347804371, 54.19948385550240033, 4.306917132069425946 ) ) ;
#17599=CARTESIAN_POINT ( 'NONE',  ( 56.79116909180255135, 49.79948385550240175, -4.963592699179005585 ) ) ;
#17600=CARTESIAN_POINT ( 'NONE',  ( 56.66441430157294690, 46.90051614449765793, -2.141517661632166281 ) ) ;
#17616=CARTESIAN_POINT ( 'NONE',  ( 42.39856655714566358, 60.89948385550241028, 2.493737253992119207 ) ) ;
#17620=CARTESIAN_POINT ( 'NONE',  ( 51.92680522751233951, 53.59948385550240602, -6.007379884777223289 ) ) ;
#17624=CARTESIAN_POINT ( 'NONE',  ( 52.62207051974829852, 44.60051614449766078, -7.992620115222797139 ) ) ;
#17625=CARTESIAN_POINT ( 'NONE',  ( 44.30067958973594955, 46.10051614449766078, -1.875703265242155693 ) ) ;
#17634=CARTESIAN_POINT ( 'NONE',  ( 47.70284917648453415, 55.39948385550238896, -6.992620115222774047 ) ) ;
#17644=CARTESIAN_POINT ( 'NONE',  ( 54.13287192849676188, 52.29948385550240886, 5.649768623646098220 ) ) ;
#17646=CARTESIAN_POINT ( 'NONE',  ( 45.90387839640208512, 46.30051614449766362, -5.676469297603124353 ) ) ;
#17654=ORIENTED_EDGE ( 'NONE', *, *, #16858, .T. ) ;
#17660=CARTESIAN_POINT ( 'NONE',  ( 44.28664221472221385, 49.90051614449766504, 1.832500667257213722 ) ) ;
#17662=CARTESIAN_POINT ( 'NONE',  ( 44.88205777487398507, 49.19948385550240744, -3.688883143319540814 ) ) ;
#17664=CARTESIAN_POINT ( 'NONE',  ( 47.74827507625478518, 50.59948385550238470, 7.007379884777227730 ) ) ;
#17665=CARTESIAN_POINT ( 'NONE',  ( 50.02271294988505446, 46.50051614449766646, -8.000000000000001776 ) ) ;
#17686=CARTESIAN_POINT ( 'NONE',  ( 47.74827507625478518, 54.59948385550239180, 7.007379884777227730 ) ) ;
#17688=CARTESIAN_POINT ( 'NONE',  ( 57.61547081786812896, 48.09948385550240602, 2.450534656007040901 ) ) ;
#17690=CARTESIAN_POINT ( 'NONE',  ( 43.33558569842706021, 49.90051614449766504, 2.141517661632167169 ) ) ;
#17706=CARTESIAN_POINT ( 'NONE',  ( 57.61547081786812896, 62.09948385550240602, 2.450534656007040901 ) ) ;
#17708=CARTESIAN_POINT ( 'NONE',  ( 55.69932041026404335, 51.89948385550241028, -1.875703265242203432 ) ) ;
#17711=CARTESIAN_POINT ( 'NONE',  ( 45.27934281921082516, 45.70051614449766220, 6.458785618021089192 ) ) ;
#17713=CARTESIAN_POINT ( 'NONE',  ( 48.07319477248762496, 48.40051614449766504, -6.007379884777208190 ) ) ;
#17720=ADVANCED_FACE ( 'NONE', ( #3709 ), #8557, .T. ) ;
#17733=CARTESIAN_POINT ( 'NONE',  ( 57.36023556966787851, 49.99948385550238328, -0.02388180880522424582 ) ) ;
#17735=CARTESIAN_POINT ( 'NONE',  ( 43.34962307344078880, 48.10051614449766078, -2.184720259617096705 ) ) ;
#17744=CARTESIAN_POINT ( 'NONE',  ( 43.34962307344081012, 46.89948385550240317, 2.184720259617164650 ) ) ;
#17755=CARTESIAN_POINT ( 'NONE',  ( 55.69932041026405045, 47.10051614449766078, 1.875703265242156359 ) ) ;
#17758=CARTESIAN_POINT ( 'NONE',  ( 44.88205777487398507, 59.19948385550240744, -3.688883143319540814 ) ) ;
#17760=CARTESIAN_POINT ( 'NONE',  ( 44.03140696652192787, 55.19948385550238612, -4.306917132069425058 ) ) ;
#17761=CARTESIAN_POINT ( 'NONE',  ( 57.61547081786810764, 44.90051614449765793, -2.450534656007114176 ) ) ;
#17778=CARTESIAN_POINT ( 'NONE',  ( 54.09612160359786515, 53.69948385550240744, -5.676469297603166098 ) ) ;
#17780=CARTESIAN_POINT ( 'NONE',  ( 52.57664461997811856, 51.59948385550240602, -8.007379884777229506 ) ) ;
#17783=CARTESIAN_POINT ( 'NONE',  ( 55.96859303347802239, 50.80051614449766362, -4.306917132069484566 ) ) ;
#17802=CARTESIAN_POINT ( 'NONE',  ( 50.02271294988513972, 62.49948385550240459, 8.000000000000001776 ) ) ;
#17805=CARTESIAN_POINT ( 'NONE',  ( 53.50833635130540955, 59.69948385550240744, -4.867452303228209765 ) ) ;
#17809=CARTESIAN_POINT ( 'NONE',  ( 54.72065718078918906, 52.70051614449766220, -6.458785618021089192 ) ) ;
#17811=CARTESIAN_POINT ( 'NONE',  ( 51.97223112728249816, 50.60051614449765367, -5.992620115222793586 ) ) ;
#17821=CARTESIAN_POINT ( 'NONE',  ( 54.09612160359786515, 61.69948385550240744, -5.676469297603166098 ) ) ;
#17825=CARTESIAN_POINT ( 'NONE',  ( 52.29715082351547295, 48.39948385550240317, 6.992620115222774047 ) ) ;
#17830=CARTESIAN_POINT ( 'NONE',  ( 43.33558569842703179, 59.09948385550240602, -2.141517661632099223 ) ) ;
#17832=CARTESIAN_POINT ( 'NONE',  ( 47.70284917648459100, 45.60051614449765367, 6.992620115222796251 ) ) ;
#17844=CARTESIAN_POINT ( 'NONE',  ( 45.27934281921075410, 65.29948385550241596, -6.458785618021043895 ) ) ;
#17856=CARTESIAN_POINT ( 'NONE',  ( 48.07319477248762496, 46.40051614449765793, -6.007379884777208190 ) ) ;
#17860=CARTESIAN_POINT ( 'NONE',  ( 53.54508667620428497, 56.29948385550240886, 4.840751629271157874 ) ) ;
#17862=CARTESIAN_POINT ( 'NONE',  ( 56.65037692655918988, 51.89948385550241028, -2.184720259617163762 ) ) ;
#17864=CARTESIAN_POINT ( 'NONE',  ( 56.81924384183006538, 56.80051614449764941, -4.924951120819380357 ) ) ;
#17881=CARTESIAN_POINT ( 'NONE',  ( 44.05948171654949874, 58.79948385550240886, 4.345558710429105354 ) ) ;
#17884=CARTESIAN_POINT ( 'NONE',  ( 45.27934281921075410, 53.29948385550240886, -6.458785618021043895 ) ) ;
#17886=CARTESIAN_POINT ( 'NONE',  ( 52.29715082351538769, 56.60051614449766788, -6.992620115222796251 ) ) ;
#17905=CARTESIAN_POINT ( 'NONE',  ( 53.54508667620428497, 58.29948385550240886, 4.840751629271157874 ) ) ;
#17909=CARTESIAN_POINT ( 'NONE',  ( 49.97728705011495265, 53.50051614449767357, 8.000000000000001776 ) ) ;
#17910=CARTESIAN_POINT ( 'NONE',  ( 48.02776887271750184, 47.60051614449766078, 5.992620115222795363 ) ) ;
#17915=EDGE_CURVE ( 'NONE', #7311, #14352, #7827, .T. ) ;
#17918=ORIENTED_EDGE ( 'NONE', *, *, #18385, .T. ) ;
#17920=CARTESIAN_POINT ( 'NONE',  ( 56.65037692655918988, 63.89948385550239607, -2.184720259617163762 ) ) ;
#17925=CARTESIAN_POINT ( 'NONE',  ( 45.90387839640214196, 46.69948385550240744, 5.676469297603166098 ) ) ;
#17931=CARTESIAN_POINT ( 'NONE',  ( 52.57664461997811856, 49.59948385550241312, -8.007379884777229506 ) ) ;
#17932=CARTESIAN_POINT ( 'NONE',  ( 53.93078149122418807, 45.00000000000000000, -5.235029531081472953 ) ) ;
#17933=CARTESIAN_POINT ( 'NONE',  ( 52.29715082351547295, 60.39948385550239607, 6.992620115222774047 ) ) ;
#17936=CARTESIAN_POINT ( 'NONE',  ( 55.96859303347802239, 52.80051614449764941, -4.306917132069484566 ) ) ;
#17947=CARTESIAN_POINT ( 'NONE',  ( 43.33558569842703179, 47.09948385550240602, -2.141517661632099223 ) ) ;
#17952=CARTESIAN_POINT ( 'NONE',  ( 47.74827507625470702, 56.40051614449766504, -7.007379884777204637 ) ) ;
#17959=CARTESIAN_POINT ( 'NONE',  ( 51.97223112728249816, 56.60051614449765367, -5.992620115222793586 ) ) ;
#17962=CARTESIAN_POINT ( 'NONE',  ( 43.69122665457040000, 54.99948385550239749, 0.02388180880521036456 ) ) ;
#17964=CARTESIAN_POINT ( 'NONE',  ( 44.03140696652192787, 51.19948385550238612, -4.306917132069425058 ) ) ;
#17965=CARTESIAN_POINT ( 'NONE',  ( 42.38452918213190657, 55.90051614449766504, 2.450534656007115508 ) ) ;
#17977=CARTESIAN_POINT ( 'NONE',  ( 47.70284917648453415, 63.39948385550239607, -6.992620115222774047 ) ) ;
#17981=CARTESIAN_POINT ( 'NONE',  ( 49.97728705011488159, 57.49948385550241170, -7.000000000000000888 ) ) ;
#17983=CARTESIAN_POINT ( 'NONE',  ( 43.20883090819745576, 52.79948385550240175, 4.963592699179006473 ) ) ;
#17985=CARTESIAN_POINT ( 'NONE',  ( 54.09612160359792199, 57.30051614449765651, 5.676469297603124353 ) ) ;
#17994=CARTESIAN_POINT ( 'NONE',  ( 52.29715082351547295, 62.39948385550239607, 6.992620115222774047 ) ) ;
#18000=CARTESIAN_POINT ( 'NONE',  ( 55.11794222512601493, 56.19948385550240744, 3.688883143319541702 ) ) ;
#18004=CARTESIAN_POINT ( 'NONE',  ( 56.81924384183006538, 54.80051614449764941, -4.924951120819380357 ) ) ;
#18006=CARTESIAN_POINT ( 'NONE',  ( 44.91013252490150620, 58.20051614449766220, -3.727524721679154940 ) ) ;
#18013=CARTESIAN_POINT ( 'NONE',  ( 57.36023556966787851, 63.99948385550241881, -0.02388180880522424582 ) ) ;
#18018=CARTESIAN_POINT ( 'NONE',  ( 43.34962307344081012, 46.89948385550240317, 2.184720259617164650 ) ) ;
#18022=CARTESIAN_POINT ( 'NONE',  ( 43.20883090819742023, 64.20051614449766930, -4.963592699178938972 ) ) ;
#18023=CARTESIAN_POINT ( 'NONE',  ( 53.45216259278994642, 45.00000000000002132, -5.549029329376620190 ) ) ;
#18024=CARTESIAN_POINT ( 'NONE',  ( 42.63976443033212860, 60.99948385550238328, 0.02388180880522514787 ) ) ;
#18027=CARTESIAN_POINT ( 'NONE',  ( 56.65037692655921120, 53.10051614449766078, 2.184720259617097593 ) ) ;
#18037=CARTESIAN_POINT ( 'NONE',  ( 54.09612160359786515, 47.69948385550240744, -5.676469297603166098 ) ) ;
#18045=CARTESIAN_POINT ( 'NONE',  ( 57.36023556966787851, 59.00051614449765935, 0.02388180880515038476 ) ) ;
#18050=CARTESIAN_POINT ( 'NONE',  ( 46.49166364869456913, 52.30051614449766362, -4.867452303228181343 ) ) ;
#18054=CARTESIAN_POINT ( 'NONE',  ( 48.07319477248768180, 56.59948385550239891, 6.007379884777225953 ) ) ;
#18057=CARTESIAN_POINT ( 'NONE',  ( 54.72065718078918906, 54.70051614449765509, -6.458785618021089192 ) ) ;
#18070=CARTESIAN_POINT ( 'NONE',  ( 44.03140696652193498, 65.19948385550240744, -4.306917132069424170 ) ) ;
#18074=CARTESIAN_POINT ( 'NONE',  ( 44.03140696652192787, 57.19948385550238612, -4.306917132069425058 ) ) ;
#18077=CARTESIAN_POINT ( 'NONE',  ( 45.31609314410967926, 50.69948385550240744, 6.485486291978119766 ) ) ;
#18079=CARTESIAN_POINT ( 'NONE',  ( 54.09612160359792199, 53.30051614449766362, 5.676469297603124353 ) ) ;
#18092=CARTESIAN_POINT ( 'NONE',  ( 47.74827507625478518, 62.59948385550240602, 7.007379884777227730 ) ) ;
#18098=CARTESIAN_POINT ( 'NONE',  ( 53.50833635130540955, 55.69948385550240744, -4.867452303228209765 ) ) ;
#18101=CARTESIAN_POINT ( 'NONE',  ( 41.58830220609386430, 52.00051614449766646, -0.02388180880514929535 ) ) ;
#18103=CARTESIAN_POINT ( 'NONE',  ( 51.97223112728249816, 52.60051614449765367, -5.992620115222793586 ) ) ;
#18105=CARTESIAN_POINT ( 'NONE',  ( 62.49999999999998579, 5.000000000000018652, -5.000000000000000000 ) ) ;
#18112=CARTESIAN_POINT ( 'NONE',  ( 55.96859303347804371, 64.19948385550239323, 4.306917132069425946 ) ) ;
#18117=CARTESIAN_POINT ( 'NONE',  ( 54.13287192849676188, 46.29948385550240886, 5.649768623646098220 ) ) ;
#18122=CARTESIAN_POINT ( 'NONE',  ( 54.68390685589039890, 63.30051614449767072, 6.485486291978072693 ) ) ;
#18124=CARTESIAN_POINT ( 'NONE',  ( 54.09612160359786515, 57.69948385550240744, -5.676469297603166098 ) ) ;
#18127=CARTESIAN_POINT ( 'NONE',  ( 56.66441430157294690, 54.90051614449765793, -2.141517661632166281 ) ) ;
#18138=CARTESIAN_POINT ( 'NONE',  ( 47.74827507625478518, 46.59948385550239891, 7.007379884777227730 ) ) ;
#18143=CARTESIAN_POINT ( 'NONE',  ( 54.13287192849671214, 58.70051614449765509, -5.649768623646139964 ) ) ;
#18150=CARTESIAN_POINT ( 'NONE',  ( 55.71335778527780036, 52.90051614449766504, -1.832500667257213056 ) ) ;
#18153=CARTESIAN_POINT ( 'NONE',  ( 53.54508667620428497, 58.29948385550240886, 4.840751629271157874 ) ) ;
#18156=CARTESIAN_POINT ( 'NONE',  ( 56.81924384183006538, 54.80051614449764941, -4.924951120819380357 ) ) ;
#18172=CARTESIAN_POINT ( 'NONE',  ( 44.03140696652193498, 61.19948385550240033, -4.306917132069424170 ) ) ;
#18178=CARTESIAN_POINT ( 'NONE',  ( 44.05948171654949874, 56.79948385550240886, 4.345558710429105354 ) ) ;
#18180=CARTESIAN_POINT ( 'NONE',  ( 57.61547081786812896, 52.09948385550241312, 2.450534656007040901 ) ) ;
#18182=CARTESIAN_POINT ( 'NONE',  ( 57.36023556966787851, 55.00051614449765225, 0.02388180880515038476 ) ) ;
#18193=CARTESIAN_POINT ( 'NONE',  ( 52.25172492374528588, 49.40051614449766504, 7.007379884777204637 ) ) ;
#18194=CARTESIAN_POINT ( 'NONE',  ( 57.36023556966787851, 63.99948385550241881, -0.02388180880522424582 ) ) ;
#18200=CARTESIAN_POINT ( 'NONE',  ( 44.91013252490152752, 62.79948385550240175, 3.727524721679198461 ) ) ;
#18203=CARTESIAN_POINT ( 'NONE',  ( 41.58830220609386430, 56.00051614449765935, -0.02388180880514929535 ) ) ;
#18205=CARTESIAN_POINT ( 'NONE',  ( 55.08986747509849380, 53.20051614449766220, 3.727524721679155384 ) ) ;
#18220=CARTESIAN_POINT ( 'NONE',  ( 43.34962307344081012, 52.89948385550240317, 2.184720259617164650 ) ) ;
#18225=CARTESIAN_POINT ( 'NONE',  ( 41.58830220609386430, 48.99948385550241170, 0.02388180880523263147 ) ) ;
#18228=CARTESIAN_POINT ( 'NONE',  ( 42.63976443033212860, 54.99948385550241170, 0.02388180880522514787 ) ) ;
#18231=CARTESIAN_POINT ( 'NONE',  ( 55.96859303347802239, 54.80051614449764230, -4.306917132069484566 ) ) ;
#18239=CARTESIAN_POINT ( 'NONE',  ( 52.25172492374522903, 53.59948385550241312, -7.007379884777225953 ) ) ;
#18245=CARTESIAN_POINT ( 'NONE',  ( 47.74827507625470702, 62.40051614449765793, -7.007379884777204637 ) ) ;
#18249=CARTESIAN_POINT ( 'NONE',  ( 55.71335778527780036, 54.90051614449765793, -1.832500667257213056 ) ) ;
#18252=CARTESIAN_POINT ( 'NONE',  ( 46.49166364869460466, 64.69948385550240744, 4.867452303228209765 ) ) ;
#18254=CARTESIAN_POINT ( 'NONE',  ( 45.31609314410960820, 56.30051614449766362, -6.485486291978072693 ) ) ;
#18265=CARTESIAN_POINT ( 'NONE',  ( 57.36023556966787851, 63.99948385550241170, -0.02388180880522424582 ) ) ;
#18269=CARTESIAN_POINT ( 'NONE',  ( 47.70284917648453415, 55.39948385550238896, -6.992620115222774047 ) ) ;
#18272=CARTESIAN_POINT ( 'NONE',  ( 47.37792948025162332, 61.39948385550240317, -7.992620115222770494 ) ) ;
#18273=CARTESIAN_POINT ( 'NONE',  ( 55.94051828345053679, 55.20051614449766930, 4.345558710429044069 ) ) ;
#18282=CARTESIAN_POINT ( 'NONE',  ( 55.96859303347802239, 46.80051614449766362, -4.306917132069484566 ) ) ;
#18284=CARTESIAN_POINT ( 'NONE',  ( 54.09612160359786515, 63.69948385550240744, -5.676469297603166098 ) ) ;
#18290=CARTESIAN_POINT ( 'NONE',  ( 51.97223112728249816, 44.60051614449766078, -5.992620115222793586 ) ) ;
#18293=CARTESIAN_POINT ( 'NONE',  ( 49.97728705011495265, 59.50051614449765935, 8.000000000000001776 ) ) ;
#18294=CARTESIAN_POINT ( 'NONE',  ( 48.02776887271750184, 57.60051614449765367, 5.992620115222795363 ) ) ;
#18308=CARTESIAN_POINT ( 'NONE',  ( 50.02271294988512551, 54.49948385550240459, 7.000000000000000888 ) ) ;
#18313=CARTESIAN_POINT ( 'NONE',  ( 57.60143344285433642, 45.89948385550240317, -2.493737253992118319 ) ) ;
#18316=CARTESIAN_POINT ( 'NONE',  ( 44.91013252490152752, 46.79948385550240886, 3.727524721679198461 ) ) ;
#18319=CARTESIAN_POINT ( 'NONE',  ( 43.33558569842706021, 53.90051614449765793, 2.141517661632167169 ) ) ;
#18321=CARTESIAN_POINT ( 'NONE',  ( 55.96859303347804371, 50.19948385550240744, 4.306917132069425946 ) ) ;
#18331=CARTESIAN_POINT ( 'NONE',  ( 47.70284917648453415, 53.39948385550238186, -6.992620115222774047 ) ) ;
#18336=ORIENTED_EDGE ( 'NONE', *, *, #19249, .F. ) ;
#18338=CARTESIAN_POINT ( 'NONE',  ( 45.86712807150329496, 59.70051614449766220, 5.649768623646139964 ) ) ;
#18341=PRODUCT_DEFINITION_CONTEXT ( 'detailed design', #7655, 'design' ) ;
#18345=CARTESIAN_POINT ( 'NONE',  ( 50.02271294988506156, 52.50051614449766646, -6.000000000000000888 ) ) ;
#18351=CARTESIAN_POINT ( 'NONE',  ( 45.31609314410960820, 62.30051614449766362, -6.485486291978072693 ) ) ;
#18367=CARTESIAN_POINT ( 'NONE',  ( 55.69932041026404335, 45.89948385550240317, -1.875703265242203432 ) ) ;
#18369=CARTESIAN_POINT ( 'NONE',  ( 45.31609314410967926, 62.69948385550240744, 6.485486291978119766 ) ) ;
#18370=CARTESIAN_POINT ( 'NONE',  ( 44.03140696652198471, 59.80051614449766362, 4.306917132069485454 ) ) ;
#18378=CARTESIAN_POINT ( 'NONE',  ( 50.02271294988505446, 46.50051614449765935, -7.000000000000000888 ) ) ;
#18379=CARTESIAN_POINT ( 'NONE',  ( 43.33558569842703179, 65.09948385550239891, -2.141517661632099223 ) ) ;
#18385=EDGE_CURVE ( 'NONE', #12707, #11812, #18809, .T. ) ;
#18386=CARTESIAN_POINT ( 'NONE',  ( 44.30067958973596376, 60.89948385550241028, 1.875703265242204099 ) ) ;
#18388=CARTESIAN_POINT ( 'NONE',  ( 56.65037692655918988, 47.89948385550240317, -2.184720259617163762 ) ) ;
#18389=CARTESIAN_POINT ( 'NONE',  ( 58.41169779390614281, 61.00051614449765935, 0.02388180880515032231 ) ) ;
#18390=CARTESIAN_POINT ( 'NONE',  ( 48.02776887271750184, 53.60051614449765367, 5.992620115222795363 ) ) ;
#18406=CARTESIAN_POINT ( 'NONE',  ( 45.86712807150323812, 55.29948385550240175, -5.649768623646098220 ) ) ;
#18410=CARTESIAN_POINT ( 'NONE',  ( 56.81924384183011512, 54.19948385550241454, 4.924951120819313743 ) ) ;
#18414=CARTESIAN_POINT ( 'NONE',  ( 45.86712807150323812, 61.29948385550240886, -5.649768623646098220 ) ) ;
#18418=CARTESIAN_POINT ( 'NONE',  ( 50.02271294988505446, 58.50051614449765935, -7.000000000000000888 ) ) ;
#18420=CARTESIAN_POINT ( 'NONE',  ( 52.29715082351547295, 60.39948385550239607, 6.992620115222774047 ) ) ;
#18427=CARTESIAN_POINT ( 'NONE',  ( 54.13287192849676188, 50.29948385550240175, 5.649768623646098220 ) ) ;
#18436=CARTESIAN_POINT ( 'NONE',  ( 49.97728705011494554, 61.50051614449766646, 6.000000000000000888 ) ) ;
#18442=CARTESIAN_POINT ( 'NONE',  ( 47.42335538002180328, 60.40051614449765793, -8.007379884777206414 ) ) ;
#18462=CARTESIAN_POINT ( 'NONE',  ( 55.96859303347804371, 64.19948385550239323, 4.306917132069425946 ) ) ;
#18464=CARTESIAN_POINT ( 'NONE',  ( 41.58830220609386430, 60.99948385550241170, 0.02388180880523263147 ) ) ;
#18466=CARTESIAN_POINT ( 'NONE',  ( 50.02271294988505446, 58.50051614449765935, -7.000000000000000888 ) ) ;
#18471=VERTEX_POINT ( 'NONE', #11224 ) ;
#18474=CARTESIAN_POINT ( 'NONE',  ( 54.13287192849671214, 46.70051614449766220, -5.649768623646139964 ) ) ;
#18482=CARTESIAN_POINT ( 'NONE',  ( 48.07319477248768180, 62.59948385550238470, 6.007379884777225953 ) ) ;
#18487=CARTESIAN_POINT ( 'NONE',  ( 50.02271294988505446, 60.50051614449766646, -8.000000000000001776 ) ) ;
#18488=CARTESIAN_POINT ( 'NONE',  ( 53.54508667620424234, 60.70051614449766930, -4.840751629271188961 ) ) ;
#18494=ORIENTED_EDGE ( 'NONE', *, *, #12268, .F. ) ;
#18502=CARTESIAN_POINT ( 'NONE',  ( 43.34962307344081012, 50.89948385550241028, 2.184720259617164650 ) ) ;
#18506=CARTESIAN_POINT ( 'NONE',  ( 56.81924384183011512, 52.19948385550240744, 4.924951120819313743 ) ) ;
#18509=CARTESIAN_POINT ( 'NONE',  ( 49.97728705011488159, 61.49948385550240459, -7.000000000000000888 ) ) ;
#18514=CARTESIAN_POINT ( 'NONE',  ( 55.96859303347802239, 58.80051614449764941, -4.306917132069484566 ) ) ;
#18518=CARTESIAN_POINT ( 'NONE',  ( 56.65037692655918988, 55.89948385550240317, -2.184720259617163762 ) ) ;
#18526=CARTESIAN_POINT ( 'NONE',  ( 44.03140696652192787, 49.19948385550240033, -4.306917132069425058 ) ) ;
#18535=CARTESIAN_POINT ( 'NONE',  ( 56.65037692655921120, 63.10051614449766078, 2.184720259617097593 ) ) ;
#18538=CARTESIAN_POINT ( 'NONE',  ( 44.05948171654949874, 46.79948385550238754, 4.345558710429105354 ) ) ;
#18542=CARTESIAN_POINT ( 'NONE',  ( 44.91013252490150620, 60.20051614449766220, -3.727524721679154940 ) ) ;
#18549=CARTESIAN_POINT ( 'NONE',  ( 45.27934281921082516, 59.70051614449766220, 6.458785618021089192 ) ) ;
#18565=CARTESIAN_POINT ( 'NONE',  ( 52.25172492374522903, 63.59948385550237759, -7.007379884777225953 ) ) ;
#18567=CARTESIAN_POINT ( 'NONE',  ( 41.58830220609386430, 56.99948385550241170, 0.02388180880523263147 ) ) ;
#18568=CARTESIAN_POINT ( 'NONE',  ( 57.36023556966787851, 61.00051614449766646, 0.02388180880515038476 ) ) ;
#18578=CARTESIAN_POINT ( 'NONE',  ( 47.74827507625470702, 48.40051614449765793, -7.007379884777204637 ) ) ;
#18584=CARTESIAN_POINT ( 'NONE',  ( 46.49166364869460466, 64.69948385550240744, 4.867452303228209765 ) ) ;
#18586=CARTESIAN_POINT ( 'NONE',  ( 55.94051828345050836, 47.79948385550240886, -4.345558710429104465 ) ) ;
#18587=CARTESIAN_POINT ( 'NONE',  ( 45.27934281921075410, 47.29948385550241596, -6.458785618021043895 ) ) ;
#18589=CARTESIAN_POINT ( 'NONE',  ( 47.37792948025170858, 57.60051614449765367, 7.992620115222797139 ) ) ;
#18590=CARTESIAN_POINT ( 'NONE',  ( 48.02776887271750184, 61.60051614449765367, 5.992620115222795363 ) ) ;
#18601=CARTESIAN_POINT ( 'NONE',  ( 57.36023556966787851, 51.99948385550239749, -0.02388180880522424582 ) ) ;
#18605=CARTESIAN_POINT ( 'NONE',  ( 56.79116909180255135, 53.79948385550241596, -4.963592699179005585 ) ) ;
#18607=CARTESIAN_POINT ( 'NONE',  ( 43.34962307344081012, 62.89948385550241028, 2.184720259617164650 ) ) ;
#18610=CARTESIAN_POINT ( 'NONE',  ( 45.86712807150329496, 57.70051614449765509, 5.649768623646139964 ) ) ;
#18611=CARTESIAN_POINT ( 'NONE',  ( 48.02776887271745210, 63.39948385550238896, -5.992620115222778487 ) ) ;
#18612=CARTESIAN_POINT ( 'NONE',  ( 52.25172492374522903, 57.59948385550241312, -7.007379884777225953 ) ) ;
#18620=CARTESIAN_POINT ( 'NONE',  ( 47.70284917648453415, 49.39948385550238896, -6.992620115222774047 ) ) ;
#18626=CARTESIAN_POINT ( 'NONE',  ( 49.99999999999997158, 45.00000000000003553, -7.000000000000000888 ) ) ;
#18630=CARTESIAN_POINT ( 'NONE',  ( 55.08986747509849380, 59.20051614449766220, 3.727524721679155384 ) ) ;
#18636=CARTESIAN_POINT ( 'NONE',  ( 47.37792948025170858, 59.60051614449765367, 7.992620115222797139 ) ) ;
#18660=CARTESIAN_POINT ( 'NONE',  ( 43.34962307344081012, 62.89948385550241028, 2.184720259617164650 ) ) ;
#18662=CARTESIAN_POINT ( 'NONE',  ( 49.97728705011486738, 57.49948385550241170, -8.000000000000001776 ) ) ;
#18663=CARTESIAN_POINT ( 'NONE',  ( 43.33558569842706021, 63.90051614449765793, 2.141517661632167169 ) ) ;
#18668=CARTESIAN_POINT ( 'NONE',  ( 54.09612160359792199, 53.30051614449766362, 5.676469297603124353 ) ) ;
#18678=CARTESIAN_POINT ( 'NONE',  ( 54.68390685589039890, 57.30051614449767072, 6.485486291978072693 ) ) ;
#18679=CARTESIAN_POINT ( 'NONE',  ( 48.07319477248762496, 60.40051614449765793, -6.007379884777208190 ) ) ;
#18692=CARTESIAN_POINT ( 'NONE',  ( 52.29715082351547295, 56.39948385550239607, 6.992620115222774047 ) ) ;
#18697=CARTESIAN_POINT ( 'NONE',  ( 49.97728705011486738, 53.49948385550240459, -8.000000000000001776 ) ) ;
#18700=CARTESIAN_POINT ( 'NONE',  ( 55.71335778527780747, 46.09948385550240602, 1.832500667257165983 ) ) ;
#18703=CARTESIAN_POINT ( 'NONE',  ( 55.94051828345053679, 61.20051614449766220, 4.345558710429044069 ) ) ;
#18704=CARTESIAN_POINT ( 'NONE',  ( 44.88205777487398507, 63.19948385550240744, -3.688883143319540814 ) ) ;
#18706=CARTESIAN_POINT ( 'NONE',  ( 43.33558569842703179, 59.09948385550240602, -2.141517661632099223 ) ) ;
#18708=CARTESIAN_POINT ( 'NONE',  ( 49.99999999999997158, 65.00000000000002842, -7.000000000000000888 ) ) ;
#18714=CARTESIAN_POINT ( 'NONE',  ( 44.05948171654949874, 56.79948385550240886, 4.345558710429105354 ) ) ;
#18721=CARTESIAN_POINT ( 'NONE',  ( 47.74827507625470702, 64.40051614449765793, -7.007379884777204637 ) ) ;
#18724=CARTESIAN_POINT ( 'NONE',  ( 57.36023556966787851, 47.99948385550239038, -0.02388180880522424582 ) ) ;
#18726=CARTESIAN_POINT ( 'NONE',  ( 56.30877334542961421, 61.00051614449765935, 0.02388180880515774693 ) ) ;
#18746=CARTESIAN_POINT ( 'NONE',  ( 44.28664221472220675, 47.09948385550240602, -1.832500667257165317 ) ) ;
#18747=MECHANICAL_DESIGN_GEOMETRIC_PRESENTATION_REPRESENTATION('',(#15290),#263);
#18749=CARTESIAN_POINT ( 'NONE',  ( 55.96859303347804371, 46.19948385550238612, 4.306917132069425946 ) ) ;
#18750=CARTESIAN_POINT ( 'NONE',  ( 55.96859303347802239, 58.80051614449764941, -4.306917132069484566 ) ) ;
#18763=CARTESIAN_POINT ( 'NONE',  ( 52.25172492374528588, 53.40051614449765083, 7.007379884777204637 ) ) ;
#18773=CARTESIAN_POINT ( 'NONE',  ( 45.90387839640214196, 48.69948385550240744, 5.676469297603166098 ) ) ;
#18776=CARTESIAN_POINT ( 'NONE',  ( 47.42335538002188144, 46.59948385550239891, 8.007379884777233059 ) ) ;
#18777=CARTESIAN_POINT ( 'NONE',  ( 44.91013252490150620, 64.20051614449766930, -3.727524721679154940 ) ) ;
#18780=DIRECTION ( 'NONE',  ( 0.000000000000000000, 1.000000000000000000, 0.000000000000000000 ) ) ;
#18792=CARTESIAN_POINT ( 'NONE',  ( 54.13287192849676188, 56.29948385550240175, 5.649768623646098220 ) ) ;
#18797=CARTESIAN_POINT ( 'NONE',  ( 57.60143344285433642, 51.89948385550241028, -2.493737253992118319 ) ) ;
#18799=CARTESIAN_POINT ( 'NONE',  ( 55.08986747509847248, 51.79948385550240175, -3.727524721679197572 ) ) ;
#18802=CARTESIAN_POINT ( 'NONE',  ( 47.37792948025170858, 45.60051614449765367, 7.992620115222797139 ) ) ;
#18804=CARTESIAN_POINT ( 'NONE',  ( 55.11794222512599362, 44.80051614449766362, -3.688883143319583446 ) ) ;
#18809=CIRCLE ( 'NONE', #12530, 0.4999999999999972244 ) ;
#18815=CARTESIAN_POINT ( 'NONE',  ( 49.97728705011488159, 55.49948385550240459, -7.000000000000000888 ) ) ;
#18827=CARTESIAN_POINT ( 'NONE',  ( 45.86712807150323812, 53.29948385550240886, -5.649768623646098220 ) ) ;
#18830=CARTESIAN_POINT ( 'NONE',  ( 55.08986747509849380, 61.20051614449766220, 3.727524721679155384 ) ) ;
#18854=CARTESIAN_POINT ( 'NONE',  ( 48.07319477248768180, 48.59948385550239891, 6.007379884777225953 ) ) ;
#18856=CARTESIAN_POINT ( 'NONE',  ( 42.63976443033212860, 46.99948385550240459, 0.02388180880522514787 ) ) ;
#18857=CARTESIAN_POINT ( 'NONE',  ( 47.37792948025170858, 45.60051614449765367, 7.992620115222797139 ) ) ;
#18867=CARTESIAN_POINT ( 'NONE',  ( 44.03140696652198471, 49.80051614449765651, 4.306917132069485454 ) ) ;
#18874=CARTESIAN_POINT ( 'NONE',  ( 47.74827507625478518, 52.59948385550239180, 7.007379884777227730 ) ) ;
#18876=CARTESIAN_POINT ( 'NONE',  ( 56.79116909180259398, 63.20051614449766220, 4.963592699178938972 ) ) ;
#18879=CARTESIAN_POINT ( 'NONE',  ( 56.30877334542961421, 63.00051614449766646, 0.02388180880515774693 ) ) ;
#18893=CARTESIAN_POINT ( 'NONE',  ( 43.33558569842703179, 59.09948385550240602, -2.141517661632099223 ) ) ;
#18897=CARTESIAN_POINT ( 'NONE',  ( 57.60143344285433642, 59.89948385550240317, -2.493737253992118319 ) ) ;
#18899=CARTESIAN_POINT ( 'NONE',  ( 44.91013252490152752, 50.79948385550240175, 3.727524721679198461 ) ) ;
#18902=CARTESIAN_POINT ( 'NONE',  ( 49.97728705011495265, 47.50051614449765935, 8.000000000000001776 ) ) ;
#18904=CARTESIAN_POINT ( 'NONE',  ( 51.97223112728254790, 64.39948385550239607, 5.992620115222778487 ) ) ;
#18913=CARTESIAN_POINT ( 'NONE',  ( 56.66441430157296821, 58.09948385550240602, 2.141517661632100111 ) ) ;
#18921=CARTESIAN_POINT ( 'NONE',  ( 47.74827507625478518, 54.59948385550239180, 7.007379884777227730 ) ) ;
#18923=CARTESIAN_POINT ( 'NONE',  ( 52.25172492374527877, 47.40051614449766504, 7.007379884777203749 ) ) ;
#18933=( NAMED_UNIT ( * ) PLANE_ANGLE_UNIT ( ) SI_UNIT ( $, .RADIAN. ) );
#18946=CARTESIAN_POINT ( 'NONE',  ( 55.71335778527780036, 50.90051614449765793, -1.832500667257213056 ) ) ;
#18950=CARTESIAN_POINT ( 'NONE',  ( 55.08986747509847248, 51.79948385550240175, -3.727524721679197572 ) ) ;
#18952=CARTESIAN_POINT ( 'NONE',  ( 52.57664461997811856, 63.59948385550239891, -8.007379884777229506 ) ) ;
#18953=CARTESIAN_POINT ( 'NONE',  ( 56.79116909180259398, 49.20051614449766220, 4.963592699178938972 ) ) ;
#18961=CARTESIAN_POINT ( 'NONE',  ( 44.03140696652198471, 51.80051614449766362, 4.306917132069485454 ) ) ;
#18964=CARTESIAN_POINT ( 'NONE',  ( 55.00886502606627459, 44.74918607449495767, -5.000000000000008882 ) ) ;
#18968=CARTESIAN_POINT ( 'NONE',  ( 45.86712807150323812, 51.29948385550240175, -5.649768623646098220 ) ) ;
#18971=CARTESIAN_POINT ( 'NONE',  ( 50.02271294988505446, 64.50051614449766646, -8.000000000000001776 ) ) ;
#18973=CARTESIAN_POINT ( 'NONE',  ( 43.34962307344078880, 46.10051614449766078, -2.184720259617096705 ) ) ;
#18985=CARTESIAN_POINT ( 'NONE',  ( 55.94051828345050836, 59.79948385550240175, -4.345558710429103577 ) ) ;
#18989=CARTESIAN_POINT ( 'NONE',  ( 42.38452918213188525, 61.09948385550241312, -2.450534656007040013 ) ) ;
#18993=CARTESIAN_POINT ( 'NONE',  ( 53.54508667620428497, 48.29948385550240175, 4.840751629271157874 ) ) ;
#18996=CARTESIAN_POINT ( 'NONE',  ( 42.38452918213190657, 49.90051614449766504, 2.450534656007115508 ) ) ;
#18998=CARTESIAN_POINT ( 'NONE',  ( 44.28664221472221385, 49.90051614449766504, 1.832500667257213722 ) ) ;
#19009=CARTESIAN_POINT ( 'NONE',  ( 56.65037692655918988, 57.89948385550240317, -2.184720259617163762 ) ) ;
#19019=CARTESIAN_POINT ( 'NONE',  ( 54.13287192849676188, 50.29948385550240175, 5.649768623646098220 ) ) ;
#19022=CARTESIAN_POINT ( 'NONE',  ( 50.02271294988505446, 46.50051614449765935, -7.000000000000000888 ) ) ;
#19043=CARTESIAN_POINT ( 'NONE',  ( 49.97728705011494554, 51.50051614449765935, 6.000000000000000888 ) ) ;
#19047=CARTESIAN_POINT ( 'NONE',  ( 49.97728705011488870, 49.49948385550241170, -6.000000000000000888 ) ) ;
#19050=CARTESIAN_POINT ( 'NONE',  ( 55.94051828345050836, 45.79948385550240886, -4.345558710429104465 ) ) ;
#19051=CARTESIAN_POINT ( 'NONE',  ( 52.57664461997821093, 47.40051614449765793, 8.007379884777206414 ) ) ;
#19064=CARTESIAN_POINT ( 'NONE',  ( 57.36023556966787851, 51.00051614449765225, 0.02388180880515038476 ) ) ;
#19070=CARTESIAN_POINT ( 'NONE',  ( 56.66441430157296821, 50.09948385550240602, 2.141517661632100111 ) ) ;
#19072=CARTESIAN_POINT ( 'NONE',  ( 43.20883090819745576, 46.79948385550240886, 4.963592699179006473 ) ) ;
#19074=CARTESIAN_POINT ( 'NONE',  ( 52.29715082351538769, 48.60051614449766788, -6.992620115222796251 ) ) ;
#19091=CARTESIAN_POINT ( 'NONE',  ( 42.38452918213188525, 57.09948385550240602, -2.450534656007040013 ) ) ;
#19093=CARTESIAN_POINT ( 'NONE',  ( 53.54508667620428497, 52.29948385550240886, 4.840751629271157874 ) ) ;
#19097=CARTESIAN_POINT ( 'NONE',  ( 45.27934281921082516, 47.70051614449766220, 6.458785618021089192 ) ) ;
#19098=CARTESIAN_POINT ( 'NONE',  ( 55.11794222512599362, 46.80051614449766362, -3.688883143319583446 ) ) ;
#19109=CARTESIAN_POINT ( 'NONE',  ( 55.94051828345050836, 55.79948385550238044, -4.345558710429104465 ) ) ;
#19119=CARTESIAN_POINT ( 'NONE',  ( 44.03140696652192787, 51.19948385550238612, -4.306917132069425058 ) ) ;
#19122=CARTESIAN_POINT ( 'NONE',  ( 54.09612160359792199, 47.30051614449765651, 5.676469297603124353 ) ) ;
#19145=CARTESIAN_POINT ( 'NONE',  ( 48.02776887271750184, 51.60051614449766788, 5.992620115222795363 ) ) ;
#19149=CARTESIAN_POINT ( 'NONE',  ( 50.02271294988511841, 50.49948385550239749, 6.000000000000000888 ) ) ;
#19153=CARTESIAN_POINT ( 'NONE',  ( 43.34962307344081012, 50.89948385550241028, 2.184720259617164650 ) ) ;
#19155=CARTESIAN_POINT ( 'NONE',  ( 42.39856655714564226, 48.10051614449766078, -2.493737253992044156 ) ) ;
#19175=CARTESIAN_POINT ( 'NONE',  ( 49.97728705011488159, 51.49948385550240459, -7.000000000000000888 ) ) ;
#19177=CARTESIAN_POINT ( 'NONE',  ( 47.37792948025162332, 49.39948385550241028, -7.992620115222770494 ) ) ;
#19180=CARTESIAN_POINT ( 'NONE',  ( 54.09612160359792199, 49.30051614449765651, 5.676469297603124353 ) ) ;
#19193=CARTESIAN_POINT ( 'NONE',  ( 50.02271294988505446, 64.50051614449765225, -7.000000000000000888 ) ) ;
#19195=CARTESIAN_POINT ( 'NONE',  ( 43.18075615816989199, 57.19948385550241454, -4.924951120819313743 ) ) ;
#19199=CARTESIAN_POINT ( 'NONE',  ( 43.69122665457040000, 52.99948385550241170, 0.02388180880521036456 ) ) ;
#19202=CARTESIAN_POINT ( 'NONE',  ( 54.68390685589039890, 45.30051614449766362, 6.485486291978072693 ) ) ;
#19203=CARTESIAN_POINT ( 'NONE',  ( 51.92680522751238925, 51.40051614449767214, 6.007379884777208190 ) ) ;
#19211=CARTESIAN_POINT ( 'NONE',  ( 56.66441430157296821, 62.09948385550239891, 2.141517661632100111 ) ) ;
#19216=CARTESIAN_POINT ( 'NONE',  ( 52.25172492374522903, 47.59948385550240602, -7.007379884777227730 ) ) ;
#19221=CARTESIAN_POINT ( 'NONE',  ( 45.90387839640214196, 54.69948385550240744, 5.676469297603166098 ) ) ;
#19223=CARTESIAN_POINT ( 'NONE',  ( 54.13287192849671214, 48.70051614449766220, -5.649768623646139964 ) ) ;
#19240=CARTESIAN_POINT ( 'NONE',  ( 50.02271294988506156, 48.50051614449765935, -6.000000000000000888 ) ) ;
#19245=CARTESIAN_POINT ( 'NONE',  ( 48.02776887271745210, 55.39948385550240317, -5.992620115222778487 ) ) ;
#19247=CARTESIAN_POINT ( 'NONE',  ( 43.34962307344081012, 54.89948385550240317, 2.184720259617164650 ) ) ;
#19248=CARTESIAN_POINT ( 'NONE',  ( 43.18075615816994173, 49.80051614449765651, 4.924951120819380357 ) ) ;
#19249=EDGE_CURVE ( 'NONE', #18471, #7311, #15315, .T. ) ;
#19270=CARTESIAN_POINT ( 'NONE',  ( 56.65037692655918988, 51.89948385550241028, -2.184720259617163762 ) ) ;
#19272=CARTESIAN_POINT ( 'NONE',  ( 45.27934281921075410, 51.29948385550240175, -6.458785618021043895 ) ) ;
#19274=CARTESIAN_POINT ( 'NONE',  ( 55.94051828345053679, 49.20051614449766930, 4.345558710429044069 ) ) ;
#19290=CARTESIAN_POINT ( 'NONE',  ( 58.41169779390614281, 57.99948385550241170, -0.02388180880523160798 ) ) ;
#19293=CARTESIAN_POINT ( 'NONE',  ( 44.30067958973596376, 58.89948385550241028, 1.875703265242204099 ) ) ;
#19297=CARTESIAN_POINT ( 'NONE',  ( 56.79116909180259398, 53.20051614449766220, 4.963592699178938972 ) ) ;
#19299=CARTESIAN_POINT ( 'NONE',  ( 55.69932041026405045, 47.10051614449766078, 1.875703265242156359 ) ) ;
#19307=CARTESIAN_POINT ( 'NONE',  ( 43.34962307344081012, 62.89948385550241028, 2.184720259617164650 ) ) ;
#19313=CARTESIAN_POINT ( 'NONE',  ( 47.70284917648453415, 47.39948385550239607, -6.992620115222774047 ) ) ;
#19318=CARTESIAN_POINT ( 'NONE',  ( 44.03140696652192787, 55.19948385550238612, -4.306917132069425058 ) ) ;
#19319=( GEOMETRIC_REPRESENTATION_CONTEXT ( 3 ) GLOBAL_UNCERTAINTY_ASSIGNED_CONTEXT ( ( #496 ) ) GLOBAL_UNIT_ASSIGNED_CONTEXT ( ( #5087, #17061, #7831 ) ) REPRESENTATION_CONTEXT ( 'NONE', 'WORKASPACE' ) );
#19321=CARTESIAN_POINT ( 'NONE',  ( 56.65037692655921120, 45.10051614449766078, 2.184720259617097593 ) ) ;
#19331=CARTESIAN_POINT ( 'NONE',  ( 42.63976443033212860, 46.99948385550240459, 0.02388180880522514787 ) ) ;
#19341=CARTESIAN_POINT ( 'NONE',  ( 48.07319477248762496, 50.40051614449766504, -6.007379884777208190 ) ) ;
#19345=CARTESIAN_POINT ( 'NONE',  ( 51.97223112728254790, 56.39948385550241028, 5.992620115222778487 ) ) ;
#19347=CARTESIAN_POINT ( 'NONE',  ( 47.70284917648453415, 55.39948385550238896, -6.992620115222774047 ) ) ;
#19348=CARTESIAN_POINT ( 'NONE',  ( 43.20883090819742023, 56.20051614449766220, -4.963592699178938972 ) ) ;
#19369=CARTESIAN_POINT ( 'NONE',  ( 55.94051828345050836, 55.79948385550238044, -4.345558710429104465 ) ) ;
#19372=CARTESIAN_POINT ( 'NONE',  ( 49.97728705011486738, 55.49948385550241170, -8.000000000000001776 ) ) ;
#19374=CARTESIAN_POINT ( 'NONE',  ( 52.25172492374527877, 47.40051614449766504, 7.007379884777203749 ) ) ;
#19395=CARTESIAN_POINT ( 'NONE',  ( 55.69932041026404335, 57.89948385550241028, -1.875703265242203432 ) ) ;
#19399=CARTESIAN_POINT ( 'NONE',  ( 57.61547081786810764, 54.90051614449765793, -2.450534656007114176 ) ) ;
#19400=CARTESIAN_POINT ( 'NONE',  ( 44.91013252490150620, 46.20051614449766220, -3.727524721679154940 ) ) ;
#19462=COLOUR_RGB('Grey',0.48,0.52,0.57);
#19463=FILL_AREA_STYLE_COLOUR('',#19462);
#19464=FILL_AREA_STYLE('',(#19463));
#19465=SURFACE_STYLE_FILL_AREA(#19464);
#19466=SURFACE_SIDE_STYLE('',(#19465));
#19467=SURFACE_STYLE_USAGE(.BOTH.,#19466);
#19468=PRESENTATION_STYLE_ASSIGNMENT((#19467));
ENDSEC;
END-ISO-10303-21;
